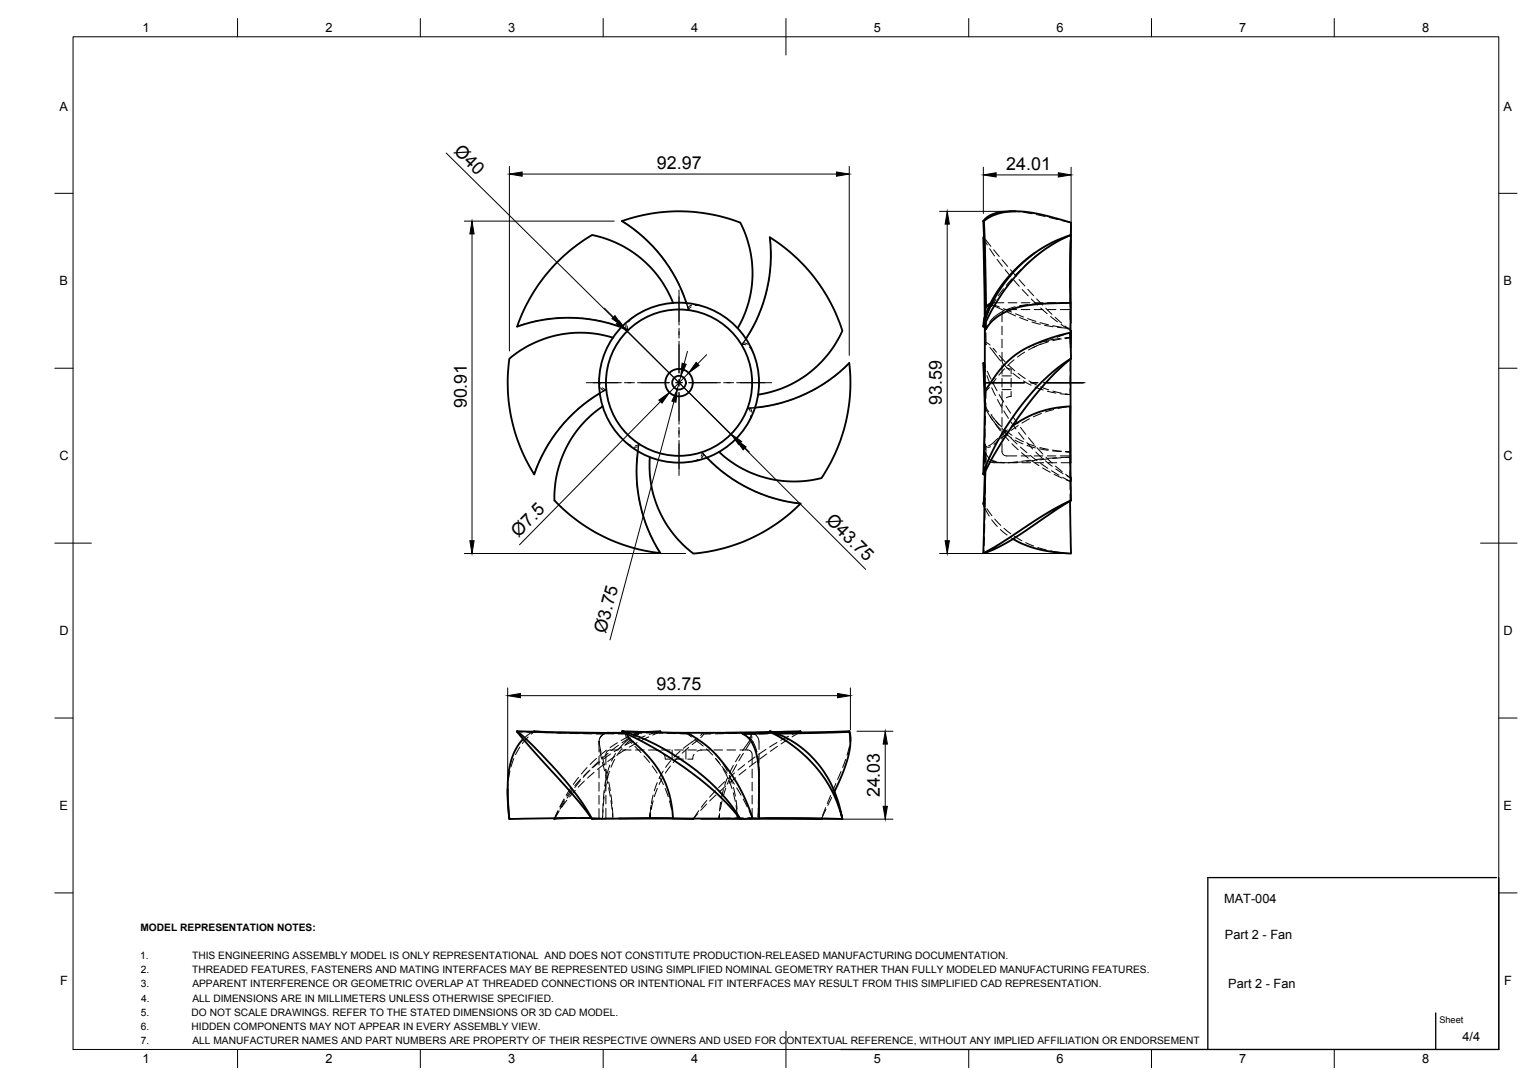
ISO-10303-21;
HEADER;
/* Generated by software containing ST-Developer
 * from STEP Tools, Inc. (www.steptools.com) 
 */

FILE_DESCRIPTION(
/* description */ ('STEP AP214'),
/* implementation_level */ '2;1');

FILE_NAME(
/* name */ 'Part 2 - Fan.step',
/* time_stamp */ '2026-11-14T05:34:33-08:00',
/* author */ (''),
/* organization */ (''),
/* preprocessor_version */ 'ST-DEVELOPER v20.2',
/* originating_system */ 'Autodesk Translation Framework v15.17.0.0',
/* authorisation */ '');

FILE_SCHEMA (('AUTOMOTIVE_DESIGN { 1 0 10303 214 3 1 1 }'));
ENDSEC;

DATA;
#10=MECHANICAL_DESIGN_GEOMETRIC_PRESENTATION_REPRESENTATION('',(#24),#37625);
#20=SHAPE_REPRESENTATION_RELATIONSHIP('SRR','None',#37640,#22);
#22=ADVANCED_BREP_SHAPE_REPRESENTATION('',(#26),#37624);
#24=STYLED_ITEM('',(#37659),#26);
#26=MANIFOLD_SOLID_BREP('Body1',#11498);
#243=B_SPLINE_SURFACE_WITH_KNOTS('',3,3,((#32650,#32651,#32652,#32653,#32654,
#32655,#32656),(#32657,#32658,#32659,#32660,#32661,#32662,#32663),(#32664,
#32665,#32666,#32667,#32668,#32669,#32670),(#32671,#32672,#32673,#32674,
#32675,#32676,#32677),(#32678,#32679,#32680,#32681,#32682,#32683,#32684),
(#32685,#32686,#32687,#32688,#32689,#32690,#32691),(#32692,#32693,#32694,
#32695,#32696,#32697,#32698),(#32699,#32700,#32701,#32702,#32703,#32704,
#32705),(#32706,#32707,#32708,#32709,#32710,#32711,#32712),(#32713,#32714,
#32715,#32716,#32717,#32718,#32719),(#32720,#32721,#32722,#32723,#32724,
#32725,#32726),(#32727,#32728,#32729,#32730,#32731,#32732,#32733),(#32734,
#32735,#32736,#32737,#32738,#32739,#32740)),.UNSPECIFIED.,.F.,.F.,.F.,(4,
3,1,1,1,3,4),(4,3,4),(0.991784279387784,0.992409194183265,0.994306895637448,
0.996204597091632,0.998102298545816,1.,1.0001828629104),(-0.00779503841308724,
0.,0.779503841308724),.UNSPECIFIED.);
#244=B_SPLINE_SURFACE_WITH_KNOTS('',3,3,((#32756,#32757,#32758,#32759,#32760,
#32761,#32762,#32763,#32764,#32765,#32766,#32767,#32768,#32769,#32770,#32771,
#32772),(#32773,#32774,#32775,#32776,#32777,#32778,#32779,#32780,#32781,
#32782,#32783,#32784,#32785,#32786,#32787,#32788,#32789),(#32790,#32791,
#32792,#32793,#32794,#32795,#32796,#32797,#32798,#32799,#32800,#32801,#32802,
#32803,#32804,#32805,#32806),(#32807,#32808,#32809,#32810,#32811,#32812,
#32813,#32814,#32815,#32816,#32817,#32818,#32819,#32820,#32821,#32822,#32823),
(#32824,#32825,#32826,#32827,#32828,#32829,#32830,#32831,#32832,#32833,
#32834,#32835,#32836,#32837,#32838,#32839,#32840),(#32841,#32842,#32843,
#32844,#32845,#32846,#32847,#32848,#32849,#32850,#32851,#32852,#32853,#32854,
#32855,#32856,#32857),(#32858,#32859,#32860,#32861,#32862,#32863,#32864,
#32865,#32866,#32867,#32868,#32869,#32870,#32871,#32872,#32873,#32874),
(#32875,#32876,#32877,#32878,#32879,#32880,#32881,#32882,#32883,#32884,
#32885,#32886,#32887,#32888,#32889,#32890,#32891),(#32892,#32893,#32894,
#32895,#32896,#32897,#32898,#32899,#32900,#32901,#32902,#32903,#32904,#32905,
#32906,#32907,#32908),(#32909,#32910,#32911,#32912,#32913,#32914,#32915,
#32916,#32917,#32918,#32919,#32920,#32921,#32922,#32923,#32924,#32925),
(#32926,#32927,#32928,#32929,#32930,#32931,#32932,#32933,#32934,#32935,
#32936,#32937,#32938,#32939,#32940,#32941,#32942),(#32943,#32944,#32945,
#32946,#32947,#32948,#32949,#32950,#32951,#32952,#32953,#32954,#32955,#32956,
#32957,#32958,#32959),(#32960,#32961,#32962,#32963,#32964,#32965,#32966,
#32967,#32968,#32969,#32970,#32971,#32972,#32973,#32974,#32975,#32976),
(#32977,#32978,#32979,#32980,#32981,#32982,#32983,#32984,#32985,#32986,
#32987,#32988,#32989,#32990,#32991,#32992,#32993),(#32994,#32995,#32996,
#32997,#32998,#32999,#33000,#33001,#33002,#33003,#33004,#33005,#33006,#33007,
#33008,#33009,#33010),(#33011,#33012,#33013,#33014,#33015,#33016,#33017,
#33018,#33019,#33020,#33021,#33022,#33023,#33024,#33025,#33026,#33027)),
 .UNSPECIFIED.,.F.,.F.,.F.,(4,2,1,1,1,1,1,1,1,1,2,4),(4,2,1,1,1,1,1,1,1,
1,1,2,4),(-0.035701835836904,0.,0.090219017653024,0.22554754413256,0.315766561785584,
0.45109508826512,0.541314105918144,0.67664263239768,0.766861650050704,0.90219017653024,
0.992409194183265,1.02810227746674),(-0.0217729438654334,0.,0.0708639855735204,
0.141727971147041,0.212591956720561,0.318887935080842,0.389751920654362,
0.460615906227882,0.566911884588163,0.637775870161683,0.708639855735204,
0.779503841308724,0.801994948010107),.UNSPECIFIED.);
#245=B_SPLINE_SURFACE_WITH_KNOTS('',3,3,((#33062,#33063,#33064,#33065,#33066,
#33067,#33068,#33069,#33070,#33071,#33072,#33073,#33074,#33075,#33076,#33077,
#33078),(#33079,#33080,#33081,#33082,#33083,#33084,#33085,#33086,#33087,
#33088,#33089,#33090,#33091,#33092,#33093,#33094,#33095),(#33096,#33097,
#33098,#33099,#33100,#33101,#33102,#33103,#33104,#33105,#33106,#33107,#33108,
#33109,#33110,#33111,#33112),(#33113,#33114,#33115,#33116,#33117,#33118,
#33119,#33120,#33121,#33122,#33123,#33124,#33125,#33126,#33127,#33128,#33129),
(#33130,#33131,#33132,#33133,#33134,#33135,#33136,#33137,#33138,#33139,
#33140,#33141,#33142,#33143,#33144,#33145,#33146),(#33147,#33148,#33149,
#33150,#33151,#33152,#33153,#33154,#33155,#33156,#33157,#33158,#33159,#33160,
#33161,#33162,#33163),(#33164,#33165,#33166,#33167,#33168,#33169,#33170,
#33171,#33172,#33173,#33174,#33175,#33176,#33177,#33178,#33179,#33180),
(#33181,#33182,#33183,#33184,#33185,#33186,#33187,#33188,#33189,#33190,
#33191,#33192,#33193,#33194,#33195,#33196,#33197),(#33198,#33199,#33200,
#33201,#33202,#33203,#33204,#33205,#33206,#33207,#33208,#33209,#33210,#33211,
#33212,#33213,#33214),(#33215,#33216,#33217,#33218,#33219,#33220,#33221,
#33222,#33223,#33224,#33225,#33226,#33227,#33228,#33229,#33230,#33231),
(#33232,#33233,#33234,#33235,#33236,#33237,#33238,#33239,#33240,#33241,
#33242,#33243,#33244,#33245,#33246,#33247,#33248),(#33249,#33250,#33251,
#33252,#33253,#33254,#33255,#33256,#33257,#33258,#33259,#33260,#33261,#33262,
#33263,#33264,#33265),(#33266,#33267,#33268,#33269,#33270,#33271,#33272,
#33273,#33274,#33275,#33276,#33277,#33278,#33279,#33280,#33281,#33282),
(#33283,#33284,#33285,#33286,#33287,#33288,#33289,#33290,#33291,#33292,
#33293,#33294,#33295,#33296,#33297,#33298,#33299),(#33300,#33301,#33302,
#33303,#33304,#33305,#33306,#33307,#33308,#33309,#33310,#33311,#33312,#33313,
#33314,#33315,#33316),(#33317,#33318,#33319,#33320,#33321,#33322,#33323,
#33324,#33325,#33326,#33327,#33328,#33329,#33330,#33331,#33332,#33333),
(#33334,#33335,#33336,#33337,#33338,#33339,#33340,#33341,#33342,#33343,
#33344,#33345,#33346,#33347,#33348,#33349,#33350)),.UNSPECIFIED.,.F.,.F.,
 .F.,(4,2,1,1,1,1,1,1,1,1,1,2,4),(4,2,1,1,1,1,1,1,1,1,1,2,4),(-0.0353050121574204,
0.,0.0909090909090909,0.181818181818182,0.272727272727273,0.409090909090909,
0.5,0.590909090909091,0.727272727272727,0.818181818181818,0.909090909090909,
1.,1.03479194496591),(-0.021689269548343,0.,0.0708639855735204,0.141727971147041,
0.212591956720561,0.318887935080842,0.389751920654362,0.460615906227882,
0.566911884588163,0.637775870161683,0.708639855735204,0.779503841308724,
0.801875267322681),.UNSPECIFIED.);
#246=B_SPLINE_SURFACE_WITH_KNOTS('',3,3,((#33361,#33362,#33363,#33364,#33365,
#33366,#33367,#33368,#33369,#33370,#33371,#33372,#33373,#33374,#33375,#33376,
#33377),(#33378,#33379,#33380,#33381,#33382,#33383,#33384,#33385,#33386,
#33387,#33388,#33389,#33390,#33391,#33392,#33393,#33394),(#33395,#33396,
#33397,#33398,#33399,#33400,#33401,#33402,#33403,#33404,#33405,#33406,#33407,
#33408,#33409,#33410,#33411),(#33412,#33413,#33414,#33415,#33416,#33417,
#33418,#33419,#33420,#33421,#33422,#33423,#33424,#33425,#33426,#33427,#33428),
(#33429,#33430,#33431,#33432,#33433,#33434,#33435,#33436,#33437,#33438,
#33439,#33440,#33441,#33442,#33443,#33444,#33445),(#33446,#33447,#33448,
#33449,#33450,#33451,#33452,#33453,#33454,#33455,#33456,#33457,#33458,#33459,
#33460,#33461,#33462),(#33463,#33464,#33465,#33466,#33467,#33468,#33469,
#33470,#33471,#33472,#33473,#33474,#33475,#33476,#33477,#33478,#33479),
(#33480,#33481,#33482,#33483,#33484,#33485,#33486,#33487,#33488,#33489,
#33490,#33491,#33492,#33493,#33494,#33495,#33496),(#33497,#33498,#33499,
#33500,#33501,#33502,#33503,#33504,#33505,#33506,#33507,#33508,#33509,#33510,
#33511,#33512,#33513),(#33514,#33515,#33516,#33517,#33518,#33519,#33520,
#33521,#33522,#33523,#33524,#33525,#33526,#33527,#33528,#33529,#33530),
(#33531,#33532,#33533,#33534,#33535,#33536,#33537,#33538,#33539,#33540,
#33541,#33542,#33543,#33544,#33545,#33546,#33547),(#33548,#33549,#33550,
#33551,#33552,#33553,#33554,#33555,#33556,#33557,#33558,#33559,#33560,#33561,
#33562,#33563,#33564),(#33565,#33566,#33567,#33568,#33569,#33570,#33571,
#33572,#33573,#33574,#33575,#33576,#33577,#33578,#33579,#33580,#33581),
(#33582,#33583,#33584,#33585,#33586,#33587,#33588,#33589,#33590,#33591,
#33592,#33593,#33594,#33595,#33596,#33597,#33598),(#33599,#33600,#33601,
#33602,#33603,#33604,#33605,#33606,#33607,#33608,#33609,#33610,#33611,#33612,
#33613,#33614,#33615),(#33616,#33617,#33618,#33619,#33620,#33621,#33622,
#33623,#33624,#33625,#33626,#33627,#33628,#33629,#33630,#33631,#33632),
(#33633,#33634,#33635,#33636,#33637,#33638,#33639,#33640,#33641,#33642,
#33643,#33644,#33645,#33646,#33647,#33648,#33649)),.UNSPECIFIED.,.F.,.F.,
 .F.,(4,2,1,1,1,1,1,1,1,1,1,2,4),(4,2,1,1,1,1,1,1,1,1,1,2,4),(-0.0353050121574204,
0.,0.0909090909090909,0.181818181818182,0.272727272727273,0.409090909090909,
0.5,0.590909090909091,0.727272727272727,0.818181818181818,0.909090909090909,
1.,1.03479194496591),(-0.021689269548343,0.,0.0708639855735204,0.141727971147041,
0.212591956720561,0.318887935080842,0.389751920654362,0.460615906227882,
0.566911884588163,0.637775870161683,0.708639855735204,0.779503841308724,
0.801875267322681),.UNSPECIFIED.);
#247=B_SPLINE_SURFACE_WITH_KNOTS('',3,3,((#33693,#33694,#33695,#33696,#33697,
#33698,#33699,#33700,#33701,#33702,#33703,#33704,#33705,#33706,#33707,#33708,
#33709),(#33710,#33711,#33712,#33713,#33714,#33715,#33716,#33717,#33718,
#33719,#33720,#33721,#33722,#33723,#33724,#33725,#33726),(#33727,#33728,
#33729,#33730,#33731,#33732,#33733,#33734,#33735,#33736,#33737,#33738,#33739,
#33740,#33741,#33742,#33743),(#33744,#33745,#33746,#33747,#33748,#33749,
#33750,#33751,#33752,#33753,#33754,#33755,#33756,#33757,#33758,#33759,#33760),
(#33761,#33762,#33763,#33764,#33765,#33766,#33767,#33768,#33769,#33770,
#33771,#33772,#33773,#33774,#33775,#33776,#33777),(#33778,#33779,#33780,
#33781,#33782,#33783,#33784,#33785,#33786,#33787,#33788,#33789,#33790,#33791,
#33792,#33793,#33794),(#33795,#33796,#33797,#33798,#33799,#33800,#33801,
#33802,#33803,#33804,#33805,#33806,#33807,#33808,#33809,#33810,#33811),
(#33812,#33813,#33814,#33815,#33816,#33817,#33818,#33819,#33820,#33821,
#33822,#33823,#33824,#33825,#33826,#33827,#33828),(#33829,#33830,#33831,
#33832,#33833,#33834,#33835,#33836,#33837,#33838,#33839,#33840,#33841,#33842,
#33843,#33844,#33845),(#33846,#33847,#33848,#33849,#33850,#33851,#33852,
#33853,#33854,#33855,#33856,#33857,#33858,#33859,#33860,#33861,#33862),
(#33863,#33864,#33865,#33866,#33867,#33868,#33869,#33870,#33871,#33872,
#33873,#33874,#33875,#33876,#33877,#33878,#33879),(#33880,#33881,#33882,
#33883,#33884,#33885,#33886,#33887,#33888,#33889,#33890,#33891,#33892,#33893,
#33894,#33895,#33896),(#33897,#33898,#33899,#33900,#33901,#33902,#33903,
#33904,#33905,#33906,#33907,#33908,#33909,#33910,#33911,#33912,#33913),
(#33914,#33915,#33916,#33917,#33918,#33919,#33920,#33921,#33922,#33923,
#33924,#33925,#33926,#33927,#33928,#33929,#33930),(#33931,#33932,#33933,
#33934,#33935,#33936,#33937,#33938,#33939,#33940,#33941,#33942,#33943,#33944,
#33945,#33946,#33947),(#33948,#33949,#33950,#33951,#33952,#33953,#33954,
#33955,#33956,#33957,#33958,#33959,#33960,#33961,#33962,#33963,#33964)),
 .UNSPECIFIED.,.F.,.F.,.F.,(4,2,1,1,1,1,1,1,1,1,2,4),(4,2,1,1,1,1,1,1,1,
1,1,2,4),(-0.035701835836904,0.,0.090219017653024,0.22554754413256,0.315766561785584,
0.45109508826512,0.541314105918144,0.67664263239768,0.766861650050704,0.90219017653024,
0.992409194183265,1.02810227746674),(-0.0217729438654334,0.,0.0708639855735204,
0.141727971147041,0.212591956720561,0.318887935080842,0.389751920654362,
0.460615906227882,0.566911884588163,0.637775870161683,0.708639855735204,
0.779503841308724,0.801994948010107),.UNSPECIFIED.);
#248=B_SPLINE_SURFACE_WITH_KNOTS('',3,3,((#33980,#33981,#33982,#33983,#33984,
#33985,#33986),(#33987,#33988,#33989,#33990,#33991,#33992,#33993),(#33994,
#33995,#33996,#33997,#33998,#33999,#34000),(#34001,#34002,#34003,#34004,
#34005,#34006,#34007),(#34008,#34009,#34010,#34011,#34012,#34013,#34014),
(#34015,#34016,#34017,#34018,#34019,#34020,#34021),(#34022,#34023,#34024,
#34025,#34026,#34027,#34028),(#34029,#34030,#34031,#34032,#34033,#34034,
#34035),(#34036,#34037,#34038,#34039,#34040,#34041,#34042),(#34043,#34044,
#34045,#34046,#34047,#34048,#34049),(#34050,#34051,#34052,#34053,#34054,
#34055,#34056),(#34057,#34058,#34059,#34060,#34061,#34062,#34063),(#34064,
#34065,#34066,#34067,#34068,#34069,#34070)),.UNSPECIFIED.,.F.,.F.,.F.,(4,
3,1,1,1,3,4),(4,3,4),(0.991784279387784,0.992409194183265,0.994306895637448,
0.996204597091632,0.998102298545816,1.,1.0001828629104),(-0.00779503841308724,
0.,0.779503841308724),.UNSPECIFIED.);
#249=B_SPLINE_SURFACE_WITH_KNOTS('',3,3,((#34072,#34073,#34074,#34075,#34076,
#34077,#34078,#34079,#34080,#34081,#34082,#34083,#34084,#34085,#34086,#34087,
#34088),(#34089,#34090,#34091,#34092,#34093,#34094,#34095,#34096,#34097,
#34098,#34099,#34100,#34101,#34102,#34103,#34104,#34105),(#34106,#34107,
#34108,#34109,#34110,#34111,#34112,#34113,#34114,#34115,#34116,#34117,#34118,
#34119,#34120,#34121,#34122),(#34123,#34124,#34125,#34126,#34127,#34128,
#34129,#34130,#34131,#34132,#34133,#34134,#34135,#34136,#34137,#34138,#34139),
(#34140,#34141,#34142,#34143,#34144,#34145,#34146,#34147,#34148,#34149,
#34150,#34151,#34152,#34153,#34154,#34155,#34156),(#34157,#34158,#34159,
#34160,#34161,#34162,#34163,#34164,#34165,#34166,#34167,#34168,#34169,#34170,
#34171,#34172,#34173),(#34174,#34175,#34176,#34177,#34178,#34179,#34180,
#34181,#34182,#34183,#34184,#34185,#34186,#34187,#34188,#34189,#34190),
(#34191,#34192,#34193,#34194,#34195,#34196,#34197,#34198,#34199,#34200,
#34201,#34202,#34203,#34204,#34205,#34206,#34207),(#34208,#34209,#34210,
#34211,#34212,#34213,#34214,#34215,#34216,#34217,#34218,#34219,#34220,#34221,
#34222,#34223,#34224),(#34225,#34226,#34227,#34228,#34229,#34230,#34231,
#34232,#34233,#34234,#34235,#34236,#34237,#34238,#34239,#34240,#34241),
(#34242,#34243,#34244,#34245,#34246,#34247,#34248,#34249,#34250,#34251,
#34252,#34253,#34254,#34255,#34256,#34257,#34258),(#34259,#34260,#34261,
#34262,#34263,#34264,#34265,#34266,#34267,#34268,#34269,#34270,#34271,#34272,
#34273,#34274,#34275),(#34276,#34277,#34278,#34279,#34280,#34281,#34282,
#34283,#34284,#34285,#34286,#34287,#34288,#34289,#34290,#34291,#34292),
(#34293,#34294,#34295,#34296,#34297,#34298,#34299,#34300,#34301,#34302,
#34303,#34304,#34305,#34306,#34307,#34308,#34309),(#34310,#34311,#34312,
#34313,#34314,#34315,#34316,#34317,#34318,#34319,#34320,#34321,#34322,#34323,
#34324,#34325,#34326),(#34327,#34328,#34329,#34330,#34331,#34332,#34333,
#34334,#34335,#34336,#34337,#34338,#34339,#34340,#34341,#34342,#34343),
(#34344,#34345,#34346,#34347,#34348,#34349,#34350,#34351,#34352,#34353,
#34354,#34355,#34356,#34357,#34358,#34359,#34360)),.UNSPECIFIED.,.F.,.F.,
 .F.,(4,2,1,1,1,1,1,1,1,1,1,2,4),(4,2,1,1,1,1,1,1,1,1,1,2,4),(-0.0353050121574204,
0.,0.0909090909090909,0.181818181818182,0.272727272727273,0.409090909090909,
0.5,0.590909090909091,0.727272727272727,0.818181818181818,0.909090909090909,
1.,1.03479194496591),(-0.021689269548343,0.,0.0708639855735204,0.141727971147041,
0.212591956720561,0.318887935080842,0.389751920654362,0.460615906227882,
0.566911884588163,0.637775870161683,0.708639855735204,0.779503841308724,
0.801875267322681),.UNSPECIFIED.);
#250=B_SPLINE_SURFACE_WITH_KNOTS('',3,3,((#34404,#34405,#34406,#34407,#34408,
#34409,#34410,#34411,#34412,#34413,#34414,#34415,#34416,#34417,#34418,#34419,
#34420),(#34421,#34422,#34423,#34424,#34425,#34426,#34427,#34428,#34429,
#34430,#34431,#34432,#34433,#34434,#34435,#34436,#34437),(#34438,#34439,
#34440,#34441,#34442,#34443,#34444,#34445,#34446,#34447,#34448,#34449,#34450,
#34451,#34452,#34453,#34454),(#34455,#34456,#34457,#34458,#34459,#34460,
#34461,#34462,#34463,#34464,#34465,#34466,#34467,#34468,#34469,#34470,#34471),
(#34472,#34473,#34474,#34475,#34476,#34477,#34478,#34479,#34480,#34481,
#34482,#34483,#34484,#34485,#34486,#34487,#34488),(#34489,#34490,#34491,
#34492,#34493,#34494,#34495,#34496,#34497,#34498,#34499,#34500,#34501,#34502,
#34503,#34504,#34505),(#34506,#34507,#34508,#34509,#34510,#34511,#34512,
#34513,#34514,#34515,#34516,#34517,#34518,#34519,#34520,#34521,#34522),
(#34523,#34524,#34525,#34526,#34527,#34528,#34529,#34530,#34531,#34532,
#34533,#34534,#34535,#34536,#34537,#34538,#34539),(#34540,#34541,#34542,
#34543,#34544,#34545,#34546,#34547,#34548,#34549,#34550,#34551,#34552,#34553,
#34554,#34555,#34556),(#34557,#34558,#34559,#34560,#34561,#34562,#34563,
#34564,#34565,#34566,#34567,#34568,#34569,#34570,#34571,#34572,#34573),
(#34574,#34575,#34576,#34577,#34578,#34579,#34580,#34581,#34582,#34583,
#34584,#34585,#34586,#34587,#34588,#34589,#34590),(#34591,#34592,#34593,
#34594,#34595,#34596,#34597,#34598,#34599,#34600,#34601,#34602,#34603,#34604,
#34605,#34606,#34607),(#34608,#34609,#34610,#34611,#34612,#34613,#34614,
#34615,#34616,#34617,#34618,#34619,#34620,#34621,#34622,#34623,#34624),
(#34625,#34626,#34627,#34628,#34629,#34630,#34631,#34632,#34633,#34634,
#34635,#34636,#34637,#34638,#34639,#34640,#34641),(#34642,#34643,#34644,
#34645,#34646,#34647,#34648,#34649,#34650,#34651,#34652,#34653,#34654,#34655,
#34656,#34657,#34658),(#34659,#34660,#34661,#34662,#34663,#34664,#34665,
#34666,#34667,#34668,#34669,#34670,#34671,#34672,#34673,#34674,#34675)),
 .UNSPECIFIED.,.F.,.F.,.F.,(4,2,1,1,1,1,1,1,1,1,2,4),(4,2,1,1,1,1,1,1,1,
1,1,2,4),(-0.035701835836904,0.,0.090219017653024,0.22554754413256,0.315766561785584,
0.45109508826512,0.541314105918144,0.67664263239768,0.766861650050704,0.90219017653024,
0.992409194183265,1.02810227746674),(-0.0217729438654334,0.,0.0708639855735204,
0.141727971147041,0.212591956720561,0.318887935080842,0.389751920654362,
0.460615906227882,0.566911884588163,0.637775870161683,0.708639855735204,
0.779503841308724,0.801994948010107),.UNSPECIFIED.);
#251=B_SPLINE_SURFACE_WITH_KNOTS('',3,3,((#34691,#34692,#34693,#34694,#34695,
#34696,#34697),(#34698,#34699,#34700,#34701,#34702,#34703,#34704),(#34705,
#34706,#34707,#34708,#34709,#34710,#34711),(#34712,#34713,#34714,#34715,
#34716,#34717,#34718),(#34719,#34720,#34721,#34722,#34723,#34724,#34725),
(#34726,#34727,#34728,#34729,#34730,#34731,#34732),(#34733,#34734,#34735,
#34736,#34737,#34738,#34739),(#34740,#34741,#34742,#34743,#34744,#34745,
#34746),(#34747,#34748,#34749,#34750,#34751,#34752,#34753),(#34754,#34755,
#34756,#34757,#34758,#34759,#34760),(#34761,#34762,#34763,#34764,#34765,
#34766,#34767),(#34768,#34769,#34770,#34771,#34772,#34773,#34774),(#34775,
#34776,#34777,#34778,#34779,#34780,#34781)),.UNSPECIFIED.,.F.,.F.,.F.,(4,
3,1,1,1,3,4),(4,3,4),(0.991784279387784,0.992409194183265,0.994306895637448,
0.996204597091632,0.998102298545816,1.,1.0001828629104),(-0.00779503841308724,
0.,0.779503841308724),.UNSPECIFIED.);
#252=B_SPLINE_SURFACE_WITH_KNOTS('',3,3,((#34783,#34784,#34785,#34786,#34787,
#34788,#34789,#34790,#34791,#34792,#34793,#34794,#34795,#34796,#34797,#34798,
#34799),(#34800,#34801,#34802,#34803,#34804,#34805,#34806,#34807,#34808,
#34809,#34810,#34811,#34812,#34813,#34814,#34815,#34816),(#34817,#34818,
#34819,#34820,#34821,#34822,#34823,#34824,#34825,#34826,#34827,#34828,#34829,
#34830,#34831,#34832,#34833),(#34834,#34835,#34836,#34837,#34838,#34839,
#34840,#34841,#34842,#34843,#34844,#34845,#34846,#34847,#34848,#34849,#34850),
(#34851,#34852,#34853,#34854,#34855,#34856,#34857,#34858,#34859,#34860,
#34861,#34862,#34863,#34864,#34865,#34866,#34867),(#34868,#34869,#34870,
#34871,#34872,#34873,#34874,#34875,#34876,#34877,#34878,#34879,#34880,#34881,
#34882,#34883,#34884),(#34885,#34886,#34887,#34888,#34889,#34890,#34891,
#34892,#34893,#34894,#34895,#34896,#34897,#34898,#34899,#34900,#34901),
(#34902,#34903,#34904,#34905,#34906,#34907,#34908,#34909,#34910,#34911,
#34912,#34913,#34914,#34915,#34916,#34917,#34918),(#34919,#34920,#34921,
#34922,#34923,#34924,#34925,#34926,#34927,#34928,#34929,#34930,#34931,#34932,
#34933,#34934,#34935),(#34936,#34937,#34938,#34939,#34940,#34941,#34942,
#34943,#34944,#34945,#34946,#34947,#34948,#34949,#34950,#34951,#34952),
(#34953,#34954,#34955,#34956,#34957,#34958,#34959,#34960,#34961,#34962,
#34963,#34964,#34965,#34966,#34967,#34968,#34969),(#34970,#34971,#34972,
#34973,#34974,#34975,#34976,#34977,#34978,#34979,#34980,#34981,#34982,#34983,
#34984,#34985,#34986),(#34987,#34988,#34989,#34990,#34991,#34992,#34993,
#34994,#34995,#34996,#34997,#34998,#34999,#35000,#35001,#35002,#35003),
(#35004,#35005,#35006,#35007,#35008,#35009,#35010,#35011,#35012,#35013,
#35014,#35015,#35016,#35017,#35018,#35019,#35020),(#35021,#35022,#35023,
#35024,#35025,#35026,#35027,#35028,#35029,#35030,#35031,#35032,#35033,#35034,
#35035,#35036,#35037),(#35038,#35039,#35040,#35041,#35042,#35043,#35044,
#35045,#35046,#35047,#35048,#35049,#35050,#35051,#35052,#35053,#35054),
(#35055,#35056,#35057,#35058,#35059,#35060,#35061,#35062,#35063,#35064,
#35065,#35066,#35067,#35068,#35069,#35070,#35071)),.UNSPECIFIED.,.F.,.F.,
 .F.,(4,2,1,1,1,1,1,1,1,1,1,2,4),(4,2,1,1,1,1,1,1,1,1,1,2,4),(-0.0353050121574204,
0.,0.0909090909090909,0.181818181818182,0.272727272727273,0.409090909090909,
0.5,0.590909090909091,0.727272727272727,0.818181818181818,0.909090909090909,
1.,1.03479194496591),(-0.021689269548343,0.,0.0708639855735204,0.141727971147041,
0.212591956720561,0.318887935080842,0.389751920654362,0.460615906227882,
0.566911884588163,0.637775870161683,0.708639855735204,0.779503841308724,
0.801875267322681),.UNSPECIFIED.);
#253=B_SPLINE_SURFACE_WITH_KNOTS('',3,3,((#35115,#35116,#35117,#35118,#35119,
#35120,#35121,#35122,#35123,#35124,#35125,#35126,#35127,#35128,#35129,#35130,
#35131),(#35132,#35133,#35134,#35135,#35136,#35137,#35138,#35139,#35140,
#35141,#35142,#35143,#35144,#35145,#35146,#35147,#35148),(#35149,#35150,
#35151,#35152,#35153,#35154,#35155,#35156,#35157,#35158,#35159,#35160,#35161,
#35162,#35163,#35164,#35165),(#35166,#35167,#35168,#35169,#35170,#35171,
#35172,#35173,#35174,#35175,#35176,#35177,#35178,#35179,#35180,#35181,#35182),
(#35183,#35184,#35185,#35186,#35187,#35188,#35189,#35190,#35191,#35192,
#35193,#35194,#35195,#35196,#35197,#35198,#35199),(#35200,#35201,#35202,
#35203,#35204,#35205,#35206,#35207,#35208,#35209,#35210,#35211,#35212,#35213,
#35214,#35215,#35216),(#35217,#35218,#35219,#35220,#35221,#35222,#35223,
#35224,#35225,#35226,#35227,#35228,#35229,#35230,#35231,#35232,#35233),
(#35234,#35235,#35236,#35237,#35238,#35239,#35240,#35241,#35242,#35243,
#35244,#35245,#35246,#35247,#35248,#35249,#35250),(#35251,#35252,#35253,
#35254,#35255,#35256,#35257,#35258,#35259,#35260,#35261,#35262,#35263,#35264,
#35265,#35266,#35267),(#35268,#35269,#35270,#35271,#35272,#35273,#35274,
#35275,#35276,#35277,#35278,#35279,#35280,#35281,#35282,#35283,#35284),
(#35285,#35286,#35287,#35288,#35289,#35290,#35291,#35292,#35293,#35294,
#35295,#35296,#35297,#35298,#35299,#35300,#35301),(#35302,#35303,#35304,
#35305,#35306,#35307,#35308,#35309,#35310,#35311,#35312,#35313,#35314,#35315,
#35316,#35317,#35318),(#35319,#35320,#35321,#35322,#35323,#35324,#35325,
#35326,#35327,#35328,#35329,#35330,#35331,#35332,#35333,#35334,#35335),
(#35336,#35337,#35338,#35339,#35340,#35341,#35342,#35343,#35344,#35345,
#35346,#35347,#35348,#35349,#35350,#35351,#35352),(#35353,#35354,#35355,
#35356,#35357,#35358,#35359,#35360,#35361,#35362,#35363,#35364,#35365,#35366,
#35367,#35368,#35369),(#35370,#35371,#35372,#35373,#35374,#35375,#35376,
#35377,#35378,#35379,#35380,#35381,#35382,#35383,#35384,#35385,#35386)),
 .UNSPECIFIED.,.F.,.F.,.F.,(4,2,1,1,1,1,1,1,1,1,2,4),(4,2,1,1,1,1,1,1,1,
1,1,2,4),(-0.035701835836904,0.,0.090219017653024,0.22554754413256,0.315766561785584,
0.45109508826512,0.541314105918144,0.67664263239768,0.766861650050704,0.90219017653024,
0.992409194183265,1.02810227746674),(-0.0217729438654334,0.,0.0708639855735204,
0.141727971147041,0.212591956720561,0.318887935080842,0.389751920654362,
0.460615906227882,0.566911884588163,0.637775870161683,0.708639855735204,
0.779503841308724,0.801994948010107),.UNSPECIFIED.);
#254=B_SPLINE_SURFACE_WITH_KNOTS('',3,3,((#35402,#35403,#35404,#35405,#35406,
#35407,#35408),(#35409,#35410,#35411,#35412,#35413,#35414,#35415),(#35416,
#35417,#35418,#35419,#35420,#35421,#35422),(#35423,#35424,#35425,#35426,
#35427,#35428,#35429),(#35430,#35431,#35432,#35433,#35434,#35435,#35436),
(#35437,#35438,#35439,#35440,#35441,#35442,#35443),(#35444,#35445,#35446,
#35447,#35448,#35449,#35450),(#35451,#35452,#35453,#35454,#35455,#35456,
#35457),(#35458,#35459,#35460,#35461,#35462,#35463,#35464),(#35465,#35466,
#35467,#35468,#35469,#35470,#35471),(#35472,#35473,#35474,#35475,#35476,
#35477,#35478),(#35479,#35480,#35481,#35482,#35483,#35484,#35485),(#35486,
#35487,#35488,#35489,#35490,#35491,#35492)),.UNSPECIFIED.,.F.,.F.,.F.,(4,
3,1,1,1,3,4),(4,3,4),(0.991784279387784,0.992409194183265,0.994306895637448,
0.996204597091632,0.998102298545816,1.,1.0001828629104),(-0.00779503841308724,
0.,0.779503841308724),.UNSPECIFIED.);
#255=B_SPLINE_SURFACE_WITH_KNOTS('',3,3,((#35494,#35495,#35496,#35497,#35498,
#35499,#35500,#35501,#35502,#35503,#35504,#35505,#35506,#35507,#35508,#35509,
#35510),(#35511,#35512,#35513,#35514,#35515,#35516,#35517,#35518,#35519,
#35520,#35521,#35522,#35523,#35524,#35525,#35526,#35527),(#35528,#35529,
#35530,#35531,#35532,#35533,#35534,#35535,#35536,#35537,#35538,#35539,#35540,
#35541,#35542,#35543,#35544),(#35545,#35546,#35547,#35548,#35549,#35550,
#35551,#35552,#35553,#35554,#35555,#35556,#35557,#35558,#35559,#35560,#35561),
(#35562,#35563,#35564,#35565,#35566,#35567,#35568,#35569,#35570,#35571,
#35572,#35573,#35574,#35575,#35576,#35577,#35578),(#35579,#35580,#35581,
#35582,#35583,#35584,#35585,#35586,#35587,#35588,#35589,#35590,#35591,#35592,
#35593,#35594,#35595),(#35596,#35597,#35598,#35599,#35600,#35601,#35602,
#35603,#35604,#35605,#35606,#35607,#35608,#35609,#35610,#35611,#35612),
(#35613,#35614,#35615,#35616,#35617,#35618,#35619,#35620,#35621,#35622,
#35623,#35624,#35625,#35626,#35627,#35628,#35629),(#35630,#35631,#35632,
#35633,#35634,#35635,#35636,#35637,#35638,#35639,#35640,#35641,#35642,#35643,
#35644,#35645,#35646),(#35647,#35648,#35649,#35650,#35651,#35652,#35653,
#35654,#35655,#35656,#35657,#35658,#35659,#35660,#35661,#35662,#35663),
(#35664,#35665,#35666,#35667,#35668,#35669,#35670,#35671,#35672,#35673,
#35674,#35675,#35676,#35677,#35678,#35679,#35680),(#35681,#35682,#35683,
#35684,#35685,#35686,#35687,#35688,#35689,#35690,#35691,#35692,#35693,#35694,
#35695,#35696,#35697),(#35698,#35699,#35700,#35701,#35702,#35703,#35704,
#35705,#35706,#35707,#35708,#35709,#35710,#35711,#35712,#35713,#35714),
(#35715,#35716,#35717,#35718,#35719,#35720,#35721,#35722,#35723,#35724,
#35725,#35726,#35727,#35728,#35729,#35730,#35731),(#35732,#35733,#35734,
#35735,#35736,#35737,#35738,#35739,#35740,#35741,#35742,#35743,#35744,#35745,
#35746,#35747,#35748),(#35749,#35750,#35751,#35752,#35753,#35754,#35755,
#35756,#35757,#35758,#35759,#35760,#35761,#35762,#35763,#35764,#35765),
(#35766,#35767,#35768,#35769,#35770,#35771,#35772,#35773,#35774,#35775,
#35776,#35777,#35778,#35779,#35780,#35781,#35782)),.UNSPECIFIED.,.F.,.F.,
 .F.,(4,2,1,1,1,1,1,1,1,1,1,2,4),(4,2,1,1,1,1,1,1,1,1,1,2,4),(-0.0353050121574204,
0.,0.0909090909090909,0.181818181818182,0.272727272727273,0.409090909090909,
0.5,0.590909090909091,0.727272727272727,0.818181818181818,0.909090909090909,
1.,1.03479194496591),(-0.021689269548343,0.,0.0708639855735204,0.141727971147041,
0.212591956720561,0.318887935080842,0.389751920654362,0.460615906227882,
0.566911884588163,0.637775870161683,0.708639855735204,0.779503841308724,
0.801875267322681),.UNSPECIFIED.);
#256=B_SPLINE_SURFACE_WITH_KNOTS('',3,3,((#35814,#35815,#35816,#35817,#35818,
#35819,#35820,#35821,#35822,#35823,#35824,#35825,#35826,#35827,#35828,#35829,
#35830),(#35831,#35832,#35833,#35834,#35835,#35836,#35837,#35838,#35839,
#35840,#35841,#35842,#35843,#35844,#35845,#35846,#35847),(#35848,#35849,
#35850,#35851,#35852,#35853,#35854,#35855,#35856,#35857,#35858,#35859,#35860,
#35861,#35862,#35863,#35864),(#35865,#35866,#35867,#35868,#35869,#35870,
#35871,#35872,#35873,#35874,#35875,#35876,#35877,#35878,#35879,#35880,#35881),
(#35882,#35883,#35884,#35885,#35886,#35887,#35888,#35889,#35890,#35891,
#35892,#35893,#35894,#35895,#35896,#35897,#35898),(#35899,#35900,#35901,
#35902,#35903,#35904,#35905,#35906,#35907,#35908,#35909,#35910,#35911,#35912,
#35913,#35914,#35915),(#35916,#35917,#35918,#35919,#35920,#35921,#35922,
#35923,#35924,#35925,#35926,#35927,#35928,#35929,#35930,#35931,#35932),
(#35933,#35934,#35935,#35936,#35937,#35938,#35939,#35940,#35941,#35942,
#35943,#35944,#35945,#35946,#35947,#35948,#35949),(#35950,#35951,#35952,
#35953,#35954,#35955,#35956,#35957,#35958,#35959,#35960,#35961,#35962,#35963,
#35964,#35965,#35966),(#35967,#35968,#35969,#35970,#35971,#35972,#35973,
#35974,#35975,#35976,#35977,#35978,#35979,#35980,#35981,#35982,#35983),
(#35984,#35985,#35986,#35987,#35988,#35989,#35990,#35991,#35992,#35993,
#35994,#35995,#35996,#35997,#35998,#35999,#36000),(#36001,#36002,#36003,
#36004,#36005,#36006,#36007,#36008,#36009,#36010,#36011,#36012,#36013,#36014,
#36015,#36016,#36017),(#36018,#36019,#36020,#36021,#36022,#36023,#36024,
#36025,#36026,#36027,#36028,#36029,#36030,#36031,#36032,#36033,#36034),
(#36035,#36036,#36037,#36038,#36039,#36040,#36041,#36042,#36043,#36044,
#36045,#36046,#36047,#36048,#36049,#36050,#36051),(#36052,#36053,#36054,
#36055,#36056,#36057,#36058,#36059,#36060,#36061,#36062,#36063,#36064,#36065,
#36066,#36067,#36068),(#36069,#36070,#36071,#36072,#36073,#36074,#36075,
#36076,#36077,#36078,#36079,#36080,#36081,#36082,#36083,#36084,#36085)),
 .UNSPECIFIED.,.F.,.F.,.F.,(4,2,1,1,1,1,1,1,1,1,2,4),(4,2,1,1,1,1,1,1,1,
1,1,2,4),(-0.035701835836904,0.,0.090219017653024,0.22554754413256,0.315766561785584,
0.45109508826512,0.541314105918144,0.67664263239768,0.766861650050704,0.90219017653024,
0.992409194183265,1.02810227746674),(-0.0217729438654334,0.,0.0708639855735204,
0.141727971147041,0.212591956720561,0.318887935080842,0.389751920654362,
0.460615906227882,0.566911884588163,0.637775870161683,0.708639855735204,
0.779503841308724,0.801994948010107),.UNSPECIFIED.);
#257=B_SPLINE_SURFACE_WITH_KNOTS('',3,3,((#36092,#36093,#36094,#36095,#36096,
#36097,#36098),(#36099,#36100,#36101,#36102,#36103,#36104,#36105),(#36106,
#36107,#36108,#36109,#36110,#36111,#36112),(#36113,#36114,#36115,#36116,
#36117,#36118,#36119),(#36120,#36121,#36122,#36123,#36124,#36125,#36126),
(#36127,#36128,#36129,#36130,#36131,#36132,#36133),(#36134,#36135,#36136,
#36137,#36138,#36139,#36140),(#36141,#36142,#36143,#36144,#36145,#36146,
#36147),(#36148,#36149,#36150,#36151,#36152,#36153,#36154),(#36155,#36156,
#36157,#36158,#36159,#36160,#36161),(#36162,#36163,#36164,#36165,#36166,
#36167,#36168),(#36169,#36170,#36171,#36172,#36173,#36174,#36175),(#36176,
#36177,#36178,#36179,#36180,#36181,#36182)),.UNSPECIFIED.,.F.,.F.,.F.,(4,
3,1,1,1,3,4),(4,3,4),(0.991784279387784,0.992409194183265,0.994306895637448,
0.996204597091632,0.998102298545816,1.,1.0001828629104),(-0.00779503841308724,
0.,0.779503841308724),.UNSPECIFIED.);
#258=B_SPLINE_SURFACE_WITH_KNOTS('',3,3,((#36183,#36184,#36185,#36186,#36187,
#36188,#36189,#36190,#36191,#36192,#36193,#36194,#36195,#36196,#36197,#36198,
#36199),(#36200,#36201,#36202,#36203,#36204,#36205,#36206,#36207,#36208,
#36209,#36210,#36211,#36212,#36213,#36214,#36215,#36216),(#36217,#36218,
#36219,#36220,#36221,#36222,#36223,#36224,#36225,#36226,#36227,#36228,#36229,
#36230,#36231,#36232,#36233),(#36234,#36235,#36236,#36237,#36238,#36239,
#36240,#36241,#36242,#36243,#36244,#36245,#36246,#36247,#36248,#36249,#36250),
(#36251,#36252,#36253,#36254,#36255,#36256,#36257,#36258,#36259,#36260,
#36261,#36262,#36263,#36264,#36265,#36266,#36267),(#36268,#36269,#36270,
#36271,#36272,#36273,#36274,#36275,#36276,#36277,#36278,#36279,#36280,#36281,
#36282,#36283,#36284),(#36285,#36286,#36287,#36288,#36289,#36290,#36291,
#36292,#36293,#36294,#36295,#36296,#36297,#36298,#36299,#36300,#36301),
(#36302,#36303,#36304,#36305,#36306,#36307,#36308,#36309,#36310,#36311,
#36312,#36313,#36314,#36315,#36316,#36317,#36318),(#36319,#36320,#36321,
#36322,#36323,#36324,#36325,#36326,#36327,#36328,#36329,#36330,#36331,#36332,
#36333,#36334,#36335),(#36336,#36337,#36338,#36339,#36340,#36341,#36342,
#36343,#36344,#36345,#36346,#36347,#36348,#36349,#36350,#36351,#36352),
(#36353,#36354,#36355,#36356,#36357,#36358,#36359,#36360,#36361,#36362,
#36363,#36364,#36365,#36366,#36367,#36368,#36369),(#36370,#36371,#36372,
#36373,#36374,#36375,#36376,#36377,#36378,#36379,#36380,#36381,#36382,#36383,
#36384,#36385,#36386),(#36387,#36388,#36389,#36390,#36391,#36392,#36393,
#36394,#36395,#36396,#36397,#36398,#36399,#36400,#36401,#36402,#36403),
(#36404,#36405,#36406,#36407,#36408,#36409,#36410,#36411,#36412,#36413,
#36414,#36415,#36416,#36417,#36418,#36419,#36420),(#36421,#36422,#36423,
#36424,#36425,#36426,#36427,#36428,#36429,#36430,#36431,#36432,#36433,#36434,
#36435,#36436,#36437),(#36438,#36439,#36440,#36441,#36442,#36443,#36444,
#36445,#36446,#36447,#36448,#36449,#36450,#36451,#36452,#36453,#36454),
(#36455,#36456,#36457,#36458,#36459,#36460,#36461,#36462,#36463,#36464,
#36465,#36466,#36467,#36468,#36469,#36470,#36471)),.UNSPECIFIED.,.F.,.F.,
 .F.,(4,2,1,1,1,1,1,1,1,1,1,2,4),(4,2,1,1,1,1,1,1,1,1,1,2,4),(-0.0353050121574204,
0.,0.0909090909090909,0.181818181818182,0.272727272727273,0.409090909090909,
0.5,0.590909090909091,0.727272727272727,0.818181818181818,0.909090909090909,
1.,1.03479194496591),(-0.021689269548343,0.,0.0708639855735204,0.141727971147041,
0.212591956720561,0.318887935080842,0.389751920654362,0.460615906227882,
0.566911884588163,0.637775870161683,0.708639855735204,0.779503841308724,
0.801875267322681),.UNSPECIFIED.);
#259=B_SPLINE_SURFACE_WITH_KNOTS('',3,3,((#36515,#36516,#36517,#36518,#36519,
#36520,#36521,#36522,#36523,#36524,#36525,#36526,#36527,#36528,#36529,#36530,
#36531),(#36532,#36533,#36534,#36535,#36536,#36537,#36538,#36539,#36540,
#36541,#36542,#36543,#36544,#36545,#36546,#36547,#36548),(#36549,#36550,
#36551,#36552,#36553,#36554,#36555,#36556,#36557,#36558,#36559,#36560,#36561,
#36562,#36563,#36564,#36565),(#36566,#36567,#36568,#36569,#36570,#36571,
#36572,#36573,#36574,#36575,#36576,#36577,#36578,#36579,#36580,#36581,#36582),
(#36583,#36584,#36585,#36586,#36587,#36588,#36589,#36590,#36591,#36592,
#36593,#36594,#36595,#36596,#36597,#36598,#36599),(#36600,#36601,#36602,
#36603,#36604,#36605,#36606,#36607,#36608,#36609,#36610,#36611,#36612,#36613,
#36614,#36615,#36616),(#36617,#36618,#36619,#36620,#36621,#36622,#36623,
#36624,#36625,#36626,#36627,#36628,#36629,#36630,#36631,#36632,#36633),
(#36634,#36635,#36636,#36637,#36638,#36639,#36640,#36641,#36642,#36643,
#36644,#36645,#36646,#36647,#36648,#36649,#36650),(#36651,#36652,#36653,
#36654,#36655,#36656,#36657,#36658,#36659,#36660,#36661,#36662,#36663,#36664,
#36665,#36666,#36667),(#36668,#36669,#36670,#36671,#36672,#36673,#36674,
#36675,#36676,#36677,#36678,#36679,#36680,#36681,#36682,#36683,#36684),
(#36685,#36686,#36687,#36688,#36689,#36690,#36691,#36692,#36693,#36694,
#36695,#36696,#36697,#36698,#36699,#36700,#36701),(#36702,#36703,#36704,
#36705,#36706,#36707,#36708,#36709,#36710,#36711,#36712,#36713,#36714,#36715,
#36716,#36717,#36718),(#36719,#36720,#36721,#36722,#36723,#36724,#36725,
#36726,#36727,#36728,#36729,#36730,#36731,#36732,#36733,#36734,#36735),
(#36736,#36737,#36738,#36739,#36740,#36741,#36742,#36743,#36744,#36745,
#36746,#36747,#36748,#36749,#36750,#36751,#36752),(#36753,#36754,#36755,
#36756,#36757,#36758,#36759,#36760,#36761,#36762,#36763,#36764,#36765,#36766,
#36767,#36768,#36769),(#36770,#36771,#36772,#36773,#36774,#36775,#36776,
#36777,#36778,#36779,#36780,#36781,#36782,#36783,#36784,#36785,#36786)),
 .UNSPECIFIED.,.F.,.F.,.F.,(4,2,1,1,1,1,1,1,1,1,2,4),(4,2,1,1,1,1,1,1,1,
1,1,2,4),(-0.035701835836904,0.,0.090219017653024,0.22554754413256,0.315766561785584,
0.45109508826512,0.541314105918144,0.67664263239768,0.766861650050704,0.90219017653024,
0.992409194183265,1.02810227746674),(-0.0217729438654334,0.,0.0708639855735204,
0.141727971147041,0.212591956720561,0.318887935080842,0.389751920654362,
0.460615906227882,0.566911884588163,0.637775870161683,0.708639855735204,
0.779503841308724,0.801994948010107),.UNSPECIFIED.);
#260=B_SPLINE_SURFACE_WITH_KNOTS('',3,3,((#36802,#36803,#36804,#36805,#36806,
#36807,#36808),(#36809,#36810,#36811,#36812,#36813,#36814,#36815),(#36816,
#36817,#36818,#36819,#36820,#36821,#36822),(#36823,#36824,#36825,#36826,
#36827,#36828,#36829),(#36830,#36831,#36832,#36833,#36834,#36835,#36836),
(#36837,#36838,#36839,#36840,#36841,#36842,#36843),(#36844,#36845,#36846,
#36847,#36848,#36849,#36850),(#36851,#36852,#36853,#36854,#36855,#36856,
#36857),(#36858,#36859,#36860,#36861,#36862,#36863,#36864),(#36865,#36866,
#36867,#36868,#36869,#36870,#36871),(#36872,#36873,#36874,#36875,#36876,
#36877,#36878),(#36879,#36880,#36881,#36882,#36883,#36884,#36885),(#36886,
#36887,#36888,#36889,#36890,#36891,#36892)),.UNSPECIFIED.,.F.,.F.,.F.,(4,
3,1,1,1,3,4),(4,3,4),(0.991784279387784,0.992409194183265,0.994306895637448,
0.996204597091632,0.998102298545816,1.,1.0001828629104),(-0.00779503841308724,
0.,0.779503841308724),.UNSPECIFIED.);
#261=B_SPLINE_SURFACE_WITH_KNOTS('',3,3,((#36894,#36895,#36896,#36897,#36898,
#36899,#36900,#36901,#36902,#36903,#36904,#36905,#36906,#36907,#36908,#36909,
#36910),(#36911,#36912,#36913,#36914,#36915,#36916,#36917,#36918,#36919,
#36920,#36921,#36922,#36923,#36924,#36925,#36926,#36927),(#36928,#36929,
#36930,#36931,#36932,#36933,#36934,#36935,#36936,#36937,#36938,#36939,#36940,
#36941,#36942,#36943,#36944),(#36945,#36946,#36947,#36948,#36949,#36950,
#36951,#36952,#36953,#36954,#36955,#36956,#36957,#36958,#36959,#36960,#36961),
(#36962,#36963,#36964,#36965,#36966,#36967,#36968,#36969,#36970,#36971,
#36972,#36973,#36974,#36975,#36976,#36977,#36978),(#36979,#36980,#36981,
#36982,#36983,#36984,#36985,#36986,#36987,#36988,#36989,#36990,#36991,#36992,
#36993,#36994,#36995),(#36996,#36997,#36998,#36999,#37000,#37001,#37002,
#37003,#37004,#37005,#37006,#37007,#37008,#37009,#37010,#37011,#37012),
(#37013,#37014,#37015,#37016,#37017,#37018,#37019,#37020,#37021,#37022,
#37023,#37024,#37025,#37026,#37027,#37028,#37029),(#37030,#37031,#37032,
#37033,#37034,#37035,#37036,#37037,#37038,#37039,#37040,#37041,#37042,#37043,
#37044,#37045,#37046),(#37047,#37048,#37049,#37050,#37051,#37052,#37053,
#37054,#37055,#37056,#37057,#37058,#37059,#37060,#37061,#37062,#37063),
(#37064,#37065,#37066,#37067,#37068,#37069,#37070,#37071,#37072,#37073,
#37074,#37075,#37076,#37077,#37078,#37079,#37080),(#37081,#37082,#37083,
#37084,#37085,#37086,#37087,#37088,#37089,#37090,#37091,#37092,#37093,#37094,
#37095,#37096,#37097),(#37098,#37099,#37100,#37101,#37102,#37103,#37104,
#37105,#37106,#37107,#37108,#37109,#37110,#37111,#37112,#37113,#37114),
(#37115,#37116,#37117,#37118,#37119,#37120,#37121,#37122,#37123,#37124,
#37125,#37126,#37127,#37128,#37129,#37130,#37131),(#37132,#37133,#37134,
#37135,#37136,#37137,#37138,#37139,#37140,#37141,#37142,#37143,#37144,#37145,
#37146,#37147,#37148),(#37149,#37150,#37151,#37152,#37153,#37154,#37155,
#37156,#37157,#37158,#37159,#37160,#37161,#37162,#37163,#37164,#37165),
(#37166,#37167,#37168,#37169,#37170,#37171,#37172,#37173,#37174,#37175,
#37176,#37177,#37178,#37179,#37180,#37181,#37182)),.UNSPECIFIED.,.F.,.F.,
 .F.,(4,2,1,1,1,1,1,1,1,1,1,2,4),(4,2,1,1,1,1,1,1,1,1,1,2,4),(-0.0353050121574204,
0.,0.0909090909090909,0.181818181818182,0.272727272727273,0.409090909090909,
0.5,0.590909090909091,0.727272727272727,0.818181818181818,0.909090909090909,
1.,1.03479194496591),(-0.021689269548343,0.,0.0708639855735204,0.141727971147041,
0.212591956720561,0.318887935080842,0.389751920654362,0.460615906227882,
0.566911884588163,0.637775870161683,0.708639855735204,0.779503841308724,
0.801875267322681),.UNSPECIFIED.);
#262=B_SPLINE_SURFACE_WITH_KNOTS('',3,3,((#37226,#37227,#37228,#37229,#37230,
#37231,#37232,#37233,#37234,#37235,#37236,#37237,#37238,#37239,#37240,#37241,
#37242),(#37243,#37244,#37245,#37246,#37247,#37248,#37249,#37250,#37251,
#37252,#37253,#37254,#37255,#37256,#37257,#37258,#37259),(#37260,#37261,
#37262,#37263,#37264,#37265,#37266,#37267,#37268,#37269,#37270,#37271,#37272,
#37273,#37274,#37275,#37276),(#37277,#37278,#37279,#37280,#37281,#37282,
#37283,#37284,#37285,#37286,#37287,#37288,#37289,#37290,#37291,#37292,#37293),
(#37294,#37295,#37296,#37297,#37298,#37299,#37300,#37301,#37302,#37303,
#37304,#37305,#37306,#37307,#37308,#37309,#37310),(#37311,#37312,#37313,
#37314,#37315,#37316,#37317,#37318,#37319,#37320,#37321,#37322,#37323,#37324,
#37325,#37326,#37327),(#37328,#37329,#37330,#37331,#37332,#37333,#37334,
#37335,#37336,#37337,#37338,#37339,#37340,#37341,#37342,#37343,#37344),
(#37345,#37346,#37347,#37348,#37349,#37350,#37351,#37352,#37353,#37354,
#37355,#37356,#37357,#37358,#37359,#37360,#37361),(#37362,#37363,#37364,
#37365,#37366,#37367,#37368,#37369,#37370,#37371,#37372,#37373,#37374,#37375,
#37376,#37377,#37378),(#37379,#37380,#37381,#37382,#37383,#37384,#37385,
#37386,#37387,#37388,#37389,#37390,#37391,#37392,#37393,#37394,#37395),
(#37396,#37397,#37398,#37399,#37400,#37401,#37402,#37403,#37404,#37405,
#37406,#37407,#37408,#37409,#37410,#37411,#37412),(#37413,#37414,#37415,
#37416,#37417,#37418,#37419,#37420,#37421,#37422,#37423,#37424,#37425,#37426,
#37427,#37428,#37429),(#37430,#37431,#37432,#37433,#37434,#37435,#37436,
#37437,#37438,#37439,#37440,#37441,#37442,#37443,#37444,#37445,#37446),
(#37447,#37448,#37449,#37450,#37451,#37452,#37453,#37454,#37455,#37456,
#37457,#37458,#37459,#37460,#37461,#37462,#37463),(#37464,#37465,#37466,
#37467,#37468,#37469,#37470,#37471,#37472,#37473,#37474,#37475,#37476,#37477,
#37478,#37479,#37480),(#37481,#37482,#37483,#37484,#37485,#37486,#37487,
#37488,#37489,#37490,#37491,#37492,#37493,#37494,#37495,#37496,#37497)),
 .UNSPECIFIED.,.F.,.F.,.F.,(4,2,1,1,1,1,1,1,1,1,2,4),(4,2,1,1,1,1,1,1,1,
1,1,2,4),(-0.035701835836904,0.,0.090219017653024,0.22554754413256,0.315766561785584,
0.45109508826512,0.541314105918144,0.67664263239768,0.766861650050704,0.90219017653024,
0.992409194183265,1.02810227746674),(-0.0217729438654334,0.,0.0708639855735204,
0.141727971147041,0.212591956720561,0.318887935080842,0.389751920654362,
0.460615906227882,0.566911884588163,0.637775870161683,0.708639855735204,
0.779503841308724,0.801994948010107),.UNSPECIFIED.);
#263=B_SPLINE_SURFACE_WITH_KNOTS('',3,3,((#37513,#37514,#37515,#37516,#37517,
#37518,#37519),(#37520,#37521,#37522,#37523,#37524,#37525,#37526),(#37527,
#37528,#37529,#37530,#37531,#37532,#37533),(#37534,#37535,#37536,#37537,
#37538,#37539,#37540),(#37541,#37542,#37543,#37544,#37545,#37546,#37547),
(#37548,#37549,#37550,#37551,#37552,#37553,#37554),(#37555,#37556,#37557,
#37558,#37559,#37560,#37561),(#37562,#37563,#37564,#37565,#37566,#37567,
#37568),(#37569,#37570,#37571,#37572,#37573,#37574,#37575),(#37576,#37577,
#37578,#37579,#37580,#37581,#37582),(#37583,#37584,#37585,#37586,#37587,
#37588,#37589),(#37590,#37591,#37592,#37593,#37594,#37595,#37596),(#37597,
#37598,#37599,#37600,#37601,#37602,#37603)),.UNSPECIFIED.,.F.,.F.,.F.,(4,
3,1,1,1,3,4),(4,3,4),(0.991784279387784,0.992409194183265,0.994306895637448,
0.996204597091632,0.998102298545816,1.,1.0001828629104),(-0.00779503841308724,
0.,0.779503841308724),.UNSPECIFIED.);
#312=FACE_BOUND('',#2525,.T.);
#313=FACE_BOUND('',#2533,.T.);
#314=FACE_BOUND('',#2535,.T.);
#414=PLANE('',#12980);
#415=PLANE('',#12981);
#416=PLANE('',#12988);
#417=PLANE('',#12989);
#418=PLANE('',#12990);
#745=B_SPLINE_CURVE_WITH_KNOTS('',3,(#32202,#32203,#32204,#32205,#32206,
#32207,#32208,#32209,#32210,#32211),.UNSPECIFIED.,.F.,.F.,(4,2,2,2,4),(0.276263636539841,
0.629117133783239,1.26931031034628,1.89807374671191,2.54124258875015),
 .UNSPECIFIED.);
#746=B_SPLINE_CURVE_WITH_KNOTS('',3,(#32215,#32216,#32217,#32218,#32219,
#32220,#32221,#32222,#32223,#32224),.UNSPECIFIED.,.F.,.F.,(4,2,2,2,4),(1.00000001210554E-6,
0.634808922936136,1.24939733333229,1.87099835051043,2.49652016978958),
 .UNSPECIFIED.);
#747=B_SPLINE_CURVE_WITH_KNOTS('',3,(#32226,#32227,#32228,#32229,#32230,
#32231,#32232,#32233,#32234,#32235),.UNSPECIFIED.,.F.,.F.,(4,2,2,2,4),(9.90463797838316E-7,
0.628842488476587,1.26874459572359,1.89778547935364,2.54125154834499),
 .UNSPECIFIED.);
#748=B_SPLINE_CURVE_WITH_KNOTS('',3,(#32239,#32240,#32241,#32242,#32243,
#32244,#32245,#32246,#32247,#32248),.UNSPECIFIED.,.F.,.F.,(4,2,2,2,4),(1.00000001226936E-6,
0.634808922936138,1.24939733333229,1.87099835051041,2.49652016978955),
 .UNSPECIFIED.);
#749=B_SPLINE_CURVE_WITH_KNOTS('',3,(#32250,#32251,#32252,#32253,#32254,
#32255,#32256,#32257,#32258,#32259),.UNSPECIFIED.,.F.,.F.,(4,2,2,2,4),(9.90463797798848E-7,
0.62884248847666,1.26874459572371,1.8977854793538,2.54125154834516),
 .UNSPECIFIED.);
#750=B_SPLINE_CURVE_WITH_KNOTS('',3,(#32265,#32266,#32267,#32268,#32269,
#32270,#32271,#32272,#32273,#32274),.UNSPECIFIED.,.F.,.F.,(4,2,2,2,4),(1.00000001376695E-6,
0.680457901220549,1.33757522030194,1.9141295972232,2.49600347486028),
 .UNSPECIFIED.);
#751=B_SPLINE_CURVE_WITH_KNOTS('',3,(#32276,#32277,#32278,#32279,#32280,
#32281,#32282,#32283,#32284,#32285),.UNSPECIFIED.,.F.,.F.,(4,2,2,2,4),(-2.54325661086045,
-1.81843643838175,-1.11345157109682,-0.553213495814432,-1.00000000724521E-6),
 .UNSPECIFIED.);
#752=B_SPLINE_CURVE_WITH_KNOTS('',3,(#32289,#32290,#32291,#32292,#32293,
#32294,#32295,#32296,#32297,#32298),.UNSPECIFIED.,.F.,.F.,(4,2,2,2,4),(1.00000001195455E-6,
0.634808922936142,1.24939733333231,1.87099835051046,2.49652016978959),
 .UNSPECIFIED.);
#753=B_SPLINE_CURVE_WITH_KNOTS('',3,(#32300,#32301,#32302,#32303,#32304,
#32305,#32306,#32307,#32308,#32309),.UNSPECIFIED.,.F.,.F.,(4,2,2,2,4),(9.90463797727588E-7,
0.628842488476649,1.26874459572375,1.89778547935391,2.54125154834539),
 .UNSPECIFIED.);
#754=B_SPLINE_CURVE_WITH_KNOTS('',3,(#32313,#32314,#32315,#32316,#32317,
#32318,#32319,#32320,#32321,#32322),.UNSPECIFIED.,.F.,.F.,(4,2,2,2,4),(1.00000001181796E-6,
0.634808922936134,1.24939733333227,1.87099835051039,2.4965201697895),
 .UNSPECIFIED.);
#755=B_SPLINE_CURVE_WITH_KNOTS('',3,(#32324,#32325,#32326,#32327,#32328,
#32329,#32330,#32331,#32332,#32333),.UNSPECIFIED.,.F.,.F.,(4,2,2,2,4),(9.90463798206886E-7,
0.6288424884766,1.26874459572362,1.89778547935369,2.54125154834506),
 .UNSPECIFIED.);
#756=B_SPLINE_CURVE_WITH_KNOTS('',3,(#32337,#32338,#32339,#32340,#32341,
#32342,#32343,#32344,#32345,#32346),.UNSPECIFIED.,.F.,.F.,(4,2,2,2,4),(1.00000001290734E-6,
0.634808922936141,1.24939733333231,1.87099835051047,2.49652016978959),
 .UNSPECIFIED.);
#757=B_SPLINE_CURVE_WITH_KNOTS('',3,(#32348,#32349,#32350,#32351,#32352,
#32353,#32354,#32355,#32356,#32357),.UNSPECIFIED.,.F.,.F.,(4,2,2,2,4),(9.9046379766505E-7,
0.628842488476696,1.26874459572384,1.89778547935403,2.54125154834553),
 .UNSPECIFIED.);
#758=B_SPLINE_CURVE_WITH_KNOTS('',3,(#32363,#32364,#32365,#32366),
 .UNSPECIFIED.,.F.,.F.,(4,4),(2.08467470935283,2.49651756792621),
 .UNSPECIFIED.);
#759=B_SPLINE_CURVE_WITH_KNOTS('',3,(#32367,#32368,#32369,#32370),
 .UNSPECIFIED.,.F.,.F.,(4,4),(9.99129608606638E-7,0.276263636539841),
 .UNSPECIFIED.);
#760=B_SPLINE_CURVE_WITH_KNOTS('',3,(#32396,#32397,#32398,#32399,#32400,
#32401,#32402,#32403,#32404,#32405),.UNSPECIFIED.,.F.,.F.,(4,2,2,2,4),(-4.16323414483187,
-3.10732772174226,-2.02362880934783,-0.957049330172841,-1.00000000020696E-6),
 .UNSPECIFIED.);
#761=B_SPLINE_CURVE_WITH_KNOTS('',3,(#32408,#32409,#32410,#32411,#32412,
#32413,#32414,#32415),.UNSPECIFIED.,.F.,.F.,(4,2,2,4),(-3.79953187020984,
-2.88369731719006,-1.89738143645868,-9.66593405760108E-7),.UNSPECIFIED.);
#762=B_SPLINE_CURVE_WITH_KNOTS('',3,(#32421,#32422,#32423,#32424,#32425,
#32426,#32427,#32428,#32429,#32430),.UNSPECIFIED.,.F.,.F.,(4,2,2,2,4),(-0.416082413068314,
-0.360585309636598,-0.306832956120282,-0.200050893588257,-1.00000028174785E-6),
 .UNSPECIFIED.);
#763=B_SPLINE_CURVE_WITH_KNOTS('',3,(#32432,#32433,#32434,#32435,#32436,
#32437,#32438),.UNSPECIFIED.,.F.,.F.,(4,3,4),(6.80202241033507E-5,0.000423360973853086,
0.00074564696373395),.UNSPECIFIED.);
#764=B_SPLINE_CURVE_WITH_KNOTS('',3,(#32439,#32440,#32441,#32442,#32443,
#32444,#32445,#32446,#32447,#32448,#32449,#32450),.UNSPECIFIED.,.F.,.F.,
(4,2,2,2,2,4),(-0.410791572873837,-0.314481286284345,-0.223124863886982,
-0.108117426869209,-0.0434561601514269,-1.00000038416592E-6),
 .UNSPECIFIED.);
#765=B_SPLINE_CURVE_WITH_KNOTS('',3,(#32452,#32453,#32454,#32455,#32456,
#32457,#32458,#32459,#32460,#32461),.UNSPECIFIED.,.F.,.F.,(4,2,2,2,4),(-0.416082413067571,
-0.360585309635978,-0.306832956119768,-0.200050893587991,-1.00000028163683E-6),
 .UNSPECIFIED.);
#766=B_SPLINE_CURVE_WITH_KNOTS('',3,(#32463,#32464,#32465,#32466,#32467,
#32468,#32469),.UNSPECIFIED.,.F.,.F.,(4,3,4),(6.80202241033475E-5,0.000423360973855293,
0.000745646963733951),.UNSPECIFIED.);
#767=B_SPLINE_CURVE_WITH_KNOTS('',3,(#32470,#32471,#32472,#32473,#32474,
#32475,#32476,#32477,#32478,#32479,#32480,#32481),.UNSPECIFIED.,.F.,.F.,
(4,2,2,2,2,4),(-0.410791572872332,-0.314481286283402,-0.223124863886612,
-0.108117426869205,-0.0434561601514252,-1.00000038433246E-6),
 .UNSPECIFIED.);
#768=B_SPLINE_CURVE_WITH_KNOTS('',3,(#32483,#32484,#32485,#32486,#32487,
#32488,#32489,#32490,#32491,#32492),.UNSPECIFIED.,.F.,.F.,(4,2,2,2,4),(-0.416082413068048,
-0.360584308223045,-0.30683210398761,-0.2000503380104,-1.00000028219194E-6),
 .UNSPECIFIED.);
#769=B_SPLINE_CURVE_WITH_KNOTS('',3,(#32494,#32495,#32496,#32497,#32498,
#32499,#32500),.UNSPECIFIED.,.F.,.F.,(4,3,4),(6.80202241033436E-5,0.000423360973850319,
0.000745646963733949),.UNSPECIFIED.);
#770=B_SPLINE_CURVE_WITH_KNOTS('',3,(#32502,#32503,#32504,#32505,#32506,
#32507,#32508,#32509,#32510,#32511,#32512,#32513),.UNSPECIFIED.,.F.,.F.,
(4,2,2,2,2,4),(-0.410791572872144,-0.314481286283286,-0.223124863886566,
-0.108117426869204,-0.043456160151425,-1.00000038433246E-6),
 .UNSPECIFIED.);
#771=B_SPLINE_CURVE_WITH_KNOTS('',3,(#32516,#32517,#32518,#32519,#32520,
#32521,#32522,#32523,#32524,#32525),.UNSPECIFIED.,.F.,.F.,(4,2,2,2,4),(-0.416082413068513,
-0.360585309636774,-0.306832956120457,-0.200050893588368,-1.00000028135927E-6),
 .UNSPECIFIED.);
#772=B_SPLINE_CURVE_WITH_KNOTS('',3,(#32527,#32528,#32529,#32530,#32531,
#32532,#32533),.UNSPECIFIED.,.F.,.F.,(4,3,4),(6.80202241033427E-5,0.000423360973852712,
0.00074564696373395),.UNSPECIFIED.);
#773=B_SPLINE_CURVE_WITH_KNOTS('',3,(#32534,#32535,#32536,#32537,#32538,
#32539,#32540,#32541,#32542,#32543,#32544,#32545),.UNSPECIFIED.,.F.,.F.,
(4,2,2,2,2,4),(-0.410791572872511,-0.314481286283472,-0.223124863886587,
-0.108117426869161,-0.0434561601514204,-1.00000038433246E-6),
 .UNSPECIFIED.);
#774=B_SPLINE_CURVE_WITH_KNOTS('',3,(#32547,#32548,#32549,#32550,#32551,
#32552,#32553,#32554,#32555,#32556),.UNSPECIFIED.,.F.,.F.,(4,2,2,2,4),(-0.416082413068343,
-0.360584308223297,-0.306832103987803,-0.200050338010502,-1.00000028147029E-6),
 .UNSPECIFIED.);
#775=B_SPLINE_CURVE_WITH_KNOTS('',3,(#32558,#32559,#32560,#32561,#32562,
#32563,#32564),.UNSPECIFIED.,.F.,.F.,(4,3,4),(6.80202241033462E-5,0.000423360973856063,
0.000745646963733952),.UNSPECIFIED.);
#776=B_SPLINE_CURVE_WITH_KNOTS('',3,(#32565,#32566,#32567,#32568,#32569,
#32570,#32571,#32572,#32573,#32574,#32575,#32576),.UNSPECIFIED.,.F.,.F.,
(4,2,2,2,2,4),(-0.410791572872343,-0.314480677796283,-0.223124432164779,
-0.108117217674975,-0.0434560760701422,-1.00000038427694E-6),
 .UNSPECIFIED.);
#777=B_SPLINE_CURVE_WITH_KNOTS('',3,(#32578,#32579,#32580,#32581,#32582,
#32583,#32584,#32585,#32586,#32587),.UNSPECIFIED.,.F.,.F.,(4,2,2,2,4),(-0.41608241306817,
-0.360584308223134,-0.306832103987679,-0.200050338010442,-1.00000028141478E-6),
 .UNSPECIFIED.);
#778=B_SPLINE_CURVE_WITH_KNOTS('',3,(#32589,#32590,#32591,#32592,#32593,
#32594,#32595),.UNSPECIFIED.,.F.,.F.,(4,3,4),(6.80202241033419E-5,0.000423360973850686,
0.000745646963733949),.UNSPECIFIED.);
#779=B_SPLINE_CURVE_WITH_KNOTS('',3,(#32596,#32597,#32598,#32599,#32600,
#32601,#32602,#32603,#32604,#32605,#32606,#32607),.UNSPECIFIED.,.F.,.F.,
(4,2,2,2,2,4),(-0.410791572871703,-0.314481286282978,-0.223124863886396,
-0.108117426869157,-0.0434561601514192,-1.00000038499859E-6),
 .UNSPECIFIED.);
#780=B_SPLINE_CURVE_WITH_KNOTS('',3,(#32609,#32610,#32611,#32612,#32613,
#32614,#32615,#32616,#32617,#32618),.UNSPECIFIED.,.F.,.F.,(4,2,2,2,4),(-0.416082413069045,
-0.360585309637195,-0.306832956120764,-0.200050893588512,-1.00000028130376E-6),
 .UNSPECIFIED.);
#781=B_SPLINE_CURVE_WITH_KNOTS('',3,(#32620,#32621,#32622,#32623,#32624,
#32625,#32626),.UNSPECIFIED.,.F.,.F.,(4,3,4),(6.80202241033508E-5,0.000423360973851168,
0.000745646963733949),.UNSPECIFIED.);
#782=B_SPLINE_CURVE_WITH_KNOTS('',3,(#32627,#32628,#32629,#32630,#32631,
#32632,#32633,#32634,#32635,#32636,#32637,#32638),.UNSPECIFIED.,.F.,.F.,
(4,2,2,2,2,4),(-0.410791572871773,-0.314480677795932,-0.223124432164652,
-0.108117217674975,-0.0434560760701403,-1.0000003840549E-6),
 .UNSPECIFIED.);
#783=B_SPLINE_CURVE_WITH_KNOTS('',3,(#32640,#32641,#32642,#32643,#32644,
#32645,#32646,#32647,#32648,#32649),.UNSPECIFIED.,.F.,.F.,(4,2,2,2,4),(1.00000001324041E-6,
0.635035409735681,1.24983493879194,1.87121208677302,2.08467470935283),
 .UNSPECIFIED.);
#784=B_SPLINE_CURVE_WITH_KNOTS('',3,(#32742,#32743,#32744,#32745,#32746,
#32747),.UNSPECIFIED.,.F.,.F.,(4,2,4),(-3.04622791888176,-1.52235182247481,
-1.00000000191613E-6),.UNSPECIFIED.);
#785=B_SPLINE_CURVE_WITH_KNOTS('',3,(#32750,#32751,#32752,#32753,#32754,
#32755),.UNSPECIFIED.,.F.,.F.,(4,2,4),(-3.11031182561968,-1.55397466140411,
-1.00000000147205E-6),.UNSPECIFIED.);
#786=B_SPLINE_CURVE_WITH_KNOTS('',3,(#33029,#33030,#33031,#33032,#33033,
#33034,#33035,#33036,#33037,#33038,#33039,#33040,#33041,#33042,#33043,#33044,
#33045,#33046,#33047,#33048,#33049,#33050,#33051,#33052,#33053),
 .UNSPECIFIED.,.F.,.F.,(4,3,3,3,3,3,3,3,4),(0.169188754138552,0.21259195128669,
0.318887932838093,0.389751920511185,0.460615908147183,0.566911889469088,
0.637775876850632,0.708639855735204,0.737840512980669),.UNSPECIFIED.);
#787=B_SPLINE_CURVE_WITH_KNOTS('',3,(#33054,#33055,#33056,#33057,#33058,
#33059,#33060,#33061),.UNSPECIFIED.,.F.,.F.,(4,2,2,4),(9.75623641873708E-7,
1.95229904030299,2.9045389655587,3.79841482214538),.UNSPECIFIED.);
#788=B_SPLINE_CURVE_WITH_KNOTS('',3,(#33351,#33352,#33353,#33354,#33355,
#33356,#33357,#33358,#33359,#33360),.UNSPECIFIED.,.F.,.F.,(4,2,2,2,4),(9.99999995110559E-7,
0.975019787491179,2.07352620290794,3.13207699922824,4.16223065422311),
 .UNSPECIFIED.);
#789=B_SPLINE_CURVE_WITH_KNOTS('',3,(#33651,#33652,#33653,#33654,#33655,
#33656),.UNSPECIFIED.,.F.,.F.,(4,2,4),(-3.11031182562015,-1.55397466140411,
-1.00000000147205E-6),.UNSPECIFIED.);
#790=B_SPLINE_CURVE_WITH_KNOTS('',3,(#33658,#33659,#33660,#33661,#33662,
#33663,#33664,#33665,#33666,#33667),.UNSPECIFIED.,.F.,.F.,(4,2,2,2,4),(9.99999994354565E-7,
0.975020551048607,2.07352669960846,3.13207725037619,4.16223066592058),
 .UNSPECIFIED.);
#791=B_SPLINE_CURVE_WITH_KNOTS('',3,(#33668,#33669,#33670,#33671,#33672,
#33673,#33674,#33675,#33676,#33677,#33678,#33679,#33680,#33681,#33682,#33683,
#33684,#33685,#33686,#33687,#33688,#33689,#33690,#33691,#33692),
 .UNSPECIFIED.,.F.,.F.,(4,3,3,3,3,3,3,3,4),(0.169188762886294,0.212591956720561,
0.318887932838093,0.389751920511184,0.460615908147183,0.566911889469088,
0.637775876850632,0.708639855735204,0.737840512980669),.UNSPECIFIED.);
#792=B_SPLINE_CURVE_WITH_KNOTS('',3,(#33966,#33967,#33968,#33969,#33970,
#33971,#33972,#33973),.UNSPECIFIED.,.F.,.F.,(4,2,2,4),(9.64894431166974E-7,
1.95229904275442,2.90453896597694,3.79841482198892),.UNSPECIFIED.);
#793=B_SPLINE_CURVE_WITH_KNOTS('',3,(#33974,#33975,#33976,#33977,#33978,
#33979),.UNSPECIFIED.,.F.,.F.,(4,2,4),(-3.04622791888257,-1.52235182247559,
-1.00000000236022E-6),.UNSPECIFIED.);
#794=B_SPLINE_CURVE_WITH_KNOTS('',3,(#34362,#34363,#34364,#34365,#34366,
#34367),.UNSPECIFIED.,.F.,.F.,(4,2,4),(-3.11031182562014,-1.5539746614041,
-1.00000000236022E-6),.UNSPECIFIED.);
#795=B_SPLINE_CURVE_WITH_KNOTS('',3,(#34369,#34370,#34371,#34372,#34373,
#34374,#34375,#34376,#34377,#34378),.UNSPECIFIED.,.F.,.F.,(4,2,2,2,4),(9.99999995275062E-7,
0.975019785302907,2.07352619778517,3.13207700287578,4.16223066592084),
 .UNSPECIFIED.);
#796=B_SPLINE_CURVE_WITH_KNOTS('',3,(#34379,#34380,#34381,#34382,#34383,
#34384,#34385,#34386,#34387,#34388,#34389,#34390,#34391,#34392,#34393,#34394,
#34395,#34396,#34397,#34398,#34399,#34400,#34401,#34402,#34403),
 .UNSPECIFIED.,.F.,.F.,(4,3,3,3,3,3,3,3,4),(0.169188762886294,0.212591956720561,
0.318887932838093,0.389751920511184,0.460615908147183,0.566911889469088,
0.637775876850632,0.708639855735204,0.737840512980669),.UNSPECIFIED.);
#797=B_SPLINE_CURVE_WITH_KNOTS('',3,(#34677,#34678,#34679,#34680,#34681,
#34682,#34683,#34684),.UNSPECIFIED.,.F.,.F.,(4,2,2,4),(9.64894429904643E-7,
1.95229950803617,2.90453965820161,3.7984148219903),.UNSPECIFIED.);
#798=B_SPLINE_CURVE_WITH_KNOTS('',3,(#34685,#34686,#34687,#34688,#34689,
#34690),.UNSPECIFIED.,.F.,.F.,(4,2,4),(-3.0462279188826,-1.52235182247563,
-1.00000000236022E-6),.UNSPECIFIED.);
#799=B_SPLINE_CURVE_WITH_KNOTS('',3,(#35073,#35074,#35075,#35076,#35077,
#35078),.UNSPECIFIED.,.F.,.F.,(4,2,4),(-3.11031182562016,-1.55397466140411,
-1.00000000147205E-6),.UNSPECIFIED.);
#800=B_SPLINE_CURVE_WITH_KNOTS('',3,(#35080,#35081,#35082,#35083,#35084,
#35085,#35086,#35087,#35088,#35089),.UNSPECIFIED.,.F.,.F.,(4,2,2,2,4),(9.99999995037368E-7,
0.975020551048589,2.07352669960851,3.13207725037625,4.16223066592104),
 .UNSPECIFIED.);
#801=B_SPLINE_CURVE_WITH_KNOTS('',3,(#35090,#35091,#35092,#35093,#35094,
#35095,#35096,#35097,#35098,#35099,#35100,#35101,#35102,#35103,#35104,#35105,
#35106,#35107,#35108,#35109,#35110,#35111,#35112,#35113,#35114),
 .UNSPECIFIED.,.F.,.F.,(4,3,3,3,3,3,3,3,4),(0.169188762886294,0.212591956720561,
0.318887932838093,0.389751920511184,0.460615908147183,0.566911889469088,
0.637775876850632,0.708639855735204,0.737840512980669),.UNSPECIFIED.);
#802=B_SPLINE_CURVE_WITH_KNOTS('',3,(#35388,#35389,#35390,#35391,#35392,
#35393,#35394,#35395),.UNSPECIFIED.,.F.,.F.,(4,2,2,4),(9.64894429706047E-7,
1.95229950803846,2.90453965820592,3.7984148219965),.UNSPECIFIED.);
#803=B_SPLINE_CURVE_WITH_KNOTS('',3,(#35396,#35397,#35398,#35399,#35400,
#35401),.UNSPECIFIED.,.F.,.F.,(4,2,4),(-3.04622791888258,-1.52235182247565,
-1.00000000147205E-6),.UNSPECIFIED.);
#804=B_SPLINE_CURVE_WITH_KNOTS('',3,(#35783,#35784,#35785,#35786,#35787,
#35788),.UNSPECIFIED.,.F.,.F.,(4,2,4),(-3.11031182562014,-1.5539746614041,
-1.00000000191613E-6),.UNSPECIFIED.);
#805=B_SPLINE_CURVE_WITH_KNOTS('',3,(#35789,#35790,#35791,#35792,#35793,
#35794,#35795,#35796,#35797,#35798,#35799,#35800,#35801,#35802,#35803,#35804,
#35805,#35806,#35807,#35808,#35809,#35810,#35811,#35812,#35813),
 .UNSPECIFIED.,.F.,.F.,(4,3,3,3,3,3,3,3,4),(0.169188754745471,0.212591956720561,
0.318887932838093,0.389751920511185,0.460615908147183,0.566911889469088,
0.637775876850632,0.708639855735204,0.737840512980669),.UNSPECIFIED.);
#806=B_SPLINE_CURVE_WITH_KNOTS('',3,(#36086,#36087,#36088,#36089,#36090,
#36091),.UNSPECIFIED.,.F.,.F.,(4,2,4),(-3.04622791888258,-1.5223518224756,
-1.00000000191613E-6),.UNSPECIFIED.);
#807=B_SPLINE_CURVE_WITH_KNOTS('',3,(#36473,#36474,#36475,#36476,#36477,
#36478),.UNSPECIFIED.,.F.,.F.,(4,2,4),(-3.11031182562015,-1.55397466140411,
-1.00000000147205E-6),.UNSPECIFIED.);
#808=B_SPLINE_CURVE_WITH_KNOTS('',3,(#36480,#36481,#36482,#36483,#36484,
#36485,#36486,#36487,#36488,#36489),.UNSPECIFIED.,.F.,.F.,(4,2,2,2,4),(9.99999995076136E-7,
0.975019785302952,2.07352619778527,3.13207700287592,4.16223066592085),
 .UNSPECIFIED.);
#809=B_SPLINE_CURVE_WITH_KNOTS('',3,(#36490,#36491,#36492,#36493,#36494,
#36495,#36496,#36497,#36498,#36499,#36500,#36501,#36502,#36503,#36504,#36505,
#36506,#36507,#36508,#36509,#36510,#36511,#36512,#36513,#36514),
 .UNSPECIFIED.,.F.,.F.,(4,3,3,3,3,3,3,3,4),(0.169188762886294,0.212591956720561,
0.318887932838093,0.389751920511184,0.460615908147183,0.566911889469088,
0.637775876850632,0.708639855735204,0.737840512980669),.UNSPECIFIED.);
#810=B_SPLINE_CURVE_WITH_KNOTS('',3,(#36788,#36789,#36790,#36791,#36792,
#36793,#36794,#36795),.UNSPECIFIED.,.F.,.F.,(4,2,2,4),(9.64894430459731E-7,
1.95229950803543,2.90453965820021,3.79841482198824),.UNSPECIFIED.);
#811=B_SPLINE_CURVE_WITH_KNOTS('',3,(#36796,#36797,#36798,#36799,#36800,
#36801),.UNSPECIFIED.,.F.,.F.,(4,2,4),(-3.04622791888258,-1.52235182247563,
-1.00000000102796E-6),.UNSPECIFIED.);
#812=B_SPLINE_CURVE_WITH_KNOTS('',3,(#37184,#37185,#37186,#37187,#37188,
#37189),.UNSPECIFIED.,.F.,.F.,(4,2,4),(-3.11031182562016,-1.55397466140411,
-1.00000000102796E-6),.UNSPECIFIED.);
#813=B_SPLINE_CURVE_WITH_KNOTS('',3,(#37191,#37192,#37193,#37194,#37195,
#37196,#37197,#37198,#37199,#37200),.UNSPECIFIED.,.F.,.F.,(4,2,2,2,4),(9.99999995482632E-7,
0.975020551048628,2.07352669960854,3.13207725037628,4.16223066592066),
 .UNSPECIFIED.);
#814=B_SPLINE_CURVE_WITH_KNOTS('',3,(#37201,#37202,#37203,#37204,#37205,
#37206,#37207,#37208,#37209,#37210,#37211,#37212,#37213,#37214,#37215,#37216,
#37217,#37218,#37219,#37220,#37221,#37222,#37223,#37224,#37225),
 .UNSPECIFIED.,.F.,.F.,(4,3,3,3,3,3,3,3,4),(0.169188762886294,0.212591956720561,
0.318887932838093,0.389751920511185,0.460615908147183,0.566911889469088,
0.637775876850632,0.708639855735204,0.737840512980669),.UNSPECIFIED.);
#815=B_SPLINE_CURVE_WITH_KNOTS('',3,(#37499,#37500,#37501,#37502,#37503,
#37504,#37505,#37506),.UNSPECIFIED.,.F.,.F.,(4,2,2,4),(9.64894430661712E-7,
1.95229950804045,2.90453965820967,3.7984148220019),.UNSPECIFIED.);
#816=B_SPLINE_CURVE_WITH_KNOTS('',3,(#37507,#37508,#37509,#37510,#37511,
#37512),.UNSPECIFIED.,.F.,.F.,(4,2,4),(-3.04622791888259,-1.52235182247564,
-1.00000000147205E-6),.UNSPECIFIED.);
#1009=TOROIDAL_SURFACE('',#12961,6.25,2.5);
#1010=TOROIDAL_SURFACE('',#12968,18.75,1.25);
#1011=TOROIDAL_SURFACE('',#12975,19.375,2.5);
#1719=FACE_OUTER_BOUND('',#2494,.T.);
#1720=FACE_OUTER_BOUND('',#2495,.T.);
#1721=FACE_OUTER_BOUND('',#2496,.T.);
#1722=FACE_OUTER_BOUND('',#2497,.T.);
#1723=FACE_OUTER_BOUND('',#2498,.T.);
#1724=FACE_OUTER_BOUND('',#2499,.T.);
#1725=FACE_OUTER_BOUND('',#2500,.T.);
#1726=FACE_OUTER_BOUND('',#2501,.T.);
#1727=FACE_OUTER_BOUND('',#2502,.T.);
#1728=FACE_OUTER_BOUND('',#2503,.T.);
#1729=FACE_OUTER_BOUND('',#2504,.T.);
#1730=FACE_OUTER_BOUND('',#2505,.T.);
#1731=FACE_OUTER_BOUND('',#2506,.T.);
#1732=FACE_OUTER_BOUND('',#2507,.T.);
#1733=FACE_OUTER_BOUND('',#2508,.T.);
#1734=FACE_OUTER_BOUND('',#2509,.T.);
#1735=FACE_OUTER_BOUND('',#2510,.T.);
#1736=FACE_OUTER_BOUND('',#2511,.T.);
#1737=FACE_OUTER_BOUND('',#2512,.T.);
#1738=FACE_OUTER_BOUND('',#2513,.T.);
#1739=FACE_OUTER_BOUND('',#2514,.T.);
#1740=FACE_OUTER_BOUND('',#2515,.T.);
#1741=FACE_OUTER_BOUND('',#2516,.T.);
#1742=FACE_OUTER_BOUND('',#2517,.T.);
#1743=FACE_OUTER_BOUND('',#2518,.T.);
#1744=FACE_OUTER_BOUND('',#2519,.T.);
#1745=FACE_OUTER_BOUND('',#2520,.T.);
#1746=FACE_OUTER_BOUND('',#2521,.T.);
#1747=FACE_OUTER_BOUND('',#2522,.T.);
#1748=FACE_OUTER_BOUND('',#2523,.T.);
#1749=FACE_OUTER_BOUND('',#2524,.T.);
#1750=FACE_OUTER_BOUND('',#2526,.T.);
#1751=FACE_OUTER_BOUND('',#2527,.T.);
#1752=FACE_OUTER_BOUND('',#2528,.T.);
#1753=FACE_OUTER_BOUND('',#2529,.T.);
#1754=FACE_OUTER_BOUND('',#2530,.T.);
#1755=FACE_OUTER_BOUND('',#2531,.T.);
#1756=FACE_OUTER_BOUND('',#2532,.T.);
#1757=FACE_OUTER_BOUND('',#2534,.T.);
#1758=FACE_OUTER_BOUND('',#2536,.T.);
#2494=EDGE_LOOP('',(#10331,#10332,#10333,#10334,#10335,#10336,#10337,#10338,
#10339,#10340,#10341,#10342,#10343,#10344,#10345,#10346,#10347,#10348,#10349,
#10350,#10351,#10352,#10353,#10354,#10355,#10356,#10357));
#2495=EDGE_LOOP('',(#10358,#10359,#10360,#10361));
#2496=EDGE_LOOP('',(#10362,#10363,#10364,#10365));
#2497=EDGE_LOOP('',(#10366,#10367,#10368,#10369));
#2498=EDGE_LOOP('',(#10370,#10371,#10372,#10373));
#2499=EDGE_LOOP('',(#10374,#10375,#10376));
#2500=EDGE_LOOP('',(#10377,#10378,#10379,#10380,#10381,#10382,#10383,#10384,
#10385,#10386,#10387,#10388,#10389,#10390,#10391,#10392,#10393,#10394,#10395,
#10396,#10397,#10398,#10399,#10400,#10401,#10402,#10403,#10404,#10405,#10406,
#10407,#10408,#10409));
#2501=EDGE_LOOP('',(#10410,#10411,#10412));
#2502=EDGE_LOOP('',(#10413,#10414,#10415,#10416));
#2503=EDGE_LOOP('',(#10417,#10418,#10419,#10420,#10421));
#2504=EDGE_LOOP('',(#10422,#10423,#10424,#10425,#10426));
#2505=EDGE_LOOP('',(#10427,#10428,#10429,#10430,#10431,#10432));
#2506=EDGE_LOOP('',(#10433,#10434,#10435,#10436,#10437,#10438));
#2507=EDGE_LOOP('',(#10439,#10440,#10441,#10442));
#2508=EDGE_LOOP('',(#10443,#10444,#10445,#10446,#10447));
#2509=EDGE_LOOP('',(#10448,#10449,#10450,#10451,#10452));
#2510=EDGE_LOOP('',(#10453,#10454,#10455,#10456));
#2511=EDGE_LOOP('',(#10457,#10458,#10459,#10460,#10461));
#2512=EDGE_LOOP('',(#10462,#10463,#10464,#10465,#10466));
#2513=EDGE_LOOP('',(#10467,#10468,#10469,#10470));
#2514=EDGE_LOOP('',(#10471,#10472,#10473,#10474,#10475));
#2515=EDGE_LOOP('',(#10476,#10477,#10478,#10479,#10480));
#2516=EDGE_LOOP('',(#10481,#10482,#10483,#10484));
#2517=EDGE_LOOP('',(#10485,#10486,#10487,#10488,#10489));
#2518=EDGE_LOOP('',(#10490,#10491,#10492,#10493,#10494));
#2519=EDGE_LOOP('',(#10495,#10496,#10497,#10498));
#2520=EDGE_LOOP('',(#10499,#10500,#10501,#10502,#10503));
#2521=EDGE_LOOP('',(#10504,#10505,#10506,#10507,#10508));
#2522=EDGE_LOOP('',(#10509,#10510,#10511,#10512));
#2523=EDGE_LOOP('',(#10513));
#2524=EDGE_LOOP('',(#10514));
#2525=EDGE_LOOP('',(#10515));
#2526=EDGE_LOOP('',(#10516,#10517,#10518));
#2527=EDGE_LOOP('',(#10519,#10520,#10521));
#2528=EDGE_LOOP('',(#10522,#10523,#10524));
#2529=EDGE_LOOP('',(#10525,#10526,#10527));
#2530=EDGE_LOOP('',(#10528,#10529,#10530));
#2531=EDGE_LOOP('',(#10531,#10532,#10533));
#2532=EDGE_LOOP('',(#10534));
#2533=EDGE_LOOP('',(#10535));
#2534=EDGE_LOOP('',(#10536));
#2535=EDGE_LOOP('',(#10537));
#2536=EDGE_LOOP('',(#10538));
#2964=LINE('',#32200,#3402);
#2965=LINE('',#32361,#3403);
#2966=LINE('',#32381,#3404);
#2967=LINE('',#32391,#3405);
#2968=LINE('',#32407,#3406);
#2969=LINE('',#32749,#3407);
#2970=LINE('',#34071,#3408);
#2971=LINE('',#34782,#3409);
#2972=LINE('',#35493,#3410);
#2973=LINE('',#36893,#3411);
#2974=LINE('',#37604,#3412);
#3402=VECTOR('',#16282,21.875);
#3403=VECTOR('',#16299,21.875);
#3404=VECTOR('',#16312,1.875);
#3405=VECTOR('',#16325,20.);
#3406=VECTOR('',#16330,10.);
#3407=VECTOR('',#16341,10.);
#3408=VECTOR('',#16342,10.);
#3409=VECTOR('',#16343,10.);
#3410=VECTOR('',#16344,10.);
#3411=VECTOR('',#16345,10.);
#3412=VECTOR('',#16346,10.);
#4280=CIRCLE('',#12952,21.875);
#4281=CIRCLE('',#12953,21.875);
#4282=CIRCLE('',#12954,21.875);
#4283=CIRCLE('',#12955,21.875);
#4284=CIRCLE('',#12956,21.875);
#4285=CIRCLE('',#12957,21.875);
#4286=CIRCLE('',#12958,21.875);
#4287=CIRCLE('',#12959,21.875);
#4288=CIRCLE('',#12960,21.875);
#4289=CIRCLE('',#12962,3.75);
#4290=CIRCLE('',#12963,2.5);
#4291=CIRCLE('',#12964,6.25);
#4292=CIRCLE('',#12966,1.875);
#4293=CIRCLE('',#12967,1.875);
#4294=CIRCLE('',#12969,18.75);
#4295=CIRCLE('',#12970,1.25);
#4296=CIRCLE('',#12971,20.);
#4297=CIRCLE('',#12973,20.);
#4298=CIRCLE('',#12976,19.375);
#4299=CIRCLE('',#12977,2.5);
#4300=CIRCLE('',#12978,21.875);
#5238=VERTEX_POINT('',#32197);
#5239=VERTEX_POINT('',#32199);
#5240=VERTEX_POINT('',#32201);
#5241=VERTEX_POINT('',#32212);
#5242=VERTEX_POINT('',#32214);
#5243=VERTEX_POINT('',#32225);
#5244=VERTEX_POINT('',#32236);
#5245=VERTEX_POINT('',#32238);
#5246=VERTEX_POINT('',#32249);
#5247=VERTEX_POINT('',#32260);
#5248=VERTEX_POINT('',#32262);
#5249=VERTEX_POINT('',#32264);
#5250=VERTEX_POINT('',#32275);
#5251=VERTEX_POINT('',#32286);
#5252=VERTEX_POINT('',#32288);
#5253=VERTEX_POINT('',#32299);
#5254=VERTEX_POINT('',#32310);
#5255=VERTEX_POINT('',#32312);
#5256=VERTEX_POINT('',#32323);
#5257=VERTEX_POINT('',#32334);
#5258=VERTEX_POINT('',#32336);
#5259=VERTEX_POINT('',#32347);
#5260=VERTEX_POINT('',#32358);
#5261=VERTEX_POINT('',#32360);
#5262=VERTEX_POINT('',#32362);
#5263=VERTEX_POINT('',#32372);
#5264=VERTEX_POINT('',#32374);
#5265=VERTEX_POINT('',#32378);
#5266=VERTEX_POINT('',#32380);
#5267=VERTEX_POINT('',#32384);
#5268=VERTEX_POINT('',#32386);
#5269=VERTEX_POINT('',#32390);
#5270=VERTEX_POINT('',#32394);
#5271=VERTEX_POINT('',#32395);
#5272=VERTEX_POINT('',#32406);
#5273=VERTEX_POINT('',#32417);
#5274=VERTEX_POINT('',#32420);
#5275=VERTEX_POINT('',#32431);
#5276=VERTEX_POINT('',#32451);
#5277=VERTEX_POINT('',#32462);
#5278=VERTEX_POINT('',#32482);
#5279=VERTEX_POINT('',#32493);
#5280=VERTEX_POINT('',#32501);
#5281=VERTEX_POINT('',#32515);
#5282=VERTEX_POINT('',#32526);
#5283=VERTEX_POINT('',#32546);
#5284=VERTEX_POINT('',#32557);
#5285=VERTEX_POINT('',#32577);
#5286=VERTEX_POINT('',#32588);
#5287=VERTEX_POINT('',#32608);
#5288=VERTEX_POINT('',#32619);
#5289=VERTEX_POINT('',#32741);
#5290=VERTEX_POINT('',#32748);
#5291=VERTEX_POINT('',#33028);
#5292=VERTEX_POINT('',#33650);
#5293=VERTEX_POINT('',#33657);
#5294=VERTEX_POINT('',#33965);
#5295=VERTEX_POINT('',#34361);
#5296=VERTEX_POINT('',#34368);
#5297=VERTEX_POINT('',#34676);
#5298=VERTEX_POINT('',#35072);
#5299=VERTEX_POINT('',#35079);
#5300=VERTEX_POINT('',#35387);
#5301=VERTEX_POINT('',#36472);
#5302=VERTEX_POINT('',#36479);
#5303=VERTEX_POINT('',#36787);
#5304=VERTEX_POINT('',#37183);
#5305=VERTEX_POINT('',#37190);
#5306=VERTEX_POINT('',#37498);
#6947=EDGE_CURVE('',#5238,#5238,#4280,.T.);
#6948=EDGE_CURVE('',#5238,#5239,#2964,.T.);
#6949=EDGE_CURVE('',#5239,#5240,#745,.T.);
#6950=EDGE_CURVE('',#5240,#5241,#4281,.T.);
#6951=EDGE_CURVE('',#5241,#5242,#746,.T.);
#6952=EDGE_CURVE('',#5242,#5243,#747,.T.);
#6953=EDGE_CURVE('',#5243,#5244,#4282,.T.);
#6954=EDGE_CURVE('',#5244,#5245,#748,.T.);
#6955=EDGE_CURVE('',#5245,#5246,#749,.T.);
#6956=EDGE_CURVE('',#5246,#5247,#4283,.T.);
#6957=EDGE_CURVE('',#5247,#5248,#4284,.T.);
#6958=EDGE_CURVE('',#5248,#5249,#750,.T.);
#6959=EDGE_CURVE('',#5249,#5250,#751,.F.);
#6960=EDGE_CURVE('',#5250,#5251,#4285,.T.);
#6961=EDGE_CURVE('',#5251,#5252,#752,.T.);
#6962=EDGE_CURVE('',#5252,#5253,#753,.T.);
#6963=EDGE_CURVE('',#5253,#5254,#4286,.T.);
#6964=EDGE_CURVE('',#5254,#5255,#754,.T.);
#6965=EDGE_CURVE('',#5255,#5256,#755,.T.);
#6966=EDGE_CURVE('',#5256,#5257,#4287,.T.);
#6967=EDGE_CURVE('',#5257,#5258,#756,.T.);
#6968=EDGE_CURVE('',#5258,#5259,#757,.T.);
#6969=EDGE_CURVE('',#5259,#5260,#4288,.T.);
#6970=EDGE_CURVE('',#5261,#5260,#2965,.T.);
#6971=EDGE_CURVE('',#5261,#5262,#758,.T.);
#6972=EDGE_CURVE('',#5262,#5239,#759,.T.);
#6973=EDGE_CURVE('',#5263,#5263,#4289,.T.);
#6974=EDGE_CURVE('',#5263,#5264,#4290,.T.);
#6975=EDGE_CURVE('',#5264,#5264,#4291,.T.);
#6976=EDGE_CURVE('',#5265,#5265,#4292,.T.);
#6977=EDGE_CURVE('',#5265,#5266,#2966,.T.);
#6978=EDGE_CURVE('',#5266,#5266,#4293,.T.);
#6979=EDGE_CURVE('',#5267,#5267,#4294,.T.);
#6980=EDGE_CURVE('',#5267,#5268,#4295,.T.);
#6981=EDGE_CURVE('',#5268,#5268,#4296,.T.);
#6982=EDGE_CURVE('',#5268,#5269,#2967,.T.);
#6983=EDGE_CURVE('',#5269,#5269,#4297,.T.);
#6984=EDGE_CURVE('',#5270,#5271,#760,.F.);
#6985=EDGE_CURVE('',#5272,#5270,#2968,.T.);
#6986=EDGE_CURVE('',#5271,#5272,#761,.F.);
#6987=EDGE_CURVE('',#5273,#5273,#4298,.T.);
#6988=EDGE_CURVE('',#5273,#5247,#4299,.T.);
#6989=EDGE_CURVE('',#5274,#5246,#762,.T.);
#6990=EDGE_CURVE('',#5275,#5274,#763,.T.);
#6991=EDGE_CURVE('',#5244,#5275,#764,.T.);
#6992=EDGE_CURVE('',#5276,#5243,#765,.T.);
#6993=EDGE_CURVE('',#5277,#5276,#766,.T.);
#6994=EDGE_CURVE('',#5241,#5277,#767,.T.);
#6995=EDGE_CURVE('',#5278,#5240,#768,.T.);
#6996=EDGE_CURVE('',#5279,#5278,#769,.T.);
#6997=EDGE_CURVE('',#5280,#5279,#770,.T.);
#6998=EDGE_CURVE('',#5260,#5280,#4300,.T.);
#6999=EDGE_CURVE('',#5281,#5259,#771,.T.);
#7000=EDGE_CURVE('',#5282,#5281,#772,.T.);
#7001=EDGE_CURVE('',#5257,#5282,#773,.T.);
#7002=EDGE_CURVE('',#5283,#5256,#774,.T.);
#7003=EDGE_CURVE('',#5284,#5283,#775,.T.);
#7004=EDGE_CURVE('',#5254,#5284,#776,.T.);
#7005=EDGE_CURVE('',#5285,#5253,#777,.T.);
#7006=EDGE_CURVE('',#5286,#5285,#778,.T.);
#7007=EDGE_CURVE('',#5251,#5286,#779,.T.);
#7008=EDGE_CURVE('',#5287,#5250,#780,.T.);
#7009=EDGE_CURVE('',#5288,#5287,#781,.T.);
#7010=EDGE_CURVE('',#5248,#5288,#782,.T.);
#7011=EDGE_CURVE('',#5280,#5261,#783,.T.);
#7012=EDGE_CURVE('',#5281,#5289,#784,.T.);
#7013=EDGE_CURVE('',#5289,#5290,#2969,.T.);
#7014=EDGE_CURVE('',#5290,#5282,#785,.T.);
#7015=EDGE_CURVE('',#5291,#5258,#786,.T.);
#7016=EDGE_CURVE('',#5291,#5289,#787,.T.);
#7017=EDGE_CURVE('',#5290,#5291,#788,.T.);
#7018=EDGE_CURVE('',#5292,#5279,#789,.T.);
#7019=EDGE_CURVE('',#5292,#5293,#790,.T.);
#7020=EDGE_CURVE('',#5293,#5262,#791,.T.);
#7021=EDGE_CURVE('',#5293,#5294,#792,.T.);
#7022=EDGE_CURVE('',#5278,#5294,#793,.T.);
#7023=EDGE_CURVE('',#5294,#5292,#2970,.T.);
#7024=EDGE_CURVE('',#5295,#5277,#794,.T.);
#7025=EDGE_CURVE('',#5295,#5296,#795,.T.);
#7026=EDGE_CURVE('',#5296,#5242,#796,.T.);
#7027=EDGE_CURVE('',#5296,#5297,#797,.T.);
#7028=EDGE_CURVE('',#5276,#5297,#798,.T.);
#7029=EDGE_CURVE('',#5297,#5295,#2971,.T.);
#7030=EDGE_CURVE('',#5298,#5275,#799,.T.);
#7031=EDGE_CURVE('',#5298,#5299,#800,.T.);
#7032=EDGE_CURVE('',#5299,#5245,#801,.T.);
#7033=EDGE_CURVE('',#5299,#5300,#802,.T.);
#7034=EDGE_CURVE('',#5274,#5300,#803,.T.);
#7035=EDGE_CURVE('',#5300,#5298,#2972,.T.);
#7036=EDGE_CURVE('',#5270,#5288,#804,.T.);
#7037=EDGE_CURVE('',#5271,#5249,#805,.T.);
#7038=EDGE_CURVE('',#5287,#5272,#806,.T.);
#7039=EDGE_CURVE('',#5301,#5286,#807,.T.);
#7040=EDGE_CURVE('',#5301,#5302,#808,.T.);
#7041=EDGE_CURVE('',#5302,#5252,#809,.T.);
#7042=EDGE_CURVE('',#5302,#5303,#810,.T.);
#7043=EDGE_CURVE('',#5285,#5303,#811,.T.);
#7044=EDGE_CURVE('',#5303,#5301,#2973,.T.);
#7045=EDGE_CURVE('',#5304,#5284,#812,.T.);
#7046=EDGE_CURVE('',#5304,#5305,#813,.T.);
#7047=EDGE_CURVE('',#5305,#5255,#814,.T.);
#7048=EDGE_CURVE('',#5305,#5306,#815,.T.);
#7049=EDGE_CURVE('',#5283,#5306,#816,.T.);
#7050=EDGE_CURVE('',#5306,#5304,#2974,.T.);
#10331=ORIENTED_EDGE('',*,*,#6947,.T.);
#10332=ORIENTED_EDGE('',*,*,#6948,.T.);
#10333=ORIENTED_EDGE('',*,*,#6949,.T.);
#10334=ORIENTED_EDGE('',*,*,#6950,.T.);
#10335=ORIENTED_EDGE('',*,*,#6951,.T.);
#10336=ORIENTED_EDGE('',*,*,#6952,.T.);
#10337=ORIENTED_EDGE('',*,*,#6953,.T.);
#10338=ORIENTED_EDGE('',*,*,#6954,.T.);
#10339=ORIENTED_EDGE('',*,*,#6955,.T.);
#10340=ORIENTED_EDGE('',*,*,#6956,.T.);
#10341=ORIENTED_EDGE('',*,*,#6957,.T.);
#10342=ORIENTED_EDGE('',*,*,#6958,.T.);
#10343=ORIENTED_EDGE('',*,*,#6959,.T.);
#10344=ORIENTED_EDGE('',*,*,#6960,.T.);
#10345=ORIENTED_EDGE('',*,*,#6961,.T.);
#10346=ORIENTED_EDGE('',*,*,#6962,.T.);
#10347=ORIENTED_EDGE('',*,*,#6963,.T.);
#10348=ORIENTED_EDGE('',*,*,#6964,.T.);
#10349=ORIENTED_EDGE('',*,*,#6965,.T.);
#10350=ORIENTED_EDGE('',*,*,#6966,.T.);
#10351=ORIENTED_EDGE('',*,*,#6967,.T.);
#10352=ORIENTED_EDGE('',*,*,#6968,.T.);
#10353=ORIENTED_EDGE('',*,*,#6969,.T.);
#10354=ORIENTED_EDGE('',*,*,#6970,.F.);
#10355=ORIENTED_EDGE('',*,*,#6971,.T.);
#10356=ORIENTED_EDGE('',*,*,#6972,.T.);
#10357=ORIENTED_EDGE('',*,*,#6948,.F.);
#10358=ORIENTED_EDGE('',*,*,#6973,.F.);
#10359=ORIENTED_EDGE('',*,*,#6974,.T.);
#10360=ORIENTED_EDGE('',*,*,#6975,.F.);
#10361=ORIENTED_EDGE('',*,*,#6974,.F.);
#10362=ORIENTED_EDGE('',*,*,#6976,.T.);
#10363=ORIENTED_EDGE('',*,*,#6977,.T.);
#10364=ORIENTED_EDGE('',*,*,#6978,.T.);
#10365=ORIENTED_EDGE('',*,*,#6977,.F.);
#10366=ORIENTED_EDGE('',*,*,#6979,.F.);
#10367=ORIENTED_EDGE('',*,*,#6980,.T.);
#10368=ORIENTED_EDGE('',*,*,#6981,.F.);
#10369=ORIENTED_EDGE('',*,*,#6980,.F.);
#10370=ORIENTED_EDGE('',*,*,#6981,.T.);
#10371=ORIENTED_EDGE('',*,*,#6982,.T.);
#10372=ORIENTED_EDGE('',*,*,#6983,.T.);
#10373=ORIENTED_EDGE('',*,*,#6982,.F.);
#10374=ORIENTED_EDGE('',*,*,#6984,.F.);
#10375=ORIENTED_EDGE('',*,*,#6985,.F.);
#10376=ORIENTED_EDGE('',*,*,#6986,.F.);
#10377=ORIENTED_EDGE('',*,*,#6987,.F.);
#10378=ORIENTED_EDGE('',*,*,#6988,.T.);
#10379=ORIENTED_EDGE('',*,*,#6956,.F.);
#10380=ORIENTED_EDGE('',*,*,#6989,.F.);
#10381=ORIENTED_EDGE('',*,*,#6990,.F.);
#10382=ORIENTED_EDGE('',*,*,#6991,.F.);
#10383=ORIENTED_EDGE('',*,*,#6953,.F.);
#10384=ORIENTED_EDGE('',*,*,#6992,.F.);
#10385=ORIENTED_EDGE('',*,*,#6993,.F.);
#10386=ORIENTED_EDGE('',*,*,#6994,.F.);
#10387=ORIENTED_EDGE('',*,*,#6950,.F.);
#10388=ORIENTED_EDGE('',*,*,#6995,.F.);
#10389=ORIENTED_EDGE('',*,*,#6996,.F.);
#10390=ORIENTED_EDGE('',*,*,#6997,.F.);
#10391=ORIENTED_EDGE('',*,*,#6998,.F.);
#10392=ORIENTED_EDGE('',*,*,#6969,.F.);
#10393=ORIENTED_EDGE('',*,*,#6999,.F.);
#10394=ORIENTED_EDGE('',*,*,#7000,.F.);
#10395=ORIENTED_EDGE('',*,*,#7001,.F.);
#10396=ORIENTED_EDGE('',*,*,#6966,.F.);
#10397=ORIENTED_EDGE('',*,*,#7002,.F.);
#10398=ORIENTED_EDGE('',*,*,#7003,.F.);
#10399=ORIENTED_EDGE('',*,*,#7004,.F.);
#10400=ORIENTED_EDGE('',*,*,#6963,.F.);
#10401=ORIENTED_EDGE('',*,*,#7005,.F.);
#10402=ORIENTED_EDGE('',*,*,#7006,.F.);
#10403=ORIENTED_EDGE('',*,*,#7007,.F.);
#10404=ORIENTED_EDGE('',*,*,#6960,.F.);
#10405=ORIENTED_EDGE('',*,*,#7008,.F.);
#10406=ORIENTED_EDGE('',*,*,#7009,.F.);
#10407=ORIENTED_EDGE('',*,*,#7010,.F.);
#10408=ORIENTED_EDGE('',*,*,#6957,.F.);
#10409=ORIENTED_EDGE('',*,*,#6988,.F.);
#10410=ORIENTED_EDGE('',*,*,#6970,.T.);
#10411=ORIENTED_EDGE('',*,*,#6998,.T.);
#10412=ORIENTED_EDGE('',*,*,#7011,.T.);
#10413=ORIENTED_EDGE('',*,*,#7012,.T.);
#10414=ORIENTED_EDGE('',*,*,#7013,.T.);
#10415=ORIENTED_EDGE('',*,*,#7014,.T.);
#10416=ORIENTED_EDGE('',*,*,#7000,.T.);
#10417=ORIENTED_EDGE('',*,*,#7015,.F.);
#10418=ORIENTED_EDGE('',*,*,#7016,.T.);
#10419=ORIENTED_EDGE('',*,*,#7012,.F.);
#10420=ORIENTED_EDGE('',*,*,#6999,.T.);
#10421=ORIENTED_EDGE('',*,*,#6968,.F.);
#10422=ORIENTED_EDGE('',*,*,#7014,.F.);
#10423=ORIENTED_EDGE('',*,*,#7017,.T.);
#10424=ORIENTED_EDGE('',*,*,#7015,.T.);
#10425=ORIENTED_EDGE('',*,*,#6967,.F.);
#10426=ORIENTED_EDGE('',*,*,#7001,.T.);
#10427=ORIENTED_EDGE('',*,*,#7018,.F.);
#10428=ORIENTED_EDGE('',*,*,#7019,.T.);
#10429=ORIENTED_EDGE('',*,*,#7020,.T.);
#10430=ORIENTED_EDGE('',*,*,#6971,.F.);
#10431=ORIENTED_EDGE('',*,*,#7011,.F.);
#10432=ORIENTED_EDGE('',*,*,#6997,.T.);
#10433=ORIENTED_EDGE('',*,*,#7020,.F.);
#10434=ORIENTED_EDGE('',*,*,#7021,.T.);
#10435=ORIENTED_EDGE('',*,*,#7022,.F.);
#10436=ORIENTED_EDGE('',*,*,#6995,.T.);
#10437=ORIENTED_EDGE('',*,*,#6949,.F.);
#10438=ORIENTED_EDGE('',*,*,#6972,.F.);
#10439=ORIENTED_EDGE('',*,*,#7022,.T.);
#10440=ORIENTED_EDGE('',*,*,#7023,.T.);
#10441=ORIENTED_EDGE('',*,*,#7018,.T.);
#10442=ORIENTED_EDGE('',*,*,#6996,.T.);
#10443=ORIENTED_EDGE('',*,*,#7024,.F.);
#10444=ORIENTED_EDGE('',*,*,#7025,.T.);
#10445=ORIENTED_EDGE('',*,*,#7026,.T.);
#10446=ORIENTED_EDGE('',*,*,#6951,.F.);
#10447=ORIENTED_EDGE('',*,*,#6994,.T.);
#10448=ORIENTED_EDGE('',*,*,#7026,.F.);
#10449=ORIENTED_EDGE('',*,*,#7027,.T.);
#10450=ORIENTED_EDGE('',*,*,#7028,.F.);
#10451=ORIENTED_EDGE('',*,*,#6992,.T.);
#10452=ORIENTED_EDGE('',*,*,#6952,.F.);
#10453=ORIENTED_EDGE('',*,*,#7028,.T.);
#10454=ORIENTED_EDGE('',*,*,#7029,.T.);
#10455=ORIENTED_EDGE('',*,*,#7024,.T.);
#10456=ORIENTED_EDGE('',*,*,#6993,.T.);
#10457=ORIENTED_EDGE('',*,*,#7030,.F.);
#10458=ORIENTED_EDGE('',*,*,#7031,.T.);
#10459=ORIENTED_EDGE('',*,*,#7032,.T.);
#10460=ORIENTED_EDGE('',*,*,#6954,.F.);
#10461=ORIENTED_EDGE('',*,*,#6991,.T.);
#10462=ORIENTED_EDGE('',*,*,#7032,.F.);
#10463=ORIENTED_EDGE('',*,*,#7033,.T.);
#10464=ORIENTED_EDGE('',*,*,#7034,.F.);
#10465=ORIENTED_EDGE('',*,*,#6989,.T.);
#10466=ORIENTED_EDGE('',*,*,#6955,.F.);
#10467=ORIENTED_EDGE('',*,*,#7034,.T.);
#10468=ORIENTED_EDGE('',*,*,#7035,.T.);
#10469=ORIENTED_EDGE('',*,*,#7030,.T.);
#10470=ORIENTED_EDGE('',*,*,#6990,.T.);
#10471=ORIENTED_EDGE('',*,*,#7036,.F.);
#10472=ORIENTED_EDGE('',*,*,#6984,.T.);
#10473=ORIENTED_EDGE('',*,*,#7037,.T.);
#10474=ORIENTED_EDGE('',*,*,#6958,.F.);
#10475=ORIENTED_EDGE('',*,*,#7010,.T.);
#10476=ORIENTED_EDGE('',*,*,#7037,.F.);
#10477=ORIENTED_EDGE('',*,*,#6986,.T.);
#10478=ORIENTED_EDGE('',*,*,#7038,.F.);
#10479=ORIENTED_EDGE('',*,*,#7008,.T.);
#10480=ORIENTED_EDGE('',*,*,#6959,.F.);
#10481=ORIENTED_EDGE('',*,*,#7038,.T.);
#10482=ORIENTED_EDGE('',*,*,#6985,.T.);
#10483=ORIENTED_EDGE('',*,*,#7036,.T.);
#10484=ORIENTED_EDGE('',*,*,#7009,.T.);
#10485=ORIENTED_EDGE('',*,*,#7039,.F.);
#10486=ORIENTED_EDGE('',*,*,#7040,.T.);
#10487=ORIENTED_EDGE('',*,*,#7041,.T.);
#10488=ORIENTED_EDGE('',*,*,#6961,.F.);
#10489=ORIENTED_EDGE('',*,*,#7007,.T.);
#10490=ORIENTED_EDGE('',*,*,#7041,.F.);
#10491=ORIENTED_EDGE('',*,*,#7042,.T.);
#10492=ORIENTED_EDGE('',*,*,#7043,.F.);
#10493=ORIENTED_EDGE('',*,*,#7005,.T.);
#10494=ORIENTED_EDGE('',*,*,#6962,.F.);
#10495=ORIENTED_EDGE('',*,*,#7043,.T.);
#10496=ORIENTED_EDGE('',*,*,#7044,.T.);
#10497=ORIENTED_EDGE('',*,*,#7039,.T.);
#10498=ORIENTED_EDGE('',*,*,#7006,.T.);
#10499=ORIENTED_EDGE('',*,*,#7045,.F.);
#10500=ORIENTED_EDGE('',*,*,#7046,.T.);
#10501=ORIENTED_EDGE('',*,*,#7047,.T.);
#10502=ORIENTED_EDGE('',*,*,#6964,.F.);
#10503=ORIENTED_EDGE('',*,*,#7004,.T.);
#10504=ORIENTED_EDGE('',*,*,#7047,.F.);
#10505=ORIENTED_EDGE('',*,*,#7048,.T.);
#10506=ORIENTED_EDGE('',*,*,#7049,.F.);
#10507=ORIENTED_EDGE('',*,*,#7002,.T.);
#10508=ORIENTED_EDGE('',*,*,#6965,.F.);
#10509=ORIENTED_EDGE('',*,*,#7049,.T.);
#10510=ORIENTED_EDGE('',*,*,#7050,.T.);
#10511=ORIENTED_EDGE('',*,*,#7045,.T.);
#10512=ORIENTED_EDGE('',*,*,#7003,.T.);
#10513=ORIENTED_EDGE('',*,*,#6987,.T.);
#10514=ORIENTED_EDGE('',*,*,#6947,.F.);
#10515=ORIENTED_EDGE('',*,*,#6983,.F.);
#10516=ORIENTED_EDGE('',*,*,#7050,.F.);
#10517=ORIENTED_EDGE('',*,*,#7048,.F.);
#10518=ORIENTED_EDGE('',*,*,#7046,.F.);
#10519=ORIENTED_EDGE('',*,*,#7044,.F.);
#10520=ORIENTED_EDGE('',*,*,#7042,.F.);
#10521=ORIENTED_EDGE('',*,*,#7040,.F.);
#10522=ORIENTED_EDGE('',*,*,#7035,.F.);
#10523=ORIENTED_EDGE('',*,*,#7033,.F.);
#10524=ORIENTED_EDGE('',*,*,#7031,.F.);
#10525=ORIENTED_EDGE('',*,*,#7029,.F.);
#10526=ORIENTED_EDGE('',*,*,#7027,.F.);
#10527=ORIENTED_EDGE('',*,*,#7025,.F.);
#10528=ORIENTED_EDGE('',*,*,#7023,.F.);
#10529=ORIENTED_EDGE('',*,*,#7021,.F.);
#10530=ORIENTED_EDGE('',*,*,#7019,.F.);
#10531=ORIENTED_EDGE('',*,*,#7016,.F.);
#10532=ORIENTED_EDGE('',*,*,#7017,.F.);
#10533=ORIENTED_EDGE('',*,*,#7013,.F.);
#10534=ORIENTED_EDGE('',*,*,#6979,.T.);
#10535=ORIENTED_EDGE('',*,*,#6975,.T.);
#10536=ORIENTED_EDGE('',*,*,#6973,.T.);
#10537=ORIENTED_EDGE('',*,*,#6976,.F.);
#10538=ORIENTED_EDGE('',*,*,#6978,.F.);
#10739=CYLINDRICAL_SURFACE('',#12951,21.875);
#10740=CYLINDRICAL_SURFACE('',#12965,1.875);
#10741=CYLINDRICAL_SURFACE('',#12972,20.);
#10742=CYLINDRICAL_SURFACE('',#12974,46.875);
#10743=CYLINDRICAL_SURFACE('',#12979,21.875);
#10744=CYLINDRICAL_SURFACE('',#12982,46.875);
#10745=CYLINDRICAL_SURFACE('',#12983,46.875);
#10746=CYLINDRICAL_SURFACE('',#12984,46.875);
#10747=CYLINDRICAL_SURFACE('',#12985,46.875);
#10748=CYLINDRICAL_SURFACE('',#12986,46.875);
#10749=CYLINDRICAL_SURFACE('',#12987,46.875);
#11457=ADVANCED_FACE('',(#1719),#10739,.T.);
#11458=ADVANCED_FACE('',(#1720),#1009,.F.);
#11459=ADVANCED_FACE('',(#1721),#10740,.F.);
#11460=ADVANCED_FACE('',(#1722),#1010,.F.);
#11461=ADVANCED_FACE('',(#1723),#10741,.F.);
#11462=ADVANCED_FACE('',(#1724),#10742,.T.);
#11463=ADVANCED_FACE('',(#1725),#1011,.T.);
#11464=ADVANCED_FACE('',(#1726),#10743,.T.);
#11465=ADVANCED_FACE('',(#1727),#243,.T.);
#11466=ADVANCED_FACE('',(#1728),#244,.T.);
#11467=ADVANCED_FACE('',(#1729),#245,.T.);
#11468=ADVANCED_FACE('',(#1730),#246,.T.);
#11469=ADVANCED_FACE('',(#1731),#247,.T.);
#11470=ADVANCED_FACE('',(#1732),#248,.T.);
#11471=ADVANCED_FACE('',(#1733),#249,.T.);
#11472=ADVANCED_FACE('',(#1734),#250,.T.);
#11473=ADVANCED_FACE('',(#1735),#251,.T.);
#11474=ADVANCED_FACE('',(#1736),#252,.T.);
#11475=ADVANCED_FACE('',(#1737),#253,.T.);
#11476=ADVANCED_FACE('',(#1738),#254,.T.);
#11477=ADVANCED_FACE('',(#1739),#255,.T.);
#11478=ADVANCED_FACE('',(#1740),#256,.T.);
#11479=ADVANCED_FACE('',(#1741),#257,.T.);
#11480=ADVANCED_FACE('',(#1742),#258,.T.);
#11481=ADVANCED_FACE('',(#1743),#259,.T.);
#11482=ADVANCED_FACE('',(#1744),#260,.T.);
#11483=ADVANCED_FACE('',(#1745),#261,.T.);
#11484=ADVANCED_FACE('',(#1746),#262,.T.);
#11485=ADVANCED_FACE('',(#1747),#263,.T.);
#11486=ADVANCED_FACE('',(#1748),#414,.T.);
#11487=ADVANCED_FACE('',(#1749,#312),#415,.F.);
#11488=ADVANCED_FACE('',(#1750),#10744,.T.);
#11489=ADVANCED_FACE('',(#1751),#10745,.T.);
#11490=ADVANCED_FACE('',(#1752),#10746,.T.);
#11491=ADVANCED_FACE('',(#1753),#10747,.T.);
#11492=ADVANCED_FACE('',(#1754),#10748,.T.);
#11493=ADVANCED_FACE('',(#1755),#10749,.T.);
#11494=ADVANCED_FACE('',(#1756,#313),#416,.T.);
#11495=ADVANCED_FACE('',(#1757,#314),#417,.T.);
#11496=ADVANCED_FACE('',(#1758),#418,.T.);
#11498=CLOSED_SHELL('',(#11457,#11458,#11459,#11460,#11461,#11462,#11463,
#11464,#11465,#11466,#11467,#11468,#11469,#11470,#11471,#11472,#11473,#11474,
#11475,#11476,#11477,#11478,#11479,#11480,#11481,#11482,#11483,#11484,#11485,
#11486,#11487,#11488,#11489,#11490,#11491,#11492,#11493,#11494,#11495,#11496));
#12950=AXIS2_PLACEMENT_3D('',#32195,#16276,#16277);
#12951=AXIS2_PLACEMENT_3D('',#32196,#16278,#16279);
#12952=AXIS2_PLACEMENT_3D('',#32198,#16280,#16281);
#12953=AXIS2_PLACEMENT_3D('',#32213,#16283,#16284);
#12954=AXIS2_PLACEMENT_3D('',#32237,#16285,#16286);
#12955=AXIS2_PLACEMENT_3D('',#32261,#16287,#16288);
#12956=AXIS2_PLACEMENT_3D('',#32263,#16289,#16290);
#12957=AXIS2_PLACEMENT_3D('',#32287,#16291,#16292);
#12958=AXIS2_PLACEMENT_3D('',#32311,#16293,#16294);
#12959=AXIS2_PLACEMENT_3D('',#32335,#16295,#16296);
#12960=AXIS2_PLACEMENT_3D('',#32359,#16297,#16298);
#12961=AXIS2_PLACEMENT_3D('',#32371,#16300,#16301);
#12962=AXIS2_PLACEMENT_3D('',#32373,#16302,#16303);
#12963=AXIS2_PLACEMENT_3D('',#32375,#16304,#16305);
#12964=AXIS2_PLACEMENT_3D('',#32376,#16306,#16307);
#12965=AXIS2_PLACEMENT_3D('',#32377,#16308,#16309);
#12966=AXIS2_PLACEMENT_3D('',#32379,#16310,#16311);
#12967=AXIS2_PLACEMENT_3D('',#32382,#16313,#16314);
#12968=AXIS2_PLACEMENT_3D('',#32383,#16315,#16316);
#12969=AXIS2_PLACEMENT_3D('',#32385,#16317,#16318);
#12970=AXIS2_PLACEMENT_3D('',#32387,#16319,#16320);
#12971=AXIS2_PLACEMENT_3D('',#32388,#16321,#16322);
#12972=AXIS2_PLACEMENT_3D('',#32389,#16323,#16324);
#12973=AXIS2_PLACEMENT_3D('',#32392,#16326,#16327);
#12974=AXIS2_PLACEMENT_3D('',#32393,#16328,#16329);
#12975=AXIS2_PLACEMENT_3D('',#32416,#16331,#16332);
#12976=AXIS2_PLACEMENT_3D('',#32418,#16333,#16334);
#12977=AXIS2_PLACEMENT_3D('',#32419,#16335,#16336);
#12978=AXIS2_PLACEMENT_3D('',#32514,#16337,#16338);
#12979=AXIS2_PLACEMENT_3D('',#32639,#16339,#16340);
#12980=AXIS2_PLACEMENT_3D('',#37605,#16347,#16348);
#12981=AXIS2_PLACEMENT_3D('',#37606,#16349,#16350);
#12982=AXIS2_PLACEMENT_3D('',#37607,#16351,#16352);
#12983=AXIS2_PLACEMENT_3D('',#37608,#16353,#16354);
#12984=AXIS2_PLACEMENT_3D('',#37609,#16355,#16356);
#12985=AXIS2_PLACEMENT_3D('',#37610,#16357,#16358);
#12986=AXIS2_PLACEMENT_3D('',#37611,#16359,#16360);
#12987=AXIS2_PLACEMENT_3D('',#37612,#16361,#16362);
#12988=AXIS2_PLACEMENT_3D('',#37613,#16363,#16364);
#12989=AXIS2_PLACEMENT_3D('',#37614,#16365,#16366);
#12990=AXIS2_PLACEMENT_3D('',#37615,#16367,#16368);
#16276=DIRECTION('axis',(0.,0.,1.));
#16277=DIRECTION('refdir',(1.,0.,0.));
#16278=DIRECTION('center_axis',(0.,-1.,0.));
#16279=DIRECTION('ref_axis',(0.,0.,-1.));
#16280=DIRECTION('center_axis',(0.,1.,0.));
#16281=DIRECTION('ref_axis',(0.,0.,1.));
#16282=DIRECTION('',(0.,1.,0.));
#16283=DIRECTION('center_axis',(0.,-1.,0.));
#16284=DIRECTION('ref_axis',(0.,0.,1.));
#16285=DIRECTION('center_axis',(0.,-1.,0.));
#16286=DIRECTION('ref_axis',(0.,0.,1.));
#16287=DIRECTION('center_axis',(0.,-1.,0.));
#16288=DIRECTION('ref_axis',(0.,0.,1.));
#16289=DIRECTION('center_axis',(0.,-1.,0.));
#16290=DIRECTION('ref_axis',(0.,0.,1.));
#16291=DIRECTION('center_axis',(0.,-1.,0.));
#16292=DIRECTION('ref_axis',(0.,0.,1.));
#16293=DIRECTION('center_axis',(0.,-1.,0.));
#16294=DIRECTION('ref_axis',(0.,0.,1.));
#16295=DIRECTION('center_axis',(0.,-1.,0.));
#16296=DIRECTION('ref_axis',(2.66453528935155E-15,0.,1.));
#16297=DIRECTION('center_axis',(0.,-1.,0.));
#16298=DIRECTION('ref_axis',(-9.76996260157579E-15,0.,1.));
#16299=DIRECTION('',(0.,1.,0.));
#16300=DIRECTION('center_axis',(0.,-1.,0.));
#16301=DIRECTION('ref_axis',(0.,0.,-1.));
#16302=DIRECTION('center_axis',(0.,-1.,0.));
#16303=DIRECTION('ref_axis',(1.,0.,0.));
#16304=DIRECTION('center_axis',(1.,0.,1.2246462853756E-16));
#16305=DIRECTION('ref_axis',(-1.2246462853756E-16,0.,1.));
#16306=DIRECTION('center_axis',(0.,1.,0.));
#16307=DIRECTION('ref_axis',(0.,0.,-1.));
#16308=DIRECTION('center_axis',(0.,1.,0.));
#16309=DIRECTION('ref_axis',(0.,0.,1.));
#16310=DIRECTION('center_axis',(0.,-1.,0.));
#16311=DIRECTION('ref_axis',(0.,0.,-1.));
#16312=DIRECTION('',(0.,1.,0.));
#16313=DIRECTION('center_axis',(0.,1.,0.));
#16314=DIRECTION('ref_axis',(0.,0.,-1.));
#16315=DIRECTION('center_axis',(0.,-1.,0.));
#16316=DIRECTION('ref_axis',(0.,0.,-1.));
#16317=DIRECTION('center_axis',(0.,-1.,0.));
#16318=DIRECTION('ref_axis',(0.,0.,-1.));
#16319=DIRECTION('center_axis',(1.,0.,1.22464658788737E-16));
#16320=DIRECTION('ref_axis',(-1.22464658788737E-16,0.,1.));
#16321=DIRECTION('center_axis',(0.,1.,0.));
#16322=DIRECTION('ref_axis',(0.,0.,-1.));
#16323=DIRECTION('center_axis',(0.,-1.,0.));
#16324=DIRECTION('ref_axis',(0.,0.,-1.));
#16325=DIRECTION('',(0.,-1.,0.));
#16326=DIRECTION('center_axis',(0.,-1.,0.));
#16327=DIRECTION('ref_axis',(0.,0.,-1.));
#16328=DIRECTION('center_axis',(0.,-1.,0.));
#16329=DIRECTION('ref_axis',(0.,0.,-1.));
#16330=DIRECTION('',(-0.100145321866555,0.991509942423395,-0.0829394271972054));
#16331=DIRECTION('center_axis',(0.,1.,0.));
#16332=DIRECTION('ref_axis',(0.,0.,1.));
#16333=DIRECTION('center_axis',(0.,1.,0.));
#16334=DIRECTION('ref_axis',(0.,0.,1.));
#16335=DIRECTION('center_axis',(-1.,0.,1.22464701140385E-16));
#16336=DIRECTION('ref_axis',(-1.22464701140385E-16,0.,-1.));
#16337=DIRECTION('center_axis',(0.,-1.,0.));
#16338=DIRECTION('ref_axis',(-9.76996260157579E-15,0.,1.));
#16339=DIRECTION('center_axis',(0.,-1.,0.));
#16340=DIRECTION('ref_axis',(0.,0.,-1.));
#16341=DIRECTION('',(0.126213886040806,0.99150994242542,0.0312744151347175));
#16342=DIRECTION('',(0.0542417484749782,0.99150994242342,0.118177268532842));
#16343=DIRECTION('',(-0.0585755320417947,0.991509942423397,0.116090228363862));
#16344=DIRECTION('',(-0.127284242208166,0.991509942423416,0.0265848784275387));
#16345=DIRECTION('',(0.00240506843293452,0.9915099424234,-0.130008652486594));
#16346=DIRECTION('',(0.103144393148005,0.991509942423398,-0.0791787107603998));
#16347=DIRECTION('center_axis',(0.,1.,0.));
#16348=DIRECTION('ref_axis',(0.,0.,1.));
#16349=DIRECTION('center_axis',(0.,1.,0.));
#16350=DIRECTION('ref_axis',(0.,0.,1.));
#16351=DIRECTION('center_axis',(0.,-1.,0.));
#16352=DIRECTION('ref_axis',(0.,0.,-1.));
#16353=DIRECTION('center_axis',(0.,-1.,0.));
#16354=DIRECTION('ref_axis',(0.,0.,-1.));
#16355=DIRECTION('center_axis',(0.,-1.,0.));
#16356=DIRECTION('ref_axis',(0.,0.,-1.));
#16357=DIRECTION('center_axis',(0.,-1.,0.));
#16358=DIRECTION('ref_axis',(0.,0.,-1.));
#16359=DIRECTION('center_axis',(0.,-1.,0.));
#16360=DIRECTION('ref_axis',(0.,0.,-1.));
#16361=DIRECTION('center_axis',(0.,-1.,0.));
#16362=DIRECTION('ref_axis',(0.109251264469497,0.,0.994014165498569));
#16363=DIRECTION('center_axis',(0.,-1.,0.));
#16364=DIRECTION('ref_axis',(0.,0.,-1.));
#16365=DIRECTION('center_axis',(0.,-1.,0.));
#16366=DIRECTION('ref_axis',(0.,0.,-1.));
#16367=DIRECTION('center_axis',(0.,-1.,0.));
#16368=DIRECTION('ref_axis',(0.,0.,-1.));
#32195=CARTESIAN_POINT('',(0.,0.,0.));
#32196=CARTESIAN_POINT('Origin',(7.5111559719605E-6,20.2903503023534,4.07573877568452E-6));
#32197=CARTESIAN_POINT('',(7.51115596928158E-6,-3.14714969764662,21.8750040757388));
#32198=CARTESIAN_POINT('Origin',(7.5111559719605E-6,-3.14714969764662,4.07573877568452E-6));
#32199=CARTESIAN_POINT('',(7.51113043071691E-6,-0.359077263140675,21.8750040757388));
#32200=CARTESIAN_POINT('',(7.51115596928158E-6,20.2903503023534,21.8750040757388));
#32201=CARTESIAN_POINT('',(-11.6286532108092,17.7903562366901,18.528087484808));
#32202=CARTESIAN_POINT('Ctrl Pts',(7.51110489222162E-6,-0.359077263140676,
21.8750040757388));
#32203=CARTESIAN_POINT('Ctrl Pts',(-0.242521808837313,0.787240620602144,
21.8750040757382));
#32204=CARTESIAN_POINT('Ctrl Pts',(-0.54540759357386,1.9195211595413,21.8714101784102));
#32205=CARTESIAN_POINT('Ctrl Pts',(-1.59847036445218,5.0559408312384,21.8271017536525));
#32206=CARTESIAN_POINT('Ctrl Pts',(-2.48649791511479,6.94231008337416,21.7624093403727));
#32207=CARTESIAN_POINT('Ctrl Pts',(-4.68929447542434,10.5092773155408,21.3951090797112));
#32208=CARTESIAN_POINT('Ctrl Pts',(-5.95096816574499,12.119347275553,21.0995416323438));
#32209=CARTESIAN_POINT('Ctrl Pts',(-8.70650705890375,15.1447845037697,20.1220819188374));
#32210=CARTESIAN_POINT('Ctrl Pts',(-10.1763293042647,16.5261427053452,19.4396001110593));
#32211=CARTESIAN_POINT('Ctrl Pts',(-11.6286532108092,17.7903562366901,18.528087484808));
#32212=CARTESIAN_POINT('',(-21.6029109448944,17.7903503023534,3.43941378980876));
#32213=CARTESIAN_POINT('Origin',(7.5111559719605E-6,17.7903503023534,4.07573877568452E-6));
#32214=CARTESIAN_POINT('',(-16.8093026954431,-3.07550340054456,13.9986724319706));
#32215=CARTESIAN_POINT('Ctrl Pts',(-21.6029109448944,17.7903503023534,3.43941378980876));
#32216=CARTESIAN_POINT('Ctrl Pts',(-21.3273236992784,16.6048563822885,5.17037616111758));
#32217=CARTESIAN_POINT('Ctrl Pts',(-20.8613902773445,15.2608755267349,6.74246896531775));
#32218=CARTESIAN_POINT('Ctrl Pts',(-19.7942016810054,12.2596276657995,9.41879827256646));
#32219=CARTESIAN_POINT('Ctrl Pts',(-19.2123581961323,10.6436381400427,10.5083820514703));
#32220=CARTESIAN_POINT('Ctrl Pts',(-18.1533883573703,7.04932465914044,12.2482184494194));
#32221=CARTESIAN_POINT('Ctrl Pts',(-17.7057831864294,5.15107554627117,12.856864075177));
#32222=CARTESIAN_POINT('Ctrl Pts',(-17.0634858899474,1.10319626289942,13.6979815703421));
#32223=CARTESIAN_POINT('Ctrl Pts',(-16.8802985444201,-0.980646982039156,
13.9134220807907));
#32224=CARTESIAN_POINT('Ctrl Pts',(-16.8093024574423,-3.07550338138541,
13.9986727045614));
#32225=CARTESIAN_POINT('',(-21.7361818719648,17.7903503023534,2.46043007566383));
#32226=CARTESIAN_POINT('Ctrl Pts',(-16.809302912983,-3.07550344707786,13.9986721575575));
#32227=CARTESIAN_POINT('Ctrl Pts',(-16.9860508960446,-0.997639372661501,
13.7864368436865));
#32228=CARTESIAN_POINT('Ctrl Pts',(-17.2665397063309,1.04520175631502,13.4472040857416));
#32229=CARTESIAN_POINT('Ctrl Pts',(-18.0609524981394,5.05250922301929,12.3603585968672));
#32230=CARTESIAN_POINT('Ctrl Pts',(-18.5636987886872,6.93818763618362,11.6263456265167));
#32231=CARTESIAN_POINT('Ctrl Pts',(-19.6498492391718,10.5055771888037,9.67592682088231));
#32232=CARTESIAN_POINT('Ctrl Pts',(-20.2057076270334,12.116505550095,8.50500890855202));
#32233=CARTESIAN_POINT('Ctrl Pts',(-21.16013987792,15.143532030257,5.74031484751266));
#32234=CARTESIAN_POINT('Ctrl Pts',(-21.5432335765096,16.525560671386,4.16499696419982));
#32235=CARTESIAN_POINT('Ctrl Pts',(-21.7361818719648,17.7903503023534,2.46043007566384));
#32236=CARTESIAN_POINT('',(-16.1582306321435,17.7903503023534,-14.7454008052546));
#32237=CARTESIAN_POINT('Origin',(7.5111559719605E-6,17.7903503023534,4.07573877568452E-6));
#32238=CARTESIAN_POINT('',(-21.4250256124694,-3.07550340054456,-4.41401688263851));
#32239=CARTESIAN_POINT('Ctrl Pts',(-16.1582306321435,17.7903503023534,-14.7454008052546));
#32240=CARTESIAN_POINT('Ctrl Pts',(-17.3397256718364,16.6048563822885,-13.4507006345531));
#32241=CARTESIAN_POINT('Ctrl Pts',(-18.2783325826005,15.2608755267349,-12.1062353855568));
#32242=CARTESIAN_POINT('Ctrl Pts',(-19.7053898859821,12.2596276657995,-9.60320971372281));
#32243=CARTESIAN_POINT('Ctrl Pts',(-20.1944873080192,10.6436381400427,-8.46896178496286));
#32244=CARTESIAN_POINT('Ctrl Pts',(-20.8944892833356,7.04932465914048,-6.55625557501076));
#32245=CARTESIAN_POINT('Ctrl Pts',(-21.0912703358785,5.15107554627125,-5.8268194200479));
#32246=CARTESIAN_POINT('Ctrl Pts',(-21.3484166599352,1.10319626289929,-4.8002229921537));
#32247=CARTESIAN_POINT('Ctrl Pts',(-21.402639391837,-0.980646982039869,
-4.5226763970588));
#32248=CARTESIAN_POINT('Ctrl Pts',(-21.4250256771985,-3.07550338138541,
-4.41401652660439));
#32249=CARTESIAN_POINT('',(-15.4759234075142,17.7903503023534,-15.4599825736911));
#32250=CARTESIAN_POINT('Ctrl Pts',(-21.4250255335586,-3.07550344707786,
-4.41401722381183));
#32251=CARTESIAN_POINT('Ctrl Pts',(-21.3692938484207,-0.997639372661258,
-4.68453091522497));
#32252=CARTESIAN_POINT('Ctrl Pts',(-21.2789529111239,1.04520175631505,-5.11533406262186));
#32253=CARTESIAN_POINT('Ctrl Pts',(-20.9245311655024,5.05250922301919,-6.41406807184237));
#32254=CARTESIAN_POINT('Ctrl Pts',(-20.6641139018212,6.93818763618362,-7.26478055093226));
#32255=CARTESIAN_POINT('Ctrl Pts',(-19.81641880474,10.5055771888037,-9.33003340248447));
#32256=CARTESIAN_POINT('Ctrl Pts',(-19.2475303536038,12.116505550095,-10.4946763670602));
#32257=CARTESIAN_POINT('Ctrl Pts',(-17.6810842722838,15.1435320302569,-12.9646401010037));
#32258=CARTESIAN_POINT('Ctrl Pts',(-16.6883061704418,16.5255606713859,-14.2463494502274));
#32259=CARTESIAN_POINT('Ctrl Pts',(-15.4759234075142,17.7903503023534,-15.4599825736911));
#32260=CARTESIAN_POINT('',(7.51115596928158E-6,17.7903503023534,-21.8749959242612));
#32261=CARTESIAN_POINT('Origin',(7.5111559719605E-6,17.7903503023534,4.07573877568452E-6));
#32262=CARTESIAN_POINT('',(1.45393257050235,17.7903503023534,-21.8266247734858));
#32263=CARTESIAN_POINT('Origin',(7.5111559719605E-6,17.7903503023534,4.07573877568452E-6));
#32264=CARTESIAN_POINT('',(-9.90726159778959,-3.07550341763295,-19.5028583812017));
#32265=CARTESIAN_POINT('Ctrl Pts',(1.45393257050235,17.7903503023534,-21.8266247734858));
#32266=CARTESIAN_POINT('Ctrl Pts',(-0.42071722963709,16.5196076224518,-21.9514997755189));
#32267=CARTESIAN_POINT('Ctrl Pts',(-2.16453839481852,15.0681198554842,-21.822133979092));
#32268=CARTESIAN_POINT('Ctrl Pts',(-5.15083863820302,11.8037205632591,-21.3119549809142));
#32269=CARTESIAN_POINT('Ctrl Pts',(-6.3697426145343,10.0441260470548,-20.9514582684722));
#32270=CARTESIAN_POINT('Ctrl Pts',(-8.15807676202854,6.37804252407538,-20.316195099095));
#32271=CARTESIAN_POINT('Ctrl Pts',(-8.7555204640488,4.59032766603492,-20.0515884547815));
#32272=CARTESIAN_POINT('Ctrl Pts',(-9.59144327553473,0.814270441473194,
-19.6655393452124));
#32273=CARTESIAN_POINT('Ctrl Pts',(-9.8152351985608,-1.12645709600235,-19.5496069154558));
#32274=CARTESIAN_POINT('Ctrl Pts',(-9.90726191550005,-3.07550338999529,
-19.5028582143879));
#32275=CARTESIAN_POINT('',(2.4380266901546,17.7903503023534,-21.7387099497696));
#32276=CARTESIAN_POINT('Ctrl Pts',(2.4380266901546,17.7903503023534,-21.7387099497696));
#32277=CARTESIAN_POINT('Ctrl Pts',(0.519424066437449,16.366911361741,-21.9538832110771));
#32278=CARTESIAN_POINT('Ctrl Pts',(-1.29094448071633,14.7970175900028,-21.8969955147474));
#32279=CARTESIAN_POINT('Ctrl Pts',(-4.46152970952729,11.3236494616448,-21.4731858316244));
#32280=CARTESIAN_POINT('Ctrl Pts',(-5.790993610098,9.47257185931529,-21.12458283065));
#32281=CARTESIAN_POINT('Ctrl Pts',(-7.71013039377804,5.79264830253153,-20.4907332313965));
#32282=CARTESIAN_POINT('Ctrl Pts',(-8.36432873407734,4.10230776867177,-20.2201250966576));
#32283=CARTESIAN_POINT('Ctrl Pts',(-9.35970303244591,0.555960676466445,
-19.7788756473871));
#32284=CARTESIAN_POINT('Ctrl Pts',(-9.69063212779356,-1.24753824725553,
-19.6129040870217));
#32285=CARTESIAN_POINT('Ctrl Pts',(-9.90726128043683,-3.07550344707786,
-19.502858536994));
#32286=CARTESIAN_POINT('',(17.9712605487941,17.7903503023534,-12.4719520361622));
#32287=CARTESIAN_POINT('Origin',(7.5111559719605E-6,17.7903503023534,4.07573877568452E-6));
#32288=CARTESIAN_POINT('',(9.07087812914772,-3.07550340054456,-19.9056466697429));
#32289=CARTESIAN_POINT('Ctrl Pts',(17.9712652714714,17.790355904801,-12.4719452310979));
#32290=CARTESIAN_POINT('Ctrl Pts',(16.9719333168451,16.6048619847361,-13.9119156145767));
#32291=CARTESIAN_POINT('Ctrl Pts',(15.8700315823639,15.2608755267349,-15.1261681583902));
#32292=CARTESIAN_POINT('Ctrl Pts',(13.747312113943,12.2596276657995,-17.074421765953));
#32293=CARTESIAN_POINT('Ctrl Pts',(12.7503365640078,10.6436381400426,-17.8036504029188));
#32294=CARTESIAN_POINT('Ctrl Pts',(11.0413509854407,7.04932465914046,-18.9117190394597));
#32295=CARTESIAN_POINT('Ctrl Pts',(10.3739912214096,5.1510755462712,-19.2658811946362));
#32296=CARTESIAN_POINT('Ctrl Pts',(9.43035414950194,1.10319626289946,-19.7450195194052));
#32297=CARTESIAN_POINT('Ctrl Pts',(9.17183191995736,-0.980646982038627,
-19.859642701768));
#32298=CARTESIAN_POINT('Ctrl Pts',(9.07087779644369,-3.07550338138541,-19.9056468120741));
#32299=CARTESIAN_POINT('',(18.5160986195094,17.7903503023534,-11.6477422756871));
#32300=CARTESIAN_POINT('Ctrl Pts',(9.0708784442078,-3.07550344707787,-19.9056465168923));
#32301=CARTESIAN_POINT('Ctrl Pts',(9.32220832596597,-0.997639372661295,
-19.7911171821972));
#32302=CARTESIAN_POINT('Ctrl Pts',(9.72210758927721,1.04520175631505,-19.6071785621038));
#32303=CARTESIAN_POINT('Ctrl Pts',(10.909413367516,5.05250922301937,-18.9726474049206));
#32304=CARTESIAN_POINT('Ctrl Pts',(11.6808484158895,6.93818763618365,-18.5294580103685));
#32305=CARTESIAN_POINT('Ctrl Pts',(13.5056911618681,10.5055771888038,-17.243454405821));
#32306=CARTESIAN_POINT('Ctrl Pts',(14.5145445062954,12.1165055500951,-16.4296717356873));
#32307=CARTESIAN_POINT('Ctrl Pts',(16.5740140475861,15.143532030257,-14.3528810911652));
#32308=CARTESIAN_POINT('Ctrl Pts',(17.6026743570154,16.5255606713859,-13.0997868476268));
#32309=CARTESIAN_POINT('Ctrl Pts',(18.5160986195094,17.7903503023534,-11.6477422756871));
#32310=CARTESIAN_POINT('',(20.9558684429898,17.7903503023534,6.27435803496356));
#32311=CARTESIAN_POINT('Origin',(7.5111559719605E-6,17.7903503023534,4.07573877568452E-6));
#32312=CARTESIAN_POINT('',(21.2184672672846,-3.07550340054455,-5.31907394089049));
#32313=CARTESIAN_POINT('Ctrl Pts',(20.9558684429898,17.7903503023534,6.27435803496357));
#32314=CARTESIAN_POINT('Ctrl Pts',(21.4586093402341,16.6048563822885,4.59524200232282));
#32315=CARTESIAN_POINT('Ctrl Pts',(21.7209233366826,15.260875526735,2.97667439299652));
#32316=CARTESIAN_POINT('Ctrl Pts',(21.9206354021396,12.2596276657995,0.102349228387359));
#32317=CARTESIAN_POINT('Ctrl Pts',(21.8691652203497,10.6436381400426,-1.13178426217439));
#32318=CARTESIAN_POINT('Ctrl Pts',(21.6699530853725,7.04932465914044,-3.15879248522481));
#32319=CARTESIAN_POINT('Ctrl Pts',(21.530756201144,5.15107554627118,-3.9013718508336));
#32320=CARTESIAN_POINT('Ctrl Pts',(21.3170135369151,1.10319626289944,-4.9378748808481));
#32321=CARTESIAN_POINT('Ctrl Pts',(21.2454435758322,-0.980646982038895,
-5.21146208408366));
#32322=CARTESIAN_POINT('Ctrl Pts',(21.2184671711261,-3.07550338138541,-5.31907428975103));
#32323=CARTESIAN_POINT('',(20.6511762848484,17.7903503023534,7.2142159717446));
#32324=CARTESIAN_POINT('Ctrl Pts',(21.218467344218,-3.07550344707786,-5.31907359926584));
#32325=CARTESIAN_POINT('Ctrl Pts',(21.2856263228658,-0.997639372661455,
-5.0511681130263));
#32326=CARTESIAN_POINT('Ctrl Pts',(21.3911504312805,1.045201756315,-4.62383042535759));
#32327=CARTESIAN_POINT('Ctrl Pts',(21.6353270404075,5.05250922301931,-3.29993368314891));
#32328=CARTESIAN_POINT('Ctrl Pts',(21.769809504508,6.93818763618363,-2.42047740785612));
#32329=CARTESIAN_POINT('Ctrl Pts',(21.902142242019,10.5055771888038,-0.191947765907667));
#32330=CARTESIAN_POINT('Ctrl Pts',(21.8949111024431,12.116505550095,1.10419073571645));
#32331=CARTESIAN_POINT('Ctrl Pts',(21.5552690502941,15.143532030257,4.00920664773668));
#32332=CARTESIAN_POINT('Ctrl Pts',(21.2169197327024,16.5255606713859,5.59473714402792));
#32333=CARTESIAN_POINT('Ctrl Pts',(20.6511762848484,17.7903503023534,7.2142159717446));
#32334=CARTESIAN_POINT('',(8.16028563385461,17.7903503023534,20.2959516012968));
#32335=CARTESIAN_POINT('Origin',(7.5111559719605E-6,17.7903503023534,4.07573877568452E-6));
#32336=CARTESIAN_POINT('',(17.3881234313567,-3.07550340054456,13.2728730239015));
#32337=CARTESIAN_POINT('Ctrl Pts',(8.16028563385462,17.7903503023534,20.2959516012968));
#32338=CARTESIAN_POINT('Ctrl Pts',(9.78652523329912,16.6048563822885,19.6420985397976));
#32339=CARTESIAN_POINT('Ctrl Pts',(11.2155224484438,15.2608755267349,18.8380234824792));
#32340=CARTESIAN_POINT('Ctrl Pts',(13.587278789106,12.2596276657994,17.2020522353224));
#32341=CARTESIAN_POINT('Ctrl Pts',(14.5200720721495,10.6436381400426,16.3923415812932));
#32342=CARTESIAN_POINT('Ctrl Pts',(15.980644181587,7.0493246591405,14.9727723071226));
#32343=CARTESIAN_POINT('Ctrl Pts',(16.4744282700841,5.15107554627125,14.4009531392434));
#32344=CARTESIAN_POINT('Ctrl Pts',(17.1515325992541,1.1031962628995,13.587593326393));
#32345=CARTESIAN_POINT('Ctrl Pts',(17.3208085470894,-0.980646982038474,
13.3610588464829));
#32346=CARTESIAN_POINT('Ctrl Pts',(17.3881236441529,-3.07550338138541,13.2728727312108));
#32347=CARTESIAN_POINT('',(7.23550265652423,17.7903503023534,20.6437255183797));
#32348=CARTESIAN_POINT('Ctrl Pts',(17.3881232122309,-3.07550344707786,13.27287329705));
#32349=CARTESIAN_POINT('Ctrl Pts',(17.2205392070531,-0.99763937266114,13.4924166394196));
#32350=CARTESIAN_POINT('Ctrl Pts',(16.9522263546354,1.04520175631507,13.8413593997489));
#32351=CARTESIAN_POINT('Ctrl Pts',(16.069403827683,5.05250922301932,14.8577004775278));
#32352=CARTESIAN_POINT('Ctrl Pts',(15.4656656691005,6.93818763618363,15.5111751206272));
#32353=CARTESIAN_POINT('Ctrl Pts',(13.8058391477021,10.5055771888038,17.0041025258692));
#32354=CARTESIAN_POINT('Ctrl Pts',(12.7879687197121,12.116505550095,17.8065781308538));
#32355=CARTESIAN_POINT('Ctrl Pts',(10.3049724668269,15.143532030257,19.3522830770956));
#32356=CARTESIAN_POINT('Ctrl Pts',(8.85439745942891,16.5255606713859,20.0763130235044));
#32357=CARTESIAN_POINT('Ctrl Pts',(7.23550265652423,17.7903503023534,20.6437255183797));
#32358=CARTESIAN_POINT('',(7.51115596928158E-6,17.7903503023534,21.8750040757388));
#32359=CARTESIAN_POINT('Origin',(7.5111559719605E-6,17.7903503023534,4.07573877568452E-6));
#32360=CARTESIAN_POINT('',(7.51080208344241E-6,1.03580637516255,21.8750040757388));
#32361=CARTESIAN_POINT('',(7.51115596928158E-6,20.2903503023534,21.8750040757388));
#32362=CARTESIAN_POINT('',(0.464173657934616,-3.07550341763295,21.8700789498582));
#32363=CARTESIAN_POINT('Ctrl Pts',(7.51044819783525E-6,1.03580637516255,
21.8750040757388));
#32364=CARTESIAN_POINT('Ctrl Pts',(0.243703115036094,-0.321768697993278,
21.8750040757467));
#32365=CARTESIAN_POINT('Ctrl Pts',(0.391146320999169,-1.69625048081135,
21.8716288639911));
#32366=CARTESIAN_POINT('Ctrl Pts',(0.464174017015567,-3.0755033986066,21.8700789374039));
#32367=CARTESIAN_POINT('Ctrl Pts',(0.464173305560506,-3.07550345570599,
21.8700789525037));
#32368=CARTESIAN_POINT('Ctrl Pts',(0.342862298231604,-2.16265365777846,
21.8726536313927));
#32369=CARTESIAN_POINT('Ctrl Pts',(0.189893689499557,-1.25657667567048,
21.8750040757392));
#32370=CARTESIAN_POINT('Ctrl Pts',(7.51110489346195E-6,-0.359077263140675,
21.8750040757388));
#32371=CARTESIAN_POINT('Origin',(7.5111559719605E-6,13.1028503023534,4.07573877568452E-6));
#32372=CARTESIAN_POINT('',(7.51115597150125E-6,13.1028503023534,3.75000407573878));
#32373=CARTESIAN_POINT('Origin',(7.5111559719605E-6,13.1028503023534,4.07573877568452E-6));
#32374=CARTESIAN_POINT('',(7.51115597119509E-6,15.6028503023534,6.25000407573878));
#32375=CARTESIAN_POINT('Origin',(7.51115597119509E-6,13.1028503023534,6.25000407573878));
#32376=CARTESIAN_POINT('Origin',(7.5111559719605E-6,15.6028503023534,4.07573877568452E-6));
#32377=CARTESIAN_POINT('Origin',(7.5111559719605E-6,13.1028503023534,4.07573877568452E-6));
#32378=CARTESIAN_POINT('',(7.51115597173087E-6,13.1028503023534,-1.87499592426122));
#32379=CARTESIAN_POINT('Origin',(7.5111559719605E-6,13.1028503023534,4.07573877568452E-6));
#32380=CARTESIAN_POINT('',(7.51115597173087E-6,15.6028503023534,-1.87499592426122));
#32381=CARTESIAN_POINT('',(7.51115597173087E-6,13.1028503023534,-1.87499592426122));
#32382=CARTESIAN_POINT('Origin',(7.5111559719605E-6,15.6028503023534,4.07573877568452E-6));
#32383=CARTESIAN_POINT('Origin',(7.5111559719605E-6,14.3528503023534,4.07573877568452E-6));
#32384=CARTESIAN_POINT('',(7.51115596966429E-6,15.6028503023534,18.7500040757388));
#32385=CARTESIAN_POINT('Origin',(7.5111559719605E-6,15.6028503023534,4.07573877568452E-6));
#32386=CARTESIAN_POINT('',(7.5111559695112E-6,14.3528503023534,20.0000040757388));
#32387=CARTESIAN_POINT('Origin',(7.51115596966428E-6,14.3528503023534,18.7500040757388));
#32388=CARTESIAN_POINT('Origin',(7.5111559719605E-6,14.3528503023534,4.07573877568452E-6));
#32389=CARTESIAN_POINT('Origin',(7.5111559719605E-6,15.6028503023534,4.07573877568452E-6));
#32390=CARTESIAN_POINT('',(7.5111559695112E-6,-3.14714969764662,20.0000040757388));
#32391=CARTESIAN_POINT('',(7.5111559695112E-6,15.6028503023534,20.0000040757388));
#32392=CARTESIAN_POINT('Origin',(7.5111559719605E-6,-3.14714969764662,4.07573877568452E-6));
#32393=CARTESIAN_POINT('Origin',(7.5111559719605E-6,21.2397676607012,4.07573877568452E-6));
#32394=CARTESIAN_POINT('',(29.890987486445,20.7105311502984,-36.1080966928894));
#32395=CARTESIAN_POINT('',(-0.621426586513352,-3.27137103605589,-46.8708765192191));
#32396=CARTESIAN_POINT('Ctrl Pts',(-0.621426973050868,-3.27137033355074,
-46.8708764811895));
#32397=CARTESIAN_POINT('Ctrl Pts',(1.22198947607096,-0.293500394512695,
-46.8953172968223));
#32398=CARTESIAN_POINT('Ctrl Pts',(3.47149086853713,2.39667808539656,-46.812476661266));
#32399=CARTESIAN_POINT('Ctrl Pts',(8.47386002556298,7.40863725852386,-46.1734052030165));
#32400=CARTESIAN_POINT('Ctrl Pts',(11.2378060047234,9.72308571822484,-45.603191808413));
#32401=CARTESIAN_POINT('Ctrl Pts',(16.8130139628313,13.8834472854297,-43.8519117248611));
#32402=CARTESIAN_POINT('Ctrl Pts',(19.6837688691993,15.782750805847,-42.6607369480052));
#32403=CARTESIAN_POINT('Ctrl Pts',(24.9813517355624,18.7788815506097,-39.7661777334129));
#32404=CARTESIAN_POINT('Ctrl Pts',(27.4992571672096,19.9779504583433,-38.0880170308874));
#32405=CARTESIAN_POINT('Ctrl Pts',(29.8909874864411,20.7105311502992,-36.1080966928852));
#32406=CARTESIAN_POINT('',(29.906901044747,20.5529756002067,-36.0949172314265));
#32407=CARTESIAN_POINT('',(29.906901044747,20.5529756002067,-36.0949172314265));
#32408=CARTESIAN_POINT('Ctrl Pts',(29.9069010447472,20.5529756002057,-36.0949172314263));
#32409=CARTESIAN_POINT('Ctrl Pts',(27.4917467114803,19.3280006163688,-38.0960232290689));
#32410=CARTESIAN_POINT('Ctrl Pts',(24.9374114080822,17.7790790293585,-39.7993592079281));
#32411=CARTESIAN_POINT('Ctrl Pts',(19.584902818122,14.2745254800632,-42.7044404021991));
#32412=CARTESIAN_POINT('Ctrl Pts',(16.7183127703354,12.2572382417917,-43.8921366201915));
#32413=CARTESIAN_POINT('Ctrl Pts',(8.45552582412058,6.00731091640547,-46.4561374167343));
#32414=CARTESIAN_POINT('Ctrl Pts',(3.38588451053795,1.62140339199547,-46.9240070793036));
#32415=CARTESIAN_POINT('Ctrl Pts',(-0.621426068179982,-3.27137132078905,
-46.8708764931867));
#32416=CARTESIAN_POINT('Origin',(7.5111559719605E-6,17.7903503023534,4.07573877568452E-6));
#32417=CARTESIAN_POINT('',(7.51115596958774E-6,20.2903503023534,-19.3749959242612));
#32418=CARTESIAN_POINT('Origin',(7.5111559719605E-6,20.2903503023534,4.07573877568452E-6));
#32419=CARTESIAN_POINT('Origin',(7.51115596958774E-6,17.7903503023534,-19.3749959242612));
#32420=CARTESIAN_POINT('',(-12.693647630517,19.9464420456703,-16.2756753502908));
#32421=CARTESIAN_POINT('Ctrl Pts',(-12.6936476305231,19.9464420456617,-16.2756753502661));
#32422=CARTESIAN_POINT('Ctrl Pts',(-12.8235252273233,19.8728182056928,-16.3334681308482));
#32423=CARTESIAN_POINT('Ctrl Pts',(-12.9581519320085,19.7918094976896,-16.371317941139));
#32424=CARTESIAN_POINT('Ctrl Pts',(-13.2224716578103,19.625306229008,-16.4147366199682));
#32425=CARTESIAN_POINT('Ctrl Pts',(-13.3532075689092,19.5393897285476,-16.4214641365178));
#32426=CARTESIAN_POINT('Ctrl Pts',(-13.7362414247294,19.2783123963091,-16.407438160254));
#32427=CARTESIAN_POINT('Ctrl Pts',(-13.987254982389,19.0945659360765,-16.3530231613382));
#32428=CARTESIAN_POINT('Ctrl Pts',(-14.6625794013184,18.5673472018936,-16.1138738953652));
#32429=CARTESIAN_POINT('Ctrl Pts',(-15.0965980929232,18.1860724615002,-15.8396990959256));
#32430=CARTESIAN_POINT('Ctrl Pts',(-15.4759234075142,17.7903503023534,-15.4599825736911));
#32431=CARTESIAN_POINT('',(-12.5441843191278,20.1925493450899,-15.6634703684439));
#32432=CARTESIAN_POINT('Ctrl Pts',(-12.5441843191278,20.1925493450898,-15.6634703684439));
#32433=CARTESIAN_POINT('Ctrl Pts',(-12.5734306475263,20.1623540838438,-15.774258024762));
#32434=CARTESIAN_POINT('Ctrl Pts',(-12.6011389695311,20.1252944701824,-15.8835795820431));
#32435=CARTESIAN_POINT('Ctrl Pts',(-12.6271510859688,20.0815864671199,-15.9906280584417));
#32436=CARTESIAN_POINT('Ctrl Pts',(-12.6507434848167,20.0419443009946,-16.0877185953578));
#32437=CARTESIAN_POINT('Ctrl Pts',(-12.6729413900718,19.9968331833498,-16.1829393382146));
#32438=CARTESIAN_POINT('Ctrl Pts',(-12.6936476305122,19.946442045657,-16.2756753502846));
#32439=CARTESIAN_POINT('Ctrl Pts',(-16.1582306321435,17.7903503023534,-14.7454008052546));
#32440=CARTESIAN_POINT('Ctrl Pts',(-15.9327118880776,18.0166323356832,-14.9925276628623));
#32441=CARTESIAN_POINT('Ctrl Pts',(-15.6779879864518,18.244370505181,-15.2146917900135));
#32442=CARTESIAN_POINT('Ctrl Pts',(-15.1369202951668,18.6805240933459,-15.5819230082715));
#32443=CARTESIAN_POINT('Ctrl Pts',(-14.8487394640944,18.8925325606821,-15.7331109967917));
#32444=CARTESIAN_POINT('Ctrl Pts',(-14.163605905897,19.353358815909,-15.9788255101609));
#32445=CARTESIAN_POINT('Ctrl Pts',(-13.7876875418779,19.5776706634899,-16.0374669418776));
#32446=CARTESIAN_POINT('Ctrl Pts',(-13.260925054244,19.8635098001506,-16.0019414049453));
#32447=CARTESIAN_POINT('Ctrl Pts',(-13.066900930548,19.9622625901948,-15.9623273700109));
#32448=CARTESIAN_POINT('Ctrl Pts',(-12.7633032903853,20.1031710857547,-15.8284713051116));
#32449=CARTESIAN_POINT('Ctrl Pts',(-12.6477215025671,20.1529191619863,-15.7566974006731));
#32450=CARTESIAN_POINT('Ctrl Pts',(-12.5441843191278,20.1925493450899,-15.6634703684439));
#32451=CARTESIAN_POINT('',(-20.6391955918159,19.9464420456703,-0.223416847360512));
#32452=CARTESIAN_POINT('Ctrl Pts',(-20.6391955918004,19.9464420456617,-0.223416847340363));
#32453=CARTESIAN_POINT('Ctrl Pts',(-20.7653571642138,19.8728182056928,-0.157907662608692));
#32454=CARTESIAN_POINT('Ctrl Pts',(-20.8788877149336,19.7918094976896,-0.0762512372233672));
#32455=CARTESIAN_POINT('Ctrl Pts',(-21.0776344584369,19.625306229008,0.103331142385521));
#32456=CARTESIAN_POINT('Ctrl Pts',(-21.1644067499811,19.5393897285476,0.201350055611236));
#32457=CARTESIAN_POINT('Ctrl Pts',(-21.3922585030362,19.2783123963091,0.509563036104214));
#32458=CARTESIAN_POINT('Ctrl Pts',(-21.5062195370944,19.0945659360766,0.739740534900876));
#32459=CARTESIAN_POINT('Ctrl Pts',(-21.7403030000965,18.5673472018931,1.41683755495611));
#32460=CARTESIAN_POINT('Ctrl Pts',(-21.7965507382266,18.1860724614997,1.92711222340975));
#32461=CARTESIAN_POINT('Ctrl Pts',(-21.7361818719648,17.7903503023534,2.46043007566384));
#32462=CARTESIAN_POINT('',(-20.067365612881,20.1925493450899,0.0414315931501207));
#32463=CARTESIAN_POINT('Ctrl Pts',(-20.067365612881,20.1925493450898,0.0414315931501189));
#32464=CARTESIAN_POINT('Ctrl Pts',(-20.1722176779583,20.1623540838436,-0.00477768044781249));
#32465=CARTESIAN_POINT('Ctrl Pts',(-20.2749645693503,20.1252944701819,-0.0512753180664436));
#32466=CARTESIAN_POINT('Ctrl Pts',(-20.3748767276733,20.0815864671191,-0.0976818598491867));
#32467=CARTESIAN_POINT('Ctrl Pts',(-20.4654947861664,20.0419443009939,-0.139771539306826));
#32468=CARTESIAN_POINT('Ctrl Pts',(-20.5537815282644,19.9968331833494,-0.181785680229823));
#32469=CARTESIAN_POINT('Ctrl Pts',(-20.6391955918081,19.946442045657,-0.223416847360427));
#32470=CARTESIAN_POINT('Ctrl Pts',(-21.6029109448944,17.7903503023534,3.43941378980876));
#32471=CARTESIAN_POINT('Ctrl Pts',(-21.6555138652825,18.0166323356831,3.10901506032762));
#32472=CARTESIAN_POINT('Ctrl Pts',(-21.6703910192109,18.244370505181,2.7713468270818));
#32473=CARTESIAN_POINT('Ctrl Pts',(-21.6201537593587,18.6805240933459,2.11935815238101));
#32474=CARTESIAN_POINT('Ctrl Pts',(-21.55867947929,18.8925325606821,1.79978513699883));
#32475=CARTESIAN_POINT('Ctrl Pts',(-21.3236130350936,19.3533588159098,1.11092565824911));
#32476=CARTESIAN_POINT('Ctrl Pts',(-21.1350794862891,19.5776706634905,0.780458511779776));
#32477=CARTESIAN_POINT('Ctrl Pts',(-20.7788734640431,19.8635098001506,0.390768825148143));
#32478=CARTESIAN_POINT('Ctrl Pts',(-20.6269299019448,19.9622625901948,0.263773603676359));
#32479=CARTESIAN_POINT('Ctrl Pts',(-20.3329869837774,20.1031710857547,0.109869301975848));
#32480=CARTESIAN_POINT('Ctrl Pts',(-20.2048078196825,20.1529191619863,0.0642541189165845));
#32481=CARTESIAN_POINT('Ctrl Pts',(-20.067365612881,20.1925493450898,0.0414315931501027));
#32482=CARTESIAN_POINT('',(-13.0430026535592,19.9464420456703,15.9970821676198));
#32483=CARTESIAN_POINT('Ctrl Pts',(-13.0430026535338,19.9464420456617,15.9970821676202));
#32484=CARTESIAN_POINT('Ctrl Pts',(-13.0704465353675,19.872816673671,16.1365664678557));
#32485=CARTESIAN_POINT('Ctrl Pts',(-13.0773897151475,19.7918112588121,16.2762344448439));
#32486=CARTESIAN_POINT('Ctrl Pts',(-13.0609029504193,19.625306229008,16.5435915160662));
#32487=CARTESIAN_POINT('Ctrl Pts',(-13.0383703170438,19.5393897285476,16.6725466181869));
#32488=CARTESIAN_POINT('Ctrl Pts',(-12.9394629499546,19.2783123963091,17.0428559421987));
#32489=CARTESIAN_POINT('Ctrl Pts',(-12.8305564773841,19.0945659360765,17.2754675895172));
#32490=CARTESIAN_POINT('Ctrl Pts',(-12.4471293623855,18.5673472018934,17.8806444972902));
#32491=CARTESIAN_POINT('Ctrl Pts',(-12.0832504529845,18.1860724615001,18.2427718017058));
#32492=CARTESIAN_POINT('Ctrl Pts',(-11.6286463934656,17.7903503023534,18.5280917635313));
#32493=CARTESIAN_POINT('',(-12.4794056444224,20.1925493450899,15.715137789166));
#32494=CARTESIAN_POINT('Ctrl Pts',(-12.4794056444224,20.1925493450898,15.715137789166));
#32495=CARTESIAN_POINT('Ctrl Pts',(-12.5809077025813,20.162354083844,15.7683034238049));
#32496=CARTESIAN_POINT('Ctrl Pts',(-12.6813226584862,20.125294470183,15.8196433753545));
#32497=CARTESIAN_POINT('Ctrl Pts',(-12.7798989656392,20.081586467121,15.868823840671));
#32498=CARTESIAN_POINT('Ctrl Pts',(-12.8693054374623,20.0419443009953,15.9134294057765));
#32499=CARTESIAN_POINT('Ctrl Pts',(-12.9571992988835,19.9968331833502,15.9562593718345));
#32500=CARTESIAN_POINT('Ctrl Pts',(-13.0430026535542,19.946442045657,15.9970821676137));
#32501=CARTESIAN_POINT('',(-10.7801530410109,17.7903503023534,19.0342827190051));
#32502=CARTESIAN_POINT('Ctrl Pts',(-10.7801530410109,17.7903503023534,19.0342827190051));
#32503=CARTESIAN_POINT('Ctrl Pts',(-11.0712665538967,18.0166323356832,18.8694090998557));
#32504=CARTESIAN_POINT('Ctrl Pts',(-11.3445419630327,18.244370505181,18.6705078273261));
#32505=CARTESIAN_POINT('Ctrl Pts',(-11.8229648159352,18.6805240933458,18.2247224663774));
#32506=CARTESIAN_POINT('Ctrl Pts',(-12.0344884736088,18.8925325606821,17.9774094228175));
#32507=CARTESIAN_POINT('Ctrl Pts',(-12.4264989703763,19.3533588159099,17.3641302163587));
#32508=CARTESIAN_POINT('Ctrl Pts',(-12.5673198444194,19.5776706634906,17.0106858567289));
#32509=CARTESIAN_POINT('Ctrl Pts',(-12.6499006875901,19.8635098001506,16.4892252287881));
#32510=CARTESIAN_POINT('Ctrl Pts',(-12.6544542884334,19.9622625901948,16.2912507429088));
#32511=CARTESIAN_POINT('Ctrl Pts',(-12.5915111049841,20.1031710857547,15.9654791528645));
#32512=CARTESIAN_POINT('Ctrl Pts',(-12.5472560895544,20.1529191619863,15.8368240455314));
#32513=CARTESIAN_POINT('Ctrl Pts',(-12.4794056444224,20.1925493450899,15.715137789166));
#32514=CARTESIAN_POINT('Origin',(7.5111559719605E-6,17.7903503023534,4.07573877568452E-6));
#32515=CARTESIAN_POINT('',(4.37484296764849,19.9464420456703,20.1714550984892));
#32516=CARTESIAN_POINT('Ctrl Pts',(4.37484296766468,19.9464420456617,20.1714550984696));
#32517=CARTESIAN_POINT('Ctrl Pts',(4.46678329128665,19.8728182056928,20.2798763718909));
#32518=CARTESIAN_POINT('Ctrl Pts',(4.57165534378247,19.7918094976897,20.3723902106327));
#32519=CARTESIAN_POINT('Ctrl Pts',(4.79096052918446,19.625306229008,20.5261931194967));
#32520=CARTESIAN_POINT('Ctrl Pts',(4.90583055496595,19.5393897285475,20.5889785884108));
#32521=CARTESIAN_POINT('Ctrl Pts',(5.2570177774387,19.2783123963091,20.742533782027));
#32522=CARTESIAN_POINT('Ctrl Pts',(5.50678296150517,19.0945659360764,20.8024182630235));
#32523=CARTESIAN_POINT('Ctrl Pts',(6.21899221642201,18.5673472018938,20.8799645036025));
#32524=CARTESIAN_POINT('Ctrl Pts',(6.72898953279836,18.1860724615004,20.8212551977046));
#32525=CARTESIAN_POINT('Ctrl Pts',(7.23550265652423,17.7903503023534,20.6437255183797));
#32526=CARTESIAN_POINT('',(4.50580696382332,20.1925493450899,19.5550277686639));
#32527=CARTESIAN_POINT('Ctrl Pts',(4.50580696382332,20.1925493450898,19.5550277686639));
#32528=CARTESIAN_POINT('Ctrl Pts',(4.48408803263945,20.1623540838438,19.6675335042753));
#32529=CARTESIAN_POINT('Ctrl Pts',(4.46161952210836,20.1252944701825,19.7780510143322));
#32530=CARTESIAN_POINT('Ctrl Pts',(4.43860903600032,20.0815864671201,19.885784593266));
#32531=CARTESIAN_POINT('Ctrl Pts',(4.41773904769133,20.0419443009947,19.9834965026223));
#32532=CARTESIAN_POINT('Ctrl Pts',(4.3964239373066,19.9968331833498,20.0789187376476));
#32533=CARTESIAN_POINT('Ctrl Pts',(4.37484296764684,19.946442045657,20.1714550984815));
#32534=CARTESIAN_POINT('Ctrl Pts',(8.16028563385462,17.7903503023534,20.2959516012968));
#32535=CARTESIAN_POINT('Ctrl Pts',(7.84987594130768,18.0166323356831,20.4207562905075));
#32536=CARTESIAN_POINT('Ctrl Pts',(7.52398423384595,18.244370505181,20.5103986937555));
#32537=CARTESIAN_POINT('Ctrl Pts',(6.87716343447198,18.6805240933459,20.6065021157174));
#32538=CARTESIAN_POINT('Ctrl Pts',(6.55192346758059,18.8925325606821,20.6176808100472));
#32539=CARTESIAN_POINT('Ctrl Pts',(5.82802792947244,19.3533588159096,20.5417936269589));
#32540=CARTESIAN_POINT('Ctrl Pts',(5.46389362295823,19.5776706634904,20.431522865921));
#32541=CARTESIAN_POINT('Ctrl Pts',(5.00471097362036,19.8635098001506,20.1709617853684));
#32542=CARTESIAN_POINT('Ctrl Pts',(4.84708916414706,19.9622625901948,20.0510868608924));
#32543=CARTESIAN_POINT('Ctrl Pts',(4.63163511193388,20.1031710857547,19.798760634337));
#32544=CARTESIAN_POINT('Ctrl Pts',(4.55864104944201,20.1529191619863,19.6839455226377));
#32545=CARTESIAN_POINT('Ctrl Pts',(4.50580696382331,20.1925493450898,19.5550277686639));
#32546=CARTESIAN_POINT('',(18.4983482597372,19.9464420456703,9.15631398661356));
#32547=CARTESIAN_POINT('Ctrl Pts',(18.4983482597319,19.9464420456617,9.15631398658867));
#32548=CARTESIAN_POINT('Ctrl Pts',(18.6404422355597,19.872816673671,9.15203161624641));
#32549=CARTESIAN_POINT('Ctrl Pts',(18.7781534476127,19.791811258812,9.12772166732995));
#32550=CARTESIAN_POINT('Ctrl Pts',(19.0351386685812,19.625306229008,9.05215571502665));
#32551=CARTESIAN_POINT('Ctrl Pts',(19.1558466144338,19.5393897285476,9.00149281205167));
#32552=CARTESIAN_POINT('Ctrl Pts',(19.4948625508543,19.2783123963091,8.82266368252409));
#32553=CARTESIAN_POINT('Ctrl Pts',(19.6974081685334,19.0945659360765,8.66472676158745));
#32554=CARTESIAN_POINT('Ctrl Pts',(20.2020914679953,18.5673472018936,8.1562484341617));
#32555=CARTESIAN_POINT('Ctrl Pts',(20.4741688100664,18.1860724615003,7.7209118227428));
#32556=CARTESIAN_POINT('Ctrl Pts',(20.6511762848484,17.7903503023534,7.2142159717446));
#32557=CARTESIAN_POINT('',(18.0980606826517,20.1925493450899,8.66958605760119));
#32558=CARTESIAN_POINT('Ctrl Pts',(18.0980606826517,20.1925493450898,8.66958605760119));
#32559=CARTESIAN_POINT('Ctrl Pts',(18.1724796766112,20.1623540838435,8.75671278057142));
#32560=CARTESIAN_POINT('Ctrl Pts',(18.2448768581592,20.1252944701818,8.84318590991689));
#32561=CARTESIAN_POINT('Ctrl Pts',(18.3147595584651,20.0815864671188,8.92834702016679));
#32562=CARTESIAN_POINT('Ctrl Pts',(18.3781415805357,20.0419443009937,9.00558621306851));
#32563=CARTESIAN_POINT('Ctrl Pts',(18.4394559340548,19.9968331833493,9.0817458278276));
#32564=CARTESIAN_POINT('Ctrl Pts',(18.4983482597302,19.946442045657,9.15631398661009));
#32565=CARTESIAN_POINT('Ctrl Pts',(20.9558684429898,17.7903503023534,6.27435803496357));
#32566=CARTESIAN_POINT('Ctrl Pts',(20.8599066157679,18.0166341860667,6.59486317686292));
#32567=CARTESIAN_POINT('Ctrl Pts',(20.7268038872205,18.2443686579063,6.90554168138285));
#32568=CARTESIAN_POINT('Ctrl Pts',(20.3986530062068,18.6805240933459,7.47116844499778));
#32569=CARTESIAN_POINT('Ctrl Pts',(20.2046090588531,18.8925325606821,7.73242109238302));
#32570=CARTESIAN_POINT('Ctrl Pts',(19.6939365843773,19.3533588159097,8.25107052934689));
#32571=CARTESIAN_POINT('Ctrl Pts',(19.3806894051836,19.5776706634905,8.46700949907594));
#32572=CARTESIAN_POINT('Ctrl Pts',(18.8906788502492,19.8635098001506,8.66355577404548));
#32573=CARTESIAN_POINT('Ctrl Pts',(18.6986812695782,19.9622625901948,8.71204867410587));
#32574=CARTESIAN_POINT('Ctrl Pts',(18.3670712774808,20.1031710857547,8.72317460615268));
#32575=CARTESIAN_POINT('Ctrl Pts',(18.2317941549313,20.1529191619863,8.70865761099829));
#32576=CARTESIAN_POINT('Ctrl Pts',(18.0980606826517,20.1925493450899,8.6695860576012));
#32577=CARTESIAN_POINT('',(18.6922256707601,19.9464420456703,-8.75371524283479));
#32578=CARTESIAN_POINT('Ctrl Pts',(18.6922256707374,19.9464420456617,-8.75371524284621));
#32579=CARTESIAN_POINT('Ctrl Pts',(18.7774717236184,19.872816673671,-8.86747880085354));
#32580=CARTESIAN_POINT('Ctrl Pts',(18.844326976535,19.7918112588121,-8.99030276715853));
#32581=CARTESIAN_POINT('Ctrl Pts',(18.9454748005239,19.625306229008,-9.23833650406963));
#32582=CARTESIAN_POINT('Ctrl Pts',(18.9811251212272,19.5393897285476,-9.36429757965868));
#32583=CARTESIAN_POINT('Ctrl Pts',(19.0526838568059,19.2783123963091,-9.74084905034631));
#32584=CARTESIAN_POINT('Ctrl Pts',(19.0554889268077,19.0945659360765,-9.99767765042472));
#32585=CARTESIAN_POINT('Ctrl Pts',(18.9726094526565,18.5673472018935,-10.7092859942362));
#32586=CARTESIAN_POINT('Ctrl Pts',(18.8018870324763,18.1860724615002,-11.193432563529));
#32587=CARTESIAN_POINT('Ctrl Pts',(18.5160986195094,17.7903503023534,-11.6477422756871));
#32588=CARTESIAN_POINT('',(18.0621112303383,20.1925493450899,-8.74422771304759));
#32589=CARTESIAN_POINT('Ctrl Pts',(18.0621112303383,20.1925493450898,-8.74422771304759));
#32590=CARTESIAN_POINT('Ctrl Pts',(18.1766291291173,20.162354083844,-8.74808820217735));
#32591=CARTESIAN_POINT('Ctrl Pts',(18.2893754484039,20.1252944701829,-8.75077548367181));
#32592=CARTESIAN_POINT('Ctrl Pts',(18.3995282364447,20.0815864671208,-8.75231489509503));
#32593=CARTESIAN_POINT('Ctrl Pts',(18.4994343135196,20.0419443009952,-8.75371110629433));
#32594=CARTESIAN_POINT('Ctrl Pts',(18.5972071721593,19.9968331833502,-8.75416385508704));
#32595=CARTESIAN_POINT('Ctrl Pts',(18.692225670753,19.946442045657,-8.75371524283147));
#32596=CARTESIAN_POINT('Ctrl Pts',(17.9712605487941,17.7903503023534,-12.4719520361622));
#32597=CARTESIAN_POINT('Ctrl Pts',(18.1620087785714,18.0166323356831,-12.1970966186916));
#32598=CARTESIAN_POINT('Ctrl Pts',(18.3219213867259,18.244370505181,-11.8993230080315));
#32599=CARTESIAN_POINT('Ctrl Pts',(18.5595464636318,18.6805240933458,-11.2901043797534));
#32600=CARTESIAN_POINT('Ctrl Pts',(18.6428175859483,18.8925325606821,-10.9755063513766));
#32601=CARTESIAN_POINT('Ctrl Pts',(18.7299149642054,19.35335881591,-10.2528738989142));
#32602=CARTESIAN_POINT('Ctrl Pts',(18.7034364273428,19.5776706634907,-9.87333164697644));
#32603=CARTESIAN_POINT('Ctrl Pts',(18.5515859090712,19.8635098001506,-9.36768137035073));
#32604=CARTESIAN_POINT('Ctrl Pts',(18.4697906514847,19.9622625901948,-9.18733678857422));
#32605=CARTESIAN_POINT('Ctrl Pts',(18.2717338071635,20.1031710857547,-8.92113675168414));
#32606=CARTESIAN_POINT('Ctrl Pts',(18.1760400569865,20.1529191619863,-8.82442403684966));
#32607=CARTESIAN_POINT('Ctrl Pts',(18.0621112303383,20.1925493450898,-8.74422771304758));
#32608=CARTESIAN_POINT('',(4.81048155583834,19.9464420456703,-20.0720152820648));
#32609=CARTESIAN_POINT('Ctrl Pts',(4.81048155581525,19.9464420456617,-20.0720152820541));
#32610=CARTESIAN_POINT('Ctrl Pts',(4.77468841403889,19.8728182056928,-20.2095908854138));
#32611=CARTESIAN_POINT('Ctrl Pts',(4.72034220990053,19.7918094976896,-20.3384452522362));
#32612=CARTESIAN_POINT('Ctrl Pts',(4.58948764646888,19.625306229008,-20.5721698387655));
#32613=CARTESIAN_POINT('Ctrl Pts',(4.51323492339935,19.5393897285476,-20.6785778279124));
#32614=CARTESIAN_POINT('Ctrl Pts',(4.26345127071336,19.2783123963091,-20.9693007020821));
#32615=CARTESIAN_POINT('Ctrl Pts',(4.06440351811344,19.0945659360765,-21.1316238070946));
#32616=CARTESIAN_POINT('Ctrl Pts',(3.4563712048186,18.567347201894,-21.5105065702365));
#32617=CARTESIAN_POINT('Ctrl Pts',(2.97140648688581,18.1860724615007,-21.6788908559357));
#32618=CARTESIAN_POINT('Ctrl Pts',(2.4380266901546,17.7903503023534,-21.7387099497696));
#32619=CARTESIAN_POINT('',(4.42502927770989,20.1925493450898,-19.5734565969181));
#32620=CARTESIAN_POINT('Ctrl Pts',(4.42502927770989,20.1925493450898,-19.5734565969181));
#32621=CARTESIAN_POINT('Ctrl Pts',(4.49341176778961,20.162354083844,-19.6653972710923));
#32622=CARTESIAN_POINT('Ctrl Pts',(4.5616069467874,20.1252944701828,-19.7552213856496));
#32623=CARTESIAN_POINT('Ctrl Pts',(4.62908252646208,20.0815864671207,-19.8423021105449));
#32624=CARTESIAN_POINT('Ctrl Pts',(4.69028134479012,20.0419443009951,-19.9212823503358));
#32625=CARTESIAN_POINT('Ctrl Pts',(4.75088775179068,19.9968331833501,-19.9980065336062));
#32626=CARTESIAN_POINT('Ctrl Pts',(4.81048155583652,19.946442045657,-20.0720152820572));
#32627=CARTESIAN_POINT('Ctrl Pts',(1.45393257050235,17.7903503023534,-21.8266247734858));
#32628=CARTESIAN_POINT('Ctrl Pts',(1.78775549475546,18.0166341860667,-21.8043880131364));
#32629=CARTESIAN_POINT('Ctrl Pts',(2.1202627839953,18.2443686579063,-21.743754918874));
#32630=CARTESIAN_POINT('Ctrl Pts',(2.74472854424224,18.6805240933458,-21.549695261277));
#32631=CARTESIAN_POINT('Ctrl Pts',(3.04260988270327,18.8925325606821,-21.4186505839066));
#32632=CARTESIAN_POINT('Ctrl Pts',(3.66189101140341,19.3533588159101,-21.036192091666));
#32633=CARTESIAN_POINT('Ctrl Pts',(3.94211999519319,19.5776706634907,-20.7788496144794));
#32634=CARTESIAN_POINT('Ctrl Pts',(4.24277605102848,19.8635098001506,-20.3448603078825));
#32635=CARTESIAN_POINT('Ctrl Pts',(4.33277661380831,19.9622625901948,-20.1684671928266));
#32636=CARTESIAN_POINT('Ctrl Pts',(4.41741376066054,20.1031710857547,-19.8476471083627));
#32637=CARTESIAN_POINT('Ctrl Pts',(4.43336272853615,20.1529191619863,-19.7125313303895));
#32638=CARTESIAN_POINT('Ctrl Pts',(4.4250292777099,20.1925493450898,-19.5734565969181));
#32639=CARTESIAN_POINT('Origin',(7.5111559719605E-6,20.2903503023534,4.07573877568452E-6));
#32640=CARTESIAN_POINT('Ctrl Pts',(-10.7801530410109,17.7903503023534,19.0342827190051));
#32641=CARTESIAN_POINT('Ctrl Pts',(-9.25446266768857,16.6044337968475,19.8983652243397));
#32642=CARTESIAN_POINT('Ctrl Pts',(-7.73431157051831,15.2599230184859,20.514394463872));
#32643=CARTESIAN_POINT('Ctrl Pts',(-4.97570813316128,12.2573869722707,21.3487202901183));
#32644=CARTESIAN_POINT('Ctrl Pts',(-3.76084392376818,10.6406932625641,21.5730668416575));
#32645=CARTESIAN_POINT('Ctrl Pts',(-1.74098153262667,7.04601500804021,21.8296182862512));
#32646=CARTESIAN_POINT('Ctrl Pts',(-0.986571430673042,5.14830176393068,
21.8591019108078));
#32647=CARTESIAN_POINT('Ctrl Pts',(-0.278505434869228,2.43854448983318,
21.8739805820085));
#32648=CARTESIAN_POINT('Ctrl Pts',(-0.126302322075248,1.73945090916345,
21.8750040757347));
#32649=CARTESIAN_POINT('Ctrl Pts',(7.5104481972281E-6,1.03580637516255,
21.8750040757388));
#32650=CARTESIAN_POINT('Ctrl Pts',(-19.3643013307678,20.9435908393615,50.1865120070872));
#32651=CARTESIAN_POINT('Ctrl Pts',(-19.2220541116569,20.9358615047579,50.1240929228611));
#32652=CARTESIAN_POINT('Ctrl Pts',(-19.079806892546,20.9281321701544,50.061673838635));
#32653=CARTESIAN_POINT('Ctrl Pts',(-18.9375596734351,20.9204028355509,49.9992547544089));
#32654=CARTESIAN_POINT('Ctrl Pts',(-4.71283776234417,20.1474693751975,43.7573463318004));
#32655=CARTESIAN_POINT('Ctrl Pts',(4.99651958832846,20.0812550388979,28.7471447887935));
#32656=CARTESIAN_POINT('Ctrl Pts',(5.0291830418987,19.8399463130827,13.2252152613227));
#32657=CARTESIAN_POINT('Ctrl Pts',(-19.3642064856396,20.9469886892296,50.1865190303546));
#32658=CARTESIAN_POINT('Ctrl Pts',(-19.2219541714401,20.9392720585054,50.1241062032879));
#32659=CARTESIAN_POINT('Ctrl Pts',(-19.0797018572407,20.9315554277811,50.0616933762211));
#32660=CARTESIAN_POINT('Ctrl Pts',(-18.9374495430412,20.9238387970569,49.9992805491544));
#32661=CARTESIAN_POINT('Ctrl Pts',(-4.71221812309168,20.1521757246323,43.7579978424802));
#32662=CARTESIAN_POINT('Ctrl Pts',(4.99686729900256,20.0873688943554,28.7474275948137));
#32663=CARTESIAN_POINT('Ctrl Pts',(5.02977040929867,19.8474084919615,13.2255751562655));
#32664=CARTESIAN_POINT('Ctrl Pts',(-19.3641116405114,20.9503865390978,50.1865260536221));
#32665=CARTESIAN_POINT('Ctrl Pts',(-19.2218542312234,20.9426826122528,50.1241194837147));
#32666=CARTESIAN_POINT('Ctrl Pts',(-19.0795968219353,20.9349786854078,50.0617129138073));
#32667=CARTESIAN_POINT('Ctrl Pts',(-18.9373394126472,20.9272747585629,49.9993063438999));
#32668=CARTESIAN_POINT('Ctrl Pts',(-4.71159848383918,20.1568820740671,43.75864935316));
#32669=CARTESIAN_POINT('Ctrl Pts',(4.99721500967666,20.093482749813,28.747710400834));
#32670=CARTESIAN_POINT('Ctrl Pts',(5.03035777669865,19.8548706708402,13.2259350512082));
#32671=CARTESIAN_POINT('Ctrl Pts',(-19.3640167953833,20.9537843889659,50.1865330768895));
#32672=CARTESIAN_POINT('Ctrl Pts',(-19.2217542910066,20.9460931660003,50.1241327641415));
#32673=CARTESIAN_POINT('Ctrl Pts',(-19.0794917866299,20.9384019430346,50.0617324513934));
#32674=CARTESIAN_POINT('Ctrl Pts',(-18.9372292822533,20.9307107200689,49.9993321386454));
#32675=CARTESIAN_POINT('Ctrl Pts',(-4.71097884458669,20.1615884235019,43.7593008638397));
#32676=CARTESIAN_POINT('Ctrl Pts',(4.99756272035076,20.0995966052706,28.7479932068543));
#32677=CARTESIAN_POINT('Ctrl Pts',(5.03094514409862,19.862332849719,13.226294946151));
#32678=CARTESIAN_POINT('Ctrl Pts',(-19.363728775738,20.9641027630587,50.1865544047009));
#32679=CARTESIAN_POINT('Ctrl Pts',(-19.2214507989208,20.9564501184246,50.1241730932958));
#32680=CARTESIAN_POINT('Ctrl Pts',(-19.0791728221036,20.9487974737906,50.0617917818908));
#32681=CARTESIAN_POINT('Ctrl Pts',(-18.9368948452864,20.9411448291565,49.9994104704857));
#32682=CARTESIAN_POINT('Ctrl Pts',(-4.70909716356548,20.1758803657488,43.7612793299817));
#32683=CARTESIAN_POINT('Ctrl Pts',(4.99861862598245,20.1181627721728,28.7488520141665));
#32684=CARTESIAN_POINT('Ctrl Pts',(5.03272882401328,19.8849935193208,13.2273878521937));
#32685=CARTESIAN_POINT('Ctrl Pts',(-19.3631527362822,20.9847395112521,50.1865970600935));
#32686=CARTESIAN_POINT('Ctrl Pts',(-19.2208438146391,20.9771640232786,50.1242537514512));
#32687=CARTESIAN_POINT('Ctrl Pts',(-19.078534892996,20.9695885353052,50.061910442809));
#32688=CARTESIAN_POINT('Ctrl Pts',(-18.9362259713529,20.9620130473318,49.9995671341667));
#32689=CARTESIAN_POINT('Ctrl Pts',(-4.70533380704113,20.2044642499886,43.7652362699409));
#32690=CARTESIAN_POINT('Ctrl Pts',(5.00073044157035,20.1552951062578,28.7505696258898));
#32691=CARTESIAN_POINT('Ctrl Pts',(5.03629618384262,19.9303148585245,13.2295736642792));
#32692=CARTESIAN_POINT('Ctrl Pts',(-19.362288665564,21.0156946339229,50.1866610281067));
#32693=CARTESIAN_POINT('Ctrl Pts',(-19.2199333305268,21.0082348808134,50.1243747286337));
#32694=CARTESIAN_POINT('Ctrl Pts',(-19.0775779954895,21.000775127704,50.0620884291608));
#32695=CARTESIAN_POINT('Ctrl Pts',(-18.9352226604523,20.9933153745945,49.9998021296879));
#32696=CARTESIAN_POINT('Ctrl Pts',(-4.69968915672916,20.2473400636495,43.7711721823959));
#32697=CARTESIAN_POINT('Ctrl Pts',(5.00389843664987,20.2109936225946,28.7531458689445));
#32698=CARTESIAN_POINT('Ctrl Pts',(5.0416472235866,19.9982968673298,13.2328523824074));
#32699=CARTESIAN_POINT('Ctrl Pts',(-19.3614245796962,21.0466497571015,50.1867249762735));
#32700=CARTESIAN_POINT('Ctrl Pts',(-19.2190228363148,21.0393057386868,50.1244956925854));
#32701=CARTESIAN_POINT('Ctrl Pts',(-19.0766210929333,21.0319617202721,50.0622664088974));
#32702=CARTESIAN_POINT('Ctrl Pts',(-18.9342193495519,21.0246177018574,50.0000371252093));
#32703=CARTESIAN_POINT('Ctrl Pts',(-4.69404501140909,20.2902158603888,43.7771087564017));
#32704=CARTESIAN_POINT('Ctrl Pts',(5.00706678981436,20.2666921589687,28.7557218794068));
#32705=CARTESIAN_POINT('Ctrl Pts',(5.0469982633306,20.0662788761352,13.2361311005356));
#32706=CARTESIAN_POINT('Ctrl Pts',(-19.3608485148276,21.0672865061488,50.1867675983585));
#32707=CARTESIAN_POINT('Ctrl Pts',(-19.2184158350912,21.0600196441101,50.1245763285357));
#32708=CARTESIAN_POINT('Ctrl Pts',(-19.0759831553547,21.0527527820714,50.0623850587129));
#32709=CARTESIAN_POINT('Ctrl Pts',(-18.9335504756182,21.0454859200326,50.0001937888901));
#32710=CARTESIAN_POINT('Ctrl Pts',(-4.69028250197186,20.3187997161584,43.7810668066102));
#32711=CARTESIAN_POINT('Ctrl Pts',(5.00917920656114,20.3038245267329,28.7574391004138));
#32712=CARTESIAN_POINT('Ctrl Pts',(5.05056562315993,20.1116002153389,13.2383169126211));
#32713=CARTESIAN_POINT('Ctrl Pts',(-19.3605604823138,21.0776048806767,50.1867889092869));
#32714=CARTESIAN_POINT('Ctrl Pts',(-19.2181123344263,21.0703765968246,50.1246166464348));
#32715=CARTESIAN_POINT('Ctrl Pts',(-19.0756641865389,21.0631483129724,50.0624443835827));
#32716=CARTESIAN_POINT('Ctrl Pts',(-18.9332160386514,21.0559200291202,50.0002721207305));
#32717=CARTESIAN_POINT('Ctrl Pts',(-4.68840124990593,20.3330916439037,43.7830458355166));
#32718=CARTESIAN_POINT('Ctrl Pts',(5.01023541710294,20.3223907107576,28.7582977093251));
#32719=CARTESIAN_POINT('Ctrl Pts',(5.05234930307459,20.1342608849406,13.2394098186638));
#32720=CARTESIAN_POINT('Ctrl Pts',(-19.3605327274403,21.0785991614118,50.1867909628125));
#32721=CARTESIAN_POINT('Ctrl Pts',(-19.2180830890386,21.0713745949617,50.124620531476));
#32722=CARTESIAN_POINT('Ctrl Pts',(-19.0756334506368,21.0641500285117,50.0624501001396));
#32723=CARTESIAN_POINT('Ctrl Pts',(-18.9331838122351,21.0569254620617,50.0002796688031));
#32724=CARTESIAN_POINT('Ctrl Pts',(-4.68821997206204,20.3344688170607,43.7832365351574));
#32725=CARTESIAN_POINT('Ctrl Pts',(5.01033719377241,20.3241797521467,28.75838044506));
#32726=CARTESIAN_POINT('Ctrl Pts',(5.05252117884551,20.1364444718193,13.2395151313195));
#32727=CARTESIAN_POINT('Ctrl Pts',(-19.3605049725668,21.0795934421468,50.186793016338));
#32728=CARTESIAN_POINT('Ctrl Pts',(-19.2180538436508,21.0723725930989,50.1246244165172));
#32729=CARTESIAN_POINT('Ctrl Pts',(-19.0756027147348,21.0651517440511,50.0624558166965));
#32730=CARTESIAN_POINT('Ctrl Pts',(-18.9331515858188,21.0579308950032,50.0002872168757));
#32731=CARTESIAN_POINT('Ctrl Pts',(-4.68803869421815,20.3358459902176,43.7834272347982));
#32732=CARTESIAN_POINT('Ctrl Pts',(5.01043897044188,20.3259687935359,28.7584631807949));
#32733=CARTESIAN_POINT('Ctrl Pts',(5.05269305461643,20.1386280586979,13.2396204439751));
#32734=CARTESIAN_POINT('Ctrl Pts',(-19.3604772176933,21.0805877228818,50.1867950698636));
#32735=CARTESIAN_POINT('Ctrl Pts',(-19.218024598263,21.0733705912361,50.1246283015585));
#32736=CARTESIAN_POINT('Ctrl Pts',(-19.0755719788328,21.0661534595904,50.0624615332534));
#32737=CARTESIAN_POINT('Ctrl Pts',(-18.9331193594025,21.0589363279447,50.0002947649483));
#32738=CARTESIAN_POINT('Ctrl Pts',(-4.68785741637426,20.3372231633746,43.7836179344389));
#32739=CARTESIAN_POINT('Ctrl Pts',(5.01054074711136,20.327757834925,28.7585459165298));
#32740=CARTESIAN_POINT('Ctrl Pts',(5.05286493038735,20.1408116455766,13.2397257566308));
#32741=CARTESIAN_POINT('',(-11.284173078362,20.5529756002005,45.4965192546307));
#32742=CARTESIAN_POINT('Ctrl Pts',(4.37484296764849,19.9464420456703,20.1714550984892));
#32743=CARTESIAN_POINT('Ctrl Pts',(3.44448305305149,20.0189549105364,25.1661789821446));
#32744=CARTESIAN_POINT('Ctrl Pts',(1.55215272586899,20.0954766247834,29.9700084636964));
#32745=CARTESIAN_POINT('Ctrl Pts',(-3.79011625520565,20.2752040736288,38.6053112430901));
#32746=CARTESIAN_POINT('Ctrl Pts',(-7.23855178728743,20.3824974081048,42.4380069630988));
#32747=CARTESIAN_POINT('Ctrl Pts',(-11.284173078368,20.5529756002053,45.4965192546226));
#32748=CARTESIAN_POINT('',(-11.2641171037461,20.7105311502992,45.5014889049172));
#32749=CARTESIAN_POINT('',(-11.2841730783683,20.5529756002016,45.4965192546224));
#32750=CARTESIAN_POINT('Ctrl Pts',(-11.264117103744,20.7105311502982,45.50148890492));
#32751=CARTESIAN_POINT('Ctrl Pts',(-7.12723823252845,20.5483438544847,42.3780169116778));
#32752=CARTESIAN_POINT('Ctrl Pts',(-3.61607404464229,20.4520245495079,38.4420106405091));
#32753=CARTESIAN_POINT('Ctrl Pts',(1.76528630148522,20.3052748660675,29.5836747606129));
#32754=CARTESIAN_POINT('Ctrl Pts',(3.63859976812651,20.248474007324,24.6615284366429));
#32755=CARTESIAN_POINT('Ctrl Pts',(4.50580696382332,20.1925493450898,19.5550277686639));
#32756=CARTESIAN_POINT('Ctrl Pts',(16.3617859818256,-4.68328060676847,50.8901188958912));
#32757=CARTESIAN_POINT('Ctrl Pts',(16.622166238714,-4.67927906663786,50.5796103403414));
#32758=CARTESIAN_POINT('Ctrl Pts',(16.8774519664815,-4.67486342687383,50.2628798120286));
#32759=CARTESIAN_POINT('Ctrl Pts',(17.9410437802702,-4.65418501649615,48.8890505498656));
#32760=CARTESIAN_POINT('Ctrl Pts',(19.4134795663389,-4.61395560865182,46.711300994988));
#32761=CARTESIAN_POINT('Ctrl Pts',(21.157886103088,-4.53496565777432,43.2616774490902));
#32762=CARTESIAN_POINT('Ctrl Pts',(22.6517756066693,-4.42959393838223,39.075796489912));
#32763=CARTESIAN_POINT('Ctrl Pts',(23.4697878015651,-4.31850354734918,34.7535560407194));
#32764=CARTESIAN_POINT('Ctrl Pts',(23.6135578037238,-4.2170896233612,30.3929554510995));
#32765=CARTESIAN_POINT('Ctrl Pts',(23.2191400843552,-4.13063759391767,26.0539326403806));
#32766=CARTESIAN_POINT('Ctrl Pts',(22.1536599527665,-4.07121155600733,21.8071760633296));
#32767=CARTESIAN_POINT('Ctrl Pts',(20.4200758048662,-4.04803120464602,17.7504657469389));
#32768=CARTESIAN_POINT('Ctrl Pts',(18.4775377675087,-4.055480889925,14.4481772758194));
#32769=CARTESIAN_POINT('Ctrl Pts',(16.8791012600192,-4.07952578289679,12.3929056948357));
#32770=CARTESIAN_POINT('Ctrl Pts',(15.7266400983712,-4.10152925776619,11.0970184802139));
#32771=CARTESIAN_POINT('Ctrl Pts',(15.4437103800753,-4.1072571624472,10.7918674138708));
#32772=CARTESIAN_POINT('Ctrl Pts',(15.155735551125,-4.11341014061892,10.4938062779888));
#32773=CARTESIAN_POINT('Ctrl Pts',(16.0716182464065,-4.24009445412503,50.8866381127899));
#32774=CARTESIAN_POINT('Ctrl Pts',(16.3335846412505,-4.23725223817857,50.5777035993082));
#32775=CARTESIAN_POINT('Ctrl Pts',(16.5905075369587,-4.23400446880359,50.2625298947483));
#32776=CARTESIAN_POINT('Ctrl Pts',(17.6612842305945,-4.21832863439708,48.8952428878293));
#32777=CARTESIAN_POINT('Ctrl Pts',(19.1454696712926,-4.18572164472913,46.7268968947991));
#32778=CARTESIAN_POINT('Ctrl Pts',(20.9096158518361,-4.11799618192084,43.2893924007819));
#32779=CARTESIAN_POINT('Ctrl Pts',(22.4288153906464,-4.02550335874969,39.115138864075));
#32780=CARTESIAN_POINT('Ctrl Pts',(23.2747425690519,-3.92690475481451,34.801140787119));
#32781=CARTESIAN_POINT('Ctrl Pts',(23.448651990639,-3.83755718932749,30.4450413824504));
#32782=CARTESIAN_POINT('Ctrl Pts',(23.0859365661942,-3.76285616468038,26.1073385430749));
#32783=CARTESIAN_POINT('Ctrl Pts',(22.0538376043168,-3.71481495977278,21.8577037769588));
#32784=CARTESIAN_POINT('Ctrl Pts',(20.3548967622918,-3.70275434803773,17.7935954675031));
#32785=CARTESIAN_POINT('Ctrl Pts',(18.4427064539546,-3.71962751323487,14.4817346886381));
#32786=CARTESIAN_POINT('Ctrl Pts',(16.8648199692177,-3.74992063397164,12.4178382951194));
#32787=CARTESIAN_POINT('Ctrl Pts',(15.7259553229615,-3.77604797989279,11.1155040507245));
#32788=CARTESIAN_POINT('Ctrl Pts',(15.4462443232874,-3.78276245762616,10.8087153709496));
#32789=CARTESIAN_POINT('Ctrl Pts',(15.1614301028927,-3.78989370687861,10.5089349485779));
#32790=CARTESIAN_POINT('Ctrl Pts',(15.775594122299,-3.80075287541765,50.8831473876396));
#32791=CARTESIAN_POINT('Ctrl Pts',(16.0391680422694,-3.79905339336963,50.5757898857823));
#32792=CARTESIAN_POINT('Ctrl Pts',(16.2977495463562,-3.79695621683146,50.262175383072));
#32793=CARTESIAN_POINT('Ctrl Pts',(17.3758025240791,-3.78620663871065,48.9014382062803));
#32794=CARTESIAN_POINT('Ctrl Pts',(18.8718656085796,-3.76109400159902,46.7425044935959));
#32795=CARTESIAN_POINT('Ctrl Pts',(20.6559095081701,-3.70440674399875,43.3171275041978));
#32796=CARTESIAN_POINT('Ctrl Pts',(22.2005654978869,-3.62448835210827,39.1545089959556));
#32797=CARTESIAN_POINT('Ctrl Pts',(23.0745120366084,-3.53802316526296,34.8487637167761));
#32798=CARTESIAN_POINT('Ctrl Pts',(23.2786330544031,-3.46032715355504,30.4971820176086));
#32799=CARTESIAN_POINT('Ctrl Pts',(22.9476767342877,-3.39690914788247,26.1608222559414));
#32800=CARTESIAN_POINT('Ctrl Pts',(21.9490106855406,-3.35971861494906,21.9083363993147));
#32801=CARTESIAN_POINT('Ctrl Pts',(20.2847821490872,-3.35817927654809,17.8368515221065));
#32802=CARTESIAN_POINT('Ctrl Pts',(18.4030315624581,-3.38391914529348,14.515421853483));
#32803=CARTESIAN_POINT('Ctrl Pts',(16.8457803567792,-3.42007079724739,12.4428866920255));
#32804=CARTESIAN_POINT('Ctrl Pts',(15.7205799195479,-3.45006162272336,11.1340878840826));
#32805=CARTESIAN_POINT('Ctrl Pts',(15.4441049216842,-3.45770043113048,10.8256556958562));
#32806=CARTESIAN_POINT('Ctrl Pts',(15.1624694438579,-3.46574819271174,10.5241484978699));
#32807=CARTESIAN_POINT('Ctrl Pts',(14.711130350501,-2.2653457359543,50.8708167537008));
#32808=CARTESIAN_POINT('Ctrl Pts',(14.9804500746946,-2.26761569662348,50.5690252215433));
#32809=CARTESIAN_POINT('Ctrl Pts',(15.2449567812268,-2.26951335386862,50.2609131963582));
#32810=CARTESIAN_POINT('Ctrl Pts',(16.3489904126773,-2.27586002752392,48.9232880647604));
#32811=CARTESIAN_POINT('Ctrl Pts',(17.8873879492628,-2.27671432942662,46.7975592517765));
#32812=CARTESIAN_POINT('Ctrl Pts',(19.7421505042058,-2.25814179129592,43.4149557959663));
#32813=CARTESIAN_POINT('Ctrl Pts',(21.3770820388576,-2.2214798205824,39.2933713189624));
#32814=CARTESIAN_POINT('Ctrl Pts',(22.3501898623555,-2.17652897108851,35.016748143073));
#32815=CARTESIAN_POINT('Ctrl Pts',(22.6610854561747,-2.13845241575724,30.6811445102227));
#32816=CARTESIAN_POINT('Ctrl Pts',(22.442302689862,-2.11316923258448,26.3495962450917));
#32817=CARTESIAN_POINT('Ctrl Pts',(21.5616897778755,-2.11235831802136,22.0871532550128));
#32818=CARTESIAN_POINT('Ctrl Pts',(20.0200811689669,-2.14581153060268,17.9897419444869));
#32819=CARTESIAN_POINT('Ctrl Pts',(18.2459645155416,-2.20085463389179,14.6345975930576));
#32820=CARTESIAN_POINT('Ctrl Pts',(16.7617576425575,-2.25628908058851,12.5315664711582));
#32821=CARTESIAN_POINT('Ctrl Pts',(15.684964406382,-2.29898278275007,11.1999224907658));
#32822=CARTESIAN_POINT('Ctrl Pts',(15.4199619835964,-2.30966173471912,10.8856758941311));
#32823=CARTESIAN_POINT('Ctrl Pts',(15.1496042586498,-2.32072459453129,10.5780537474731));
#32824=CARTESIAN_POINT('Ctrl Pts',(12.7120990401115,0.42091842584111,50.8486555071386));
#32825=CARTESIAN_POINT('Ctrl Pts',(12.9919285081875,0.412015546281074,50.5568402051828));
#32826=CARTESIAN_POINT('Ctrl Pts',(13.2672633776138,0.403442573942463,50.2585955704578));
#32827=CARTESIAN_POINT('Ctrl Pts',(14.4187373325809,0.368526239150617,48.962439393581));
#32828=CARTESIAN_POINT('Ctrl Pts',(16.0343139487426,0.324281374370589,46.8962890085149));
#32829=CARTESIAN_POINT('Ctrl Pts',(18.0176707105305,0.279215865745994,43.5904340408452));
#32830=CARTESIAN_POINT('Ctrl Pts',(19.8164276316666,0.243759038204317,39.5424793938405));
#32831=CARTESIAN_POINT('Ctrl Pts',(20.9691269648152,0.21967725703067,35.3181165575201));
#32832=CARTESIAN_POINT('Ctrl Pts',(21.4731024416312,0.192114722189047,31.0111945273764));
#32833=CARTESIAN_POINT('Ctrl Pts',(21.4569532754525,0.154437491851918,26.6882970928525));
#32834=CARTESIAN_POINT('Ctrl Pts',(20.7893622142715,0.0954817696064694,
22.4080135319735));
#32835=CARTESIAN_POINT('Ctrl Pts',(19.4688186408849,0.0048363712043943,
18.2641179914593));
#32836=CARTESIAN_POINT('Ctrl Pts',(17.8886301147695,-0.0979118428630517,
14.8485179207147));
#32837=CARTESIAN_POINT('Ctrl Pts',(16.5359594711211,-0.184631554593919,
12.6907998414015));
#32838=CARTESIAN_POINT('Ctrl Pts',(15.546316269121,-0.247909792323189,11.3181882229936));
#32839=CARTESIAN_POINT('Ctrl Pts',(15.3019963909978,-0.263520166061751,
10.9935053189798));
#32840=CARTESIAN_POINT('Ctrl Pts',(15.0519971607038,-0.279478515480188,
10.6748977105072));
#32841=CARTESIAN_POINT('Ctrl Pts',(9.60863066089747,3.93922736422659,50.8171955610112));
#32842=CARTESIAN_POINT('Ctrl Pts',(9.90380565178832,3.92273017306588,50.5393909649465));
#32843=CARTESIAN_POINT('Ctrl Pts',(10.1949269853701,3.90651491483579,50.2550114362429));
#32844=CARTESIAN_POINT('Ctrl Pts',(11.415467332142,3.83888692720806,49.0171607997061));
#32845=CARTESIAN_POINT('Ctrl Pts',(13.1430409691099,3.74496038387833,47.0347818971594));
#32846=CARTESIAN_POINT('Ctrl Pts',(15.312014670943,3.6271896762232,43.8368541553498));
#32847=CARTESIAN_POINT('Ctrl Pts',(17.3462446376419,3.50969140214063,39.8924608868101));
#32848=CARTESIAN_POINT('Ctrl Pts',(18.7559848214645,3.40771510315772,35.7416355306005));
#32849=CARTESIAN_POINT('Ctrl Pts',(19.5353770821765,3.30695483103527,31.4751239969068));
#32850=CARTESIAN_POINT('Ctrl Pts',(19.8076156218556,3.1998573133211,27.1644954735594));
#32851=CARTESIAN_POINT('Ctrl Pts',(19.4424544689053,3.07607789704229,22.8592635001078));
#32852=CARTESIAN_POINT('Ctrl Pts',(18.4351120717144,2.92448144596071,18.6501806821044));
#32853=CARTESIAN_POINT('Ctrl Pts',(17.1292759578971,2.77158317941627,15.1497511982359));
#32854=CARTESIAN_POINT('Ctrl Pts',(15.9624469754747,2.65236568914073,12.9152769022098));
#32855=CARTESIAN_POINT('Ctrl Pts',(15.0958611037723,2.56779645721963,11.4851600873672));
#32856=CARTESIAN_POINT('Ctrl Pts',(14.8808083544882,2.54707902977605,11.1458176192315));
#32857=CARTESIAN_POINT('Ctrl Pts',(14.6596795118079,2.52604544176493,10.81176741508));
#32858=CARTESIAN_POINT('Ctrl Pts',(5.74244455804017,7.64857049485316,50.7803662328039));
#32859=CARTESIAN_POINT('Ctrl Pts',(6.05569741160819,7.62538079009264,50.5186066375066));
#32860=CARTESIAN_POINT('Ctrl Pts',(6.36538250903781,7.6024320797305,50.2501220962308));
#32861=CARTESIAN_POINT('Ctrl Pts',(7.66700342527438,7.50598047950645,49.0791935344687));
#32862=CARTESIAN_POINT('Ctrl Pts',(9.52575081707664,7.36825978906471,47.1929758832822));
#32863=CARTESIAN_POINT('Ctrl Pts',(11.9112808060609,7.18657585481396,44.1189689523312));
#32864=CARTESIAN_POINT('Ctrl Pts',(14.2193661405577,6.99739878870591,40.2935266180449));
#32865=CARTESIAN_POINT('Ctrl Pts',(15.9270736912541,6.82819742189185,36.2272337144719));
#32866=CARTESIAN_POINT('Ctrl Pts',(17.024880309348,6.66543158101024,32.0072748538597));
#32867=CARTESIAN_POINT('Ctrl Pts',(17.6299082160355,6.50060855796851,27.7109331227746));
#32868=CARTESIAN_POINT('Ctrl Pts',(17.6130179265134,6.32441606849526,23.3773141230994));
#32869=CARTESIAN_POINT('Ctrl Pts',(16.9656867939234,6.12505774886043,19.093703489216));
#32870=CARTESIAN_POINT('Ctrl Pts',(15.9747785941321,5.93384517916791,15.496190967554));
#32871=CARTESIAN_POINT('Ctrl Pts',(15.0210039512143,5.79035915091665,13.1738276179752));
#32872=CARTESIAN_POINT('Ctrl Pts',(14.295408729852,5.69001969995687,11.6778536150283));
#32873=CARTESIAN_POINT('Ctrl Pts',(14.1139837591531,5.66551509710643,11.3217339373774));
#32874=CARTESIAN_POINT('Ctrl Pts',(13.9261211880402,5.64071489355821,10.9700178599298));
#32875=CARTESIAN_POINT('Ctrl Pts',(2.10026812882245,10.6050661536892,50.7471135490468));
#32876=CARTESIAN_POINT('Ctrl Pts',(2.42970188215053,10.5777689837161,50.4994231232871));
#32877=CARTESIAN_POINT('Ctrl Pts',(2.75597229567527,10.5506896266998,50.2448900518966));
#32878=CARTESIAN_POINT('Ctrl Pts',(4.12990684291117,10.4365567481294,49.1327687224161));
#32879=CARTESIAN_POINT('Ctrl Pts',(6.10543909625537,10.2719415070743,47.3310635731816));
#32880=CARTESIAN_POINT('Ctrl Pts',(8.68319308440481,10.0511774947007,44.3660022123056));
#32881=CARTESIAN_POINT('Ctrl Pts',(11.2337573042792,9.81863871620139,40.6451852338454));
#32882=CARTESIAN_POINT('Ctrl Pts',(13.2046001804074,9.60967367489776,36.6533198393472));
#32883=CARTESIAN_POINT('Ctrl Pts',(14.5829691071597,9.41153176383594,32.4744597064717));
#32884=CARTESIAN_POINT('Ctrl Pts',(15.4807568161021,9.21500541081661,28.1908990385021));
#32885=CARTESIAN_POINT('Ctrl Pts',(15.769686211672,9.01175979868378,23.8326054364364));
#32886=CARTESIAN_POINT('Ctrl Pts',(15.4379491375815,8.78956564702969,19.4838165836314));
#32887=CARTESIAN_POINT('Ctrl Pts',(14.722757944353,8.58124477590158,15.8012895296554));
#32888=CARTESIAN_POINT('Ctrl Pts',(13.9552770836213,8.42762540105217,13.4019109616667));
#32889=CARTESIAN_POINT('Ctrl Pts',(13.3528872797445,8.32086564673385,11.8482144895222));
#32890=CARTESIAN_POINT('Ctrl Pts',(13.2009274270766,8.29482075310626,11.4774240473852));
#32891=CARTESIAN_POINT('Ctrl Pts',(13.0422921111672,8.26849188852043,11.1102890366025));
#32892=CARTESIAN_POINT('Ctrl Pts',(-2.32344597549834,13.6252616883324,50.7074105587169));
#32893=CARTESIAN_POINT('Ctrl Pts',(-1.9752998919414,13.5952855444977,50.4758359591679));
#32894=CARTESIAN_POINT('Ctrl Pts',(-1.62988469132187,13.5655149131873,50.2372979642494));
#32895=CARTESIAN_POINT('Ctrl Pts',(-0.172623734997204,13.4398628522405,
49.1926684568959));
#32896=CARTESIAN_POINT('Ctrl Pts',(1.93734073331834,13.2576618204372,47.4879749039095));
#32897=CARTESIAN_POINT('Ctrl Pts',(4.73595880494755,13.0115743729063,44.6480286235722));
#32898=CARTESIAN_POINT('Ctrl Pts',(7.56468089622281,12.751644575675,41.0474413376908));
#32899=CARTESIAN_POINT('Ctrl Pts',(9.83683823314094,12.5189796899122,37.1412195468378));
#32900=CARTESIAN_POINT('Ctrl Pts',(11.535949107776,12.301865256328,33.0098190474629));
#32901=CARTESIAN_POINT('Ctrl Pts',(12.7680096168006,12.0904144587841,28.7412692264177));
#32902=CARTESIAN_POINT('Ctrl Pts',(13.4056044510136,11.8774764455751,24.3550594803262));
#32903=CARTESIAN_POINT('Ctrl Pts',(13.4331412637371,11.6504923923572,19.9319241108741));
#32904=CARTESIAN_POINT('Ctrl Pts',(13.0314530758916,11.4410171343385,16.1522546984861));
#32905=CARTESIAN_POINT('Ctrl Pts',(12.4755385167765,11.2882220371981,13.6647941021625));
#32906=CARTESIAN_POINT('Ctrl Pts',(12.0129796713749,11.1823584691134,12.0450596698024));
#32907=CARTESIAN_POINT('Ctrl Pts',(11.8945374044748,11.1565388193505,11.657551735864));
#32908=CARTESIAN_POINT('Ctrl Pts',(11.7692258288562,11.1304479812224,11.2729059637599));
#32909=CARTESIAN_POINT('Ctrl Pts',(-6.40110428036058,15.9398275064074,50.6708432675152));
#32910=CARTESIAN_POINT('Ctrl Pts',(-6.03650538939953,15.9092719019138,50.4534079698693));
#32911=CARTESIAN_POINT('Ctrl Pts',(-5.67428759415347,15.8789225535602,50.2289124185247));
#32912=CARTESIAN_POINT('Ctrl Pts',(-4.14402253391207,15.7507918597713,49.2435830363373));
#32913=CARTESIAN_POINT('Ctrl Pts',(-1.91634595810908,15.5646999212503,47.6241454237767));
#32914=CARTESIAN_POINT('Ctrl Pts',(1.07545108130911,15.3133344724918,44.8942114163047));
#32915=CARTESIAN_POINT('Ctrl Pts',(4.14720811862536,15.0487502016962,41.3994183816965));
#32916=CARTESIAN_POINT('Ctrl Pts',(6.68230321143587,14.8142492774957,37.5686748221223));
#32917=CARTESIAN_POINT('Ctrl Pts',(8.66095132605825,14.5991383033468,33.4792697502678));
#32918=CARTESIAN_POINT('Ctrl Pts',(10.1840492935139,14.3930646018661,29.2242550823646));
#32919=CARTESIAN_POINT('Ctrl Pts',(11.1248270635106,14.1899609567462,24.8139220984123));
#32920=CARTESIAN_POINT('Ctrl Pts',(11.46434688115,13.977122935371,20.3259202309031));
#32921=CARTESIAN_POINT('Ctrl Pts',(11.3345865749015,13.7824369346935,16.4613224208427));
#32922=CARTESIAN_POINT('Ctrl Pts',(10.9619607427361,13.6409944051188,13.8967724687642));
#32923=CARTESIAN_POINT('Ctrl Pts',(10.6204652415869,13.5429643472183,12.2192199886043));
#32924=CARTESIAN_POINT('Ctrl Pts',(10.5310903287026,13.5190447294408,11.8171499065311));
#32925=CARTESIAN_POINT('Ctrl Pts',(10.4347273407624,13.4948677704672,11.4173185836932));
#32926=CARTESIAN_POINT('Ctrl Pts',(-11.2581355126793,18.188947172369,50.6263769819591));
#32927=CARTESIAN_POINT('Ctrl Pts',(-10.874837896557,18.1597316481657,50.4251496671371));
#32928=CARTESIAN_POINT('Ctrl Pts',(-10.4935569470502,18.1307342364494,50.2167577112658));
#32929=CARTESIAN_POINT('Ctrl Pts',(-8.88060641151116,18.0083786966032,49.2994700730556));
#32930=CARTESIAN_POINT('Ctrl Pts',(-6.51959375012864,17.830846834045,47.7778825471059));
#32931=CARTESIAN_POINT('Ctrl Pts',(-3.30898627378599,17.5925027676131,45.1742926484351));
#32932=CARTESIAN_POINT('Ctrl Pts',(0.0379893981926304,17.3443426911773,
41.801106220426));
#32933=CARTESIAN_POINT('Ctrl Pts',(2.87070487089537,17.1289494695207,38.0572826893845));
#32934=CARTESIAN_POINT('Ctrl Pts',(5.16554290078262,16.9369213116231,34.0164684807631));
#32935=CARTESIAN_POINT('Ctrl Pts',(7.01762411454711,16.7575317657622,29.7774553228848));
#32936=CARTESIAN_POINT('Ctrl Pts',(8.30079284685546,16.5859876106103,25.3399902329922));
#32937=CARTESIAN_POINT('Ctrl Pts',(8.99223520193867,16.4095763329362,20.7781720131405));
#32938=CARTESIAN_POINT('Ctrl Pts',(9.16889682817149,16.2491906636996,16.8166904505901));
#32939=CARTESIAN_POINT('Ctrl Pts',(9.00256941244382,16.1323920433636,14.1640860328959));
#32940=CARTESIAN_POINT('Ctrl Pts',(8.7972460292566,16.0510402241362,12.4204614509089));
#32941=CARTESIAN_POINT('Ctrl Pts',(8.74059622159544,16.0311583490605,12.0018473869615));
#32942=CARTESIAN_POINT('Ctrl Pts',(8.67685658165753,16.01103806515,11.5848534084937));
#32943=CARTESIAN_POINT('Ctrl Pts',(-15.657276494051,19.7983627848149,50.5847597853741));
#32944=CARTESIAN_POINT('Ctrl Pts',(-15.2578253879166,19.7720645135703,50.3977633519486));
#32945=CARTESIAN_POINT('Ctrl Pts',(-14.860102865805,19.7460021313493,50.2035126492778));
#32946=CARTESIAN_POINT('Ctrl Pts',(-13.175951969311,19.6361820466171,49.3459910091793));
#32947=CARTESIAN_POINT('Ctrl Pts',(-10.7000587998586,19.4774394485581,47.9103778968689));
#32948=CARTESIAN_POINT('Ctrl Pts',(-7.30079683975733,19.2670183310104,45.4178765118453));
#32949=CARTESIAN_POINT('Ctrl Pts',(-3.71645296456281,19.0520629838802,42.1517164114004));
#32950=CARTESIAN_POINT('Ctrl Pts',(-0.627027603513927,18.8717166252608,
38.4845463961827));
#32951=CARTESIAN_POINT('Ctrl Pts',(1.94045298184077,18.7178122962125,34.4868040712865));
#32952=CARTESIAN_POINT('Ctrl Pts',(4.07608978829918,18.5794411422907,30.2623003349598));
#32953=CARTESIAN_POINT('Ctrl Pts',(5.65415883179733,18.4529446490623,25.8015291609108));
#32954=CARTESIAN_POINT('Ctrl Pts',(6.64840096894227,18.3257380682571,21.1754591429953));
#32955=CARTESIAN_POINT('Ctrl Pts',(7.08845542629894,18.2102139945187,17.1294161466707));
#32956=CARTESIAN_POINT('Ctrl Pts',(7.09925335497196,18.1249152482566,14.3998463939675));
#32957=CARTESIAN_POINT('Ctrl Pts',(7.0107674651366,18.064727637235,12.5984411589748));
#32958=CARTESIAN_POINT('Ctrl Pts',(6.982201638659,18.0499634327475,12.1654452776201));
#32959=CARTESIAN_POINT('Ctrl Pts',(6.94646609919288,18.0349776243875,11.7336121997143));
#32960=CARTESIAN_POINT('Ctrl Pts',(-18.8793254736515,20.6836496418694,50.5527496580464));
#32961=CARTESIAN_POINT('Ctrl Pts',(-18.468609657083,20.6606519170286,50.3759538221809));
#32962=CARTESIAN_POINT('Ctrl Pts',(-18.0594351009059,20.6379063239872,50.1918393727547));
#32963=CARTESIAN_POINT('Ctrl Pts',(-16.3257493528884,20.5422448076096,49.3771603969211));
#32964=CARTESIAN_POINT('Ctrl Pts',(-13.7698304039347,20.4047755971079,48.0031978573159));
#32965=CARTESIAN_POINT('Ctrl Pts',(-10.2389125796356,20.225761668211,45.5904189129039));
#32966=CARTESIAN_POINT('Ctrl Pts',(-6.4887184482965,20.0475517349526,42.4011488849344));
#32967=CARTESIAN_POINT('Ctrl Pts',(-3.21976533941777,19.9048724048602,38.7891722537331));
#32968=CARTESIAN_POINT('Ctrl Pts',(-0.461559957111977,19.790507905872,34.8226183318397));
#32969=CARTESIAN_POINT('Ctrl Pts',(1.87242626469179,19.6935273080542,30.6088777136648));
#32970=CARTESIAN_POINT('Ctrl Pts',(3.65670540538569,19.6110850660289,26.1318176353169));
#32971=CARTESIAN_POINT('Ctrl Pts',(4.86251201139915,19.530779076001,21.4601528010746));
#32972=CARTESIAN_POINT('Ctrl Pts',(5.48643851700597,19.4573327991495,17.3539164024331));
#32973=CARTESIAN_POINT('Ctrl Pts',(5.6207501220497,19.4012238336331,14.5694714880378));
#32974=CARTESIAN_POINT('Ctrl Pts',(5.61368274593469,19.3605693891818,12.7268457580551));
#32975=CARTESIAN_POINT('Ctrl Pts',(5.60468015267822,19.3505226070412,12.2836407679017));
#32976=CARTESIAN_POINT('Ctrl Pts',(5.58844640000097,19.3402634731691,11.8413221987243));
#32977=CARTESIAN_POINT('Ctrl Pts',(-20.6920217811532,21.117312799858,50.5343146756899));
#32978=CARTESIAN_POINT('Ctrl Pts',(-20.2750932994788,21.0964267127388,50.3632222074524));
#32979=CARTESIAN_POINT('Ctrl Pts',(-19.8596072866037,21.0758020890032,50.1847744350595));
#32980=CARTESIAN_POINT('Ctrl Pts',(-18.098641284761,20.9891913310095,49.3940446371234));
#32981=CARTESIAN_POINT('Ctrl Pts',(-15.4986177759893,20.8653273744228,48.0545498997513));
#32982=CARTESIAN_POINT('Ctrl Pts',(-11.8950631088073,20.7063681300896,45.6863574981545));
#32983=CARTESIAN_POINT('Ctrl Pts',(-8.05329901501471,20.5515335415639,42.540109695465));
#32984=CARTESIAN_POINT('Ctrl Pts',(-4.68516379227482,20.4326519806542,38.9590447934805));
#32985=CARTESIAN_POINT('Ctrl Pts',(-1.8215597727922,20.3430531321453,35.0099997569466));
#32986=CARTESIAN_POINT('Ctrl Pts',(0.62204841812851,20.2718184169426,30.8023618711775));
#32987=CARTESIAN_POINT('Ctrl Pts',(2.52028916562565,20.2165549432469,26.3162953955452));
#32988=CARTESIAN_POINT('Ctrl Pts',(3.84298678509366,20.164982094833,21.6192526187751));
#32989=CARTESIAN_POINT('Ctrl Pts',(4.56847237094525,20.117197691553,17.4794679698934));
#32990=CARTESIAN_POINT('Ctrl Pts',(4.77097609751765,20.0788282397779,14.6644175519522));
#32991=CARTESIAN_POINT('Ctrl Pts',(4.8088478494176,20.0500302875854,12.7987962353339));
#32992=CARTESIAN_POINT('Ctrl Pts',(4.81063894211702,20.0428451797642,12.3499110360814));
#32993=CARTESIAN_POINT('Ctrl Pts',(4.80516116754767,20.0354515632684,11.9017729301386));
#32994=CARTESIAN_POINT('Ctrl Pts',(-21.2075547412075,21.2334813897109,50.5290240335005));
#32995=CARTESIAN_POINT('Ctrl Pts',(-20.7888675617946,21.2132228077857,50.3595499677703));
#32996=CARTESIAN_POINT('Ctrl Pts',(-20.371595394195,21.1932283095702,50.1827099013443));
#32997=CARTESIAN_POINT('Ctrl Pts',(-18.6029112980843,21.1093059289188,49.3987736984652));
#32998=CARTESIAN_POINT('Ctrl Pts',(-15.9904109360945,20.9894835119608,48.0690557864224));
#32999=CARTESIAN_POINT('Ctrl Pts',(-12.3663152507135,20.8364792943525,45.7135099205708));
#33000=CARTESIAN_POINT('Ctrl Pts',(-8.49866891037799,20.6885792302246,42.5794650410989));
#33001=CARTESIAN_POINT('Ctrl Pts',(-5.10252178725963,20.5767478260626,39.0071711643947));
#33002=CARTESIAN_POINT('Ctrl Pts',(-2.20917801324067,20.4944756050622,35.0631014711985));
#33003=CARTESIAN_POINT('Ctrl Pts',(0.265331834530177,20.4308554028779,30.8572109582053));
#33004=CARTESIAN_POINT('Ctrl Pts',(2.19565922030913,20.3836340081555,26.3686156145749));
#33005=CARTESIAN_POINT('Ctrl Pts',(3.55122733547804,20.340580727313,21.6644068254319));
#33006=CARTESIAN_POINT('Ctrl Pts',(4.30524135296048,20.3004356869138,17.5151329967541));
#33007=CARTESIAN_POINT('Ctrl Pts',(4.52688653784348,20.2673681898868,14.6914125247235));
#33008=CARTESIAN_POINT('Ctrl Pts',(4.57736918620936,20.2421246596599,12.8192708069574));
#33009=CARTESIAN_POINT('Ctrl Pts',(4.58218835934103,20.2357981340653,12.3687776821398));
#33010=CARTESIAN_POINT('Ctrl Pts',(4.57972725339752,20.2292648564311,11.9189947438633));
#33011=CARTESIAN_POINT('Ctrl Pts',(-21.7245808409968,21.3428689572265,50.5236748853477));
#33012=CARTESIAN_POINT('Ctrl Pts',(-21.3041387087102,21.323266505305,50.3558195556542));
#33013=CARTESIAN_POINT('Ctrl Pts',(-20.8850843833989,21.303930781031,50.180587353719));
#33014=CARTESIAN_POINT('Ctrl Pts',(-19.1087003760649,21.2228186866547,49.4034447585614));
#33015=CARTESIAN_POINT('Ctrl Pts',(-16.4837535272471,21.1072213437662,48.0835031545822));
#33016=CARTESIAN_POINT('Ctrl Pts',(-12.8391736157711,20.9604400919523,45.7406026391106));
#33017=CARTESIAN_POINT('Ctrl Pts',(-8.94572887548127,20.819779963638,42.6187594657614));
#33018=CARTESIAN_POINT('Ctrl Pts',(-5.52168169435916,20.7152993064879,39.055238489401));
#33019=CARTESIAN_POINT('Ctrl Pts',(-2.59874401318366,20.6406553883908,35.1161518300549));
#33020=CARTESIAN_POINT('Ctrl Pts',(-0.0935133882118095,20.5849601975755,
30.912023564341));
#33021=CARTESIAN_POINT('Ctrl Pts',(1.8686749135023,20.5461109852346,26.4209236529955));
#33022=CARTESIAN_POINT('Ctrl Pts',(3.25684131524749,20.5119420676311,21.7095802099905));
#33023=CARTESIAN_POINT('Ctrl Pts',(4.03911612791383,20.4797911688045,17.5508438837181));
#33024=CARTESIAN_POINT('Ctrl Pts',(4.27970845737112,20.4522911786996,14.7184653460843));
#33025=CARTESIAN_POINT('Ctrl Pts',(4.34267005657433,20.4307901345004,12.839806484766));
#33026=CARTESIAN_POINT('Ctrl Pts',(4.35048498829163,20.4253683033402,12.3877080831818));
#33027=CARTESIAN_POINT('Ctrl Pts',(4.3510077184132,20.4197421663948,11.9362847456263));
#33028=CARTESIAN_POINT('',(20.8964130901555,-3.27137079310494,41.9595781864667));
#33029=CARTESIAN_POINT('Ctrl Pts',(20.8964126143753,-3.27137063675447,41.9595776658638));
#33030=CARTESIAN_POINT('Ctrl Pts',(21.1817218893114,-3.25992113527386,41.237174740169));
#33031=CARTESIAN_POINT('Ctrl Pts',(21.4383847013129,-3.24789097083339,40.506795170327));
#33032=CARTESIAN_POINT('Ctrl Pts',(21.666400175533,-3.23555894847836,39.7701345246277));
#33033=CARTESIAN_POINT('Ctrl Pts',(22.2248182238258,-3.20535738484082,37.9660262664815));
#33034=CARTESIAN_POINT('Ctrl Pts',(22.6114159538701,-3.17334534500276,36.1242455215656));
#33035=CARTESIAN_POINT('Ctrl Pts',(22.8263278926835,-3.14345008158506,34.2697199800252));
#33036=CARTESIAN_POINT('Ctrl Pts',(22.9696025185028,-3.12351990598109,33.0333696194841));
#33037=CARTESIAN_POINT('Ctrl Pts',(23.0365723482865,-3.10453051989494,31.7913549048711));
#33038=CARTESIAN_POINT('Ctrl Pts',(23.0273212361039,-3.08752071373526,30.5510624649799));
#33039=CARTESIAN_POINT('Ctrl Pts',(23.0180701239261,-3.07051090758448,29.310770025738));
#33040=CARTESIAN_POINT('Ctrl Pts',(22.9325980698661,-3.0554806813514,28.0721998612096));
#33041=CARTESIAN_POINT('Ctrl Pts',(22.7710068479441,-3.04339100491456,26.842736737895));
#33042=CARTESIAN_POINT('Ctrl Pts',(22.5286200153623,-3.02525649028182,24.9985420552148));
#33043=CARTESIAN_POINT('Ctrl Pts',(22.1149650555836,-3.01373821257335,23.1748382152102));
#33044=CARTESIAN_POINT('Ctrl Pts',(21.5304984053267,-3.01128625574909,21.396513212607));
#33045=CARTESIAN_POINT('Ctrl Pts',(21.1408539727369,-3.00965161787009,20.2109632136553));
#33046=CARTESIAN_POINT('Ctrl Pts',(20.6752932336029,-3.01204645592803,19.0455815867227));
#33047=CARTESIAN_POINT('Ctrl Pts',(20.133973937495,-3.01891855380822,17.9077259948654));
#33048=CARTESIAN_POINT('Ctrl Pts',(19.5926547062943,-3.02579065086441,16.769870539443));
#33049=CARTESIAN_POINT('Ctrl Pts',(18.97557693629,-3.03714000665748,15.6595411124551));
#33050=CARTESIAN_POINT('Ctrl Pts',(18.2829028015464,-3.05321938564873,14.5840810598834));
#33051=CARTESIAN_POINT('Ctrl Pts',(17.9974751370287,-3.05984515577954,14.1409202203334));
#33052=CARTESIAN_POINT('Ctrl Pts',(17.6992113166365,-3.06727406915266,13.703680165412));
#33053=CARTESIAN_POINT('Ctrl Pts',(17.3881232046069,-3.07550335254719,13.2728733070379));
#33054=CARTESIAN_POINT('Ctrl Pts',(20.8964126457139,-3.2713711968523,41.9595783997524));
#33055=CARTESIAN_POINT('Ctrl Pts',(17.2051685289687,1.76302070836308,43.7978652212161));
#33056=CARTESIAN_POINT('Ctrl Pts',(12.2598686672308,6.26298698655195,45.6247956227673));
#33057=CARTESIAN_POINT('Ctrl Pts',(3.58378438842023,12.5188402359751,46.8259364130367));
#33058=CARTESIAN_POINT('Ctrl Pts',(0.582129726745584,14.4577038460462,46.9709992271213));
#33059=CARTESIAN_POINT('Ctrl Pts',(-5.33701510283081,17.8486390793514,46.6585370539501));
#33060=CARTESIAN_POINT('Ctrl Pts',(-8.30844082698423,19.3555621015299,46.2345691905119));
#33061=CARTESIAN_POINT('Ctrl Pts',(-11.284173078362,20.5529756002005,45.4965192546307));
#33062=CARTESIAN_POINT('Ctrl Pts',(-21.7707507075119,21.2883239772394,50.5183817307192));
#33063=CARTESIAN_POINT('Ctrl Pts',(-21.3522076240192,21.2711623310641,50.3520726044098));
#33064=CARTESIAN_POINT('Ctrl Pts',(-20.9350453013657,21.2542807820542,50.1784403181166));
#33065=CARTESIAN_POINT('Ctrl Pts',(-19.1614547553146,21.1834525291307,49.4060644176876));
#33066=CARTESIAN_POINT('Ctrl Pts',(-16.5379429433396,21.0834264338425,48.0919810552141));
#33067=CARTESIAN_POINT('Ctrl Pts',(-12.8944921326136,20.9598507183575,45.7566603943191));
#33068=CARTESIAN_POINT('Ctrl Pts',(-9.00132135085463,20.8461335954997,42.6421286282473));
#33069=CARTESIAN_POINT('Ctrl Pts',(-5.57643150485377,20.7684839093916,39.0838481962268));
#33070=CARTESIAN_POINT('Ctrl Pts',(-2.6518075273083,20.7206230093664,35.1477051131834));
#33071=CARTESIAN_POINT('Ctrl Pts',(-0.144357875366567,20.6916936542703,
30.9445642263901));
#33072=CARTESIAN_POINT('Ctrl Pts',(1.82053721598537,20.6796111419738,26.4518611209923));
#33073=CARTESIAN_POINT('Ctrl Pts',(3.21164056637826,20.6722203558656,21.7361128259805));
#33074=CARTESIAN_POINT('Ctrl Pts',(3.99646962984073,20.6630225594897,17.5715878573721));
#33075=CARTESIAN_POINT('Ctrl Pts',(4.23871507783227,20.6508204531822,14.7339475749565));
#33076=CARTESIAN_POINT('Ctrl Pts',(4.30264169687323,20.6394053700742,12.8537551580576));
#33077=CARTESIAN_POINT('Ctrl Pts',(4.31069886437243,20.6364191357732,12.403140363483));
#33078=CARTESIAN_POINT('Ctrl Pts',(4.31153534930859,20.6332209087108,11.9532190478412));
#33079=CARTESIAN_POINT('Ctrl Pts',(-21.2368317850234,21.2398788304839,50.5241377112808));
#33080=CARTESIAN_POINT('Ctrl Pts',(-20.8200215229436,21.2217224127637,50.3562407150369));
#33081=CARTESIAN_POINT('Ctrl Pts',(-20.4046183737684,21.2038412173392,50.1810308199636));
#33082=CARTESIAN_POINT('Ctrl Pts',(-18.6386486286545,21.1287309618461,49.4019675760705));
#33083=CARTESIAN_POINT('Ctrl Pts',(-16.0274699089574,21.0222253289507,48.0782465856348));
#33084=CARTESIAN_POINT('Ctrl Pts',(-12.4043187325921,20.8890564489947,45.7304459674085));
#33085=CARTESIAN_POINT('Ctrl Pts',(-8.5367091551944,20.7641817659416,42.6038549902468));
#33086=CARTESIAN_POINT('Ctrl Pts',(-5.1394481455897,20.6752847595175,39.0368823073392));
#33087=CARTESIAN_POINT('Ctrl Pts',(-2.24410526599034,20.6159219251614,35.0957729594708));
#33088=CARTESIAN_POINT('Ctrl Pts',(0.232973273656757,20.5752144761384,30.8908341256496));
#33089=CARTESIAN_POINT('Ctrl Pts',(2.16640899202804,20.5509334123338,26.4005312505802));
#33090=CARTESIAN_POINT('Ctrl Pts',(3.52537408730755,20.5308579865904,21.6917378372941));
#33091=CARTESIAN_POINT('Ctrl Pts',(4.28238402432898,20.510426256151,17.5364645633748));
#33092=CARTESIAN_POINT('Ctrl Pts',(4.50600998813618,20.4905046142392,14.7073007255026));
#33093=CARTESIAN_POINT('Ctrl Pts',(4.55770179730602,20.4739374093561,12.8334827801716));
#33094=CARTESIAN_POINT('Ctrl Pts',(4.56283498494982,20.469713411733,12.3844319227925));
#33095=CARTESIAN_POINT('Ctrl Pts',(4.5607603471881,20.4652767483487,11.936108840748));
#33096=CARTESIAN_POINT('Ctrl Pts',(-20.7026953550296,21.1822016013635,50.5298372191554));
#33097=CARTESIAN_POINT('Ctrl Pts',(-20.2876361428746,21.1630886105529,50.360345202981));
#33098=CARTESIAN_POINT('Ctrl Pts',(-19.8740110101105,21.1442460408093,50.1835506652342));
#33099=CARTESIAN_POINT('Ctrl Pts',(-18.1157451993227,21.0650173413637,49.3977706957327));
#33100=CARTESIAN_POINT('Ctrl Pts',(-15.5170269909309,20.9522796229575,48.0643704677906));
#33101=CARTESIAN_POINT('Ctrl Pts',(-11.914371579572,20.8098799445818,45.7040379574521));
#33102=CARTESIAN_POINT('Ctrl Pts',(-8.07256301685713,20.6742608619688,42.5653401166904));
#33103=CARTESIAN_POINT('Ctrl Pts',(-4.70319179318808,20.5745198093833,38.9896454840175));
#33104=CARTESIAN_POINT('Ctrl Pts',(-1.83741971061299,20.5040526001987,35.0435609972412));
#33105=CARTESIAN_POINT('Ctrl Pts',(0.608966176495263,20.4519664047462,30.8368346587396));
#33106=CARTESIAN_POINT('Ctrl Pts',(2.51057796417895,20.4158956934967,26.3489677971651));
#33107=CARTESIAN_POINT('Ctrl Pts',(3.83699263811829,20.3835681705302,21.6471901234823));
#33108=CARTESIAN_POINT('Ctrl Pts',(4.56579136351948,20.3523071857454,17.5012346735257));
#33109=CARTESIAN_POINT('Ctrl Pts',(4.77051650292995,20.3249607749065,14.6805961850593));
#33110=CARTESIAN_POINT('Ctrl Pts',(4.80978218635625,20.3034475984546,12.8131842367604));
#33111=CARTESIAN_POINT('Ctrl Pts',(4.81194485833614,20.2980359714688,12.3657068298895));
#33112=CARTESIAN_POINT('Ctrl Pts',(4.80691198455189,20.29241155197,11.9189933731304));
#33113=CARTESIAN_POINT('Ctrl Pts',(-18.7931495275701,20.942701117012,50.5499825156838));
#33114=CARTESIAN_POINT('Ctrl Pts',(-18.3844104556852,20.9203083949833,50.374767548075));
#33115=CARTESIAN_POINT('Ctrl Pts',(-17.9772051846334,20.898168919688,50.1922871944566));
#33116=CARTESIAN_POINT('Ctrl Pts',(-16.2467663305493,20.8048139743737,49.3824073503764));
#33117=CARTESIAN_POINT('Ctrl Pts',(-13.6930315374653,20.6706999592586,48.0142800257256));
#33118=CARTESIAN_POINT('Ctrl Pts',(-10.1643218718747,20.496623371127,45.6089923970645));
#33119=CARTESIAN_POINT('Ctrl Pts',(-6.41557697784693,20.3241023157428,42.4268731843061));
#33120=CARTESIAN_POINT('Ctrl Pts',(-3.14681387909189,20.1870685788371,38.8199146290123));
#33121=CARTESIAN_POINT('Ctrl Pts',(-0.387764824647273,20.0783595881962,
34.8560273198493));
#33122=CARTESIAN_POINT('Ctrl Pts',(1.94777122640899,19.9870599496472,30.6429562278427));
#33123=CARTESIAN_POINT('Ctrl Pts',(3.73433174589954,19.9103458023656,26.1639249023865));
#33124=CARTESIAN_POINT('Ctrl Pts',(4.9429249685331,19.8358125374395,21.4874335311705));
#33125=CARTESIAN_POINT('Ctrl Pts',(5.56948361862012,19.767331746443,17.3750052192677));
#33126=CARTESIAN_POINT('Ctrl Pts',(5.70564434247915,19.7145309927478,14.5849983059168));
#33127=CARTESIAN_POINT('Ctrl Pts',(5.69981136771872,19.6760973304852,12.7405833232543));
#33128=CARTESIAN_POINT('Ctrl Pts',(5.69118929611297,19.6666248028076,12.298763756689));
#33129=CARTESIAN_POINT('Ctrl Pts',(5.67541272468907,19.6569408091057,11.8578469720222));
#33130=CARTESIAN_POINT('Ctrl Pts',(-16.0729951996959,20.4780024533914,50.577823881251));
#33131=CARTESIAN_POINT('Ctrl Pts',(-15.6734865422844,20.4514551579611,50.3943799261068));
#33132=CARTESIAN_POINT('Ctrl Pts',(-15.2756635218504,20.4251375618498,50.2037236209258));
#33133=CARTESIAN_POINT('Ctrl Pts',(-13.585918711749,20.3138746691076,49.3591889780907));
#33134=CARTESIAN_POINT('Ctrl Pts',(-11.0979122802499,20.1526659052326,47.9411348740909));
#33135=CARTESIAN_POINT('Ctrl Pts',(-7.67711842462297,19.938389785095,45.4712448274525));
#33136=CARTESIAN_POINT('Ctrl Pts',(-4.06407758685823,19.7189203495023,42.2267652427763));
#33137=CARTESIAN_POINT('Ctrl Pts',(-0.941922279639655,19.5342279169114,
38.5749629248337));
#33138=CARTESIAN_POINT('Ctrl Pts',(1.66165202444,19.3763677050182,34.5856193142543));
#33139=CARTESIAN_POINT('Ctrl Pts',(3.83571038720547,19.2344308170631,30.3635908493067));
#33140=CARTESIAN_POINT('Ctrl Pts',(5.45465393399974,19.1049298841923,25.8974565196366));
#33141=CARTESIAN_POINT('Ctrl Pts',(6.49153137845572,18.9752993129734,21.2575392892134));
#33142=CARTESIAN_POINT('Ctrl Pts',(6.96902001911252,18.8580619466085,17.1935174826788));
#33143=CARTESIAN_POINT('Ctrl Pts',(7.00515567331294,18.7718242877839,14.4476953676603));
#33144=CARTESIAN_POINT('Ctrl Pts',(6.93350774385575,18.7111415689428,12.6364417245434));
#33145=CARTESIAN_POINT('Ctrl Pts',(6.90914089038382,18.6963263828107,12.2028004749143));
#33146=CARTESIAN_POINT('Ctrl Pts',(6.87767405528031,18.6812985797984,11.7702816402821));
#33147=CARTESIAN_POINT('Ctrl Pts',(-12.1032860351762,19.4355555088431,50.6164198137043));
#33148=CARTESIAN_POINT('Ctrl Pts',(-11.7178979337882,19.4044605226273,50.4206764214417));
#33149=CARTESIAN_POINT('Ctrl Pts',(-11.3344425025602,19.3735658358572,50.2178005709574));
#33150=CARTESIAN_POINT('Ctrl Pts',(-9.70707833240668,19.2426748194849,49.3214781077038));
#33151=CARTESIAN_POINT('Ctrl Pts',(-7.31971757114185,19.0517849995255,47.8288402064322));
#33152=CARTESIAN_POINT('Ctrl Pts',(-4.06391667596133,18.7933185397158,45.2625228787868));
#33153=CARTESIAN_POINT('Ctrl Pts',(-0.65815408706669,18.5218580841843,41.9250672284237));
#33154=CARTESIAN_POINT('Ctrl Pts',(2.24021981970534,18.2836948825759,38.2065612420059));
#33155=CARTESIAN_POINT('Ctrl Pts',(4.60650328315228,18.0697821020849,34.1795723756759));
#33156=CARTESIAN_POINT('Ctrl Pts',(6.53406799563972,17.8693333343866,29.9446179095315));
#33157=CARTESIAN_POINT('Ctrl Pts',(7.89702239493376,17.6778661310593,25.4982889661853));
#33158=CARTESIAN_POINT('Ctrl Pts',(8.6714190430009,17.4826662284719,20.9136218061456));
#33159=CARTESIAN_POINT('Ctrl Pts',(8.92083514113572,17.3068805329357,16.9224847476292));
#33160=CARTESIAN_POINT('Ctrl Pts',(8.80376329647722,17.1802068447994,14.2430779026764));
#33161=CARTESIAN_POINT('Ctrl Pts',(8.63123896138171,17.0925519552341,12.4816401372632));
#33162=CARTESIAN_POINT('Ctrl Pts',(8.58273039837833,17.0712544126695,12.0603344267302));
#33163=CARTESIAN_POINT('Ctrl Pts',(8.52719757288954,17.0497370990139,11.6405300048787));
#33164=CARTESIAN_POINT('Ctrl Pts',(-7.62272160330697,17.8320672383652,50.6581802616326));
#33165=CARTESIAN_POINT('Ctrl Pts',(-7.25398775498929,17.7976045693245,50.4481370270082));
#33166=CARTESIAN_POINT('Ctrl Pts',(-6.88750202682987,17.7633163796081,50.2310564733353));
#33167=CARTESIAN_POINT('Ctrl Pts',(-5.33391956582982,17.6178640028275,49.2745483347903));
#33168=CARTESIAN_POINT('Ctrl Pts',(-3.06553206003439,17.4049846203341,47.6952600514936));
#33169=CARTESIAN_POINT('Ctrl Pts',(-0.00463583136575324,17.1135517229592,
45.0169995840933));
#33170=CARTESIAN_POINT('Ctrl Pts',(3.15635102645389,16.8027253827761,41.5717186110543));
#33171=CARTESIAN_POINT('Ctrl Pts',(5.7904790976245,16.523022337621,37.7760221244729));
#33172=CARTESIAN_POINT('Ctrl Pts',(7.87647490362216,16.2641978724915,33.7057056652031));
#33173=CARTESIAN_POINT('Ctrl Pts',(9.51275839490381,16.0157341831644,29.4562199413809));
#33174=CARTESIAN_POINT('Ctrl Pts',(10.572992548482,15.7719994721116,25.0334778672443));
#33175=CARTESIAN_POINT('Ctrl Pts',(11.0366764891831,15.5202180684676,20.5136585803792));
#33176=CARTESIAN_POINT('Ctrl Pts',(11.0158502606114,15.2931736272884,16.6078147103202));
#33177=CARTESIAN_POINT('Ctrl Pts',(10.7170384335309,15.130708702949,14.0060109473856));
#33178=CARTESIAN_POINT('Ctrl Pts',(10.424772847932,15.0190926843839,12.3027493029688));
#33179=CARTESIAN_POINT('Ctrl Pts',(10.3476075850064,14.9920326361705,11.8959214149251));
#33180=CARTESIAN_POINT('Ctrl Pts',(10.2635094955229,14.9647422323135,11.4911075898942));
#33181=CARTESIAN_POINT('Ctrl Pts',(-3.35795326833651,15.7638142683891,50.6963817466487));
#33182=CARTESIAN_POINT('Ctrl Pts',(-3.00594729840862,15.7283726072843,50.4720971928266));
#33183=CARTESIAN_POINT('Ctrl Pts',(-2.65653363487031,15.6930928161318,50.2408753340372));
#33184=CARTESIAN_POINT('Ctrl Pts',(-1.17729495989077,15.543379415412,49.2244801690097));
#33185=CARTESIAN_POINT('Ctrl Pts',(0.971223374172476,15.3241289383934,47.55900262026));
#33186=CARTESIAN_POINT('Ctrl Pts',(3.8357234634446,15.0227233638938,44.7694897092564));
#33187=CARTESIAN_POINT('Ctrl Pts',(6.74997776965196,14.6988957424381,41.2171739295578));
#33188=CARTESIAN_POINT('Ctrl Pts',(9.11758018092376,14.4035050799014,37.3450408571422));
#33189=CARTESIAN_POINT('Ctrl Pts',(10.9206141805866,14.1252237593235,33.2320880582171));
#33190=CARTESIAN_POINT('Ctrl Pts',(12.2625916131558,13.8539516979883,28.9686983169118));
#33191=CARTESIAN_POINT('Ctrl Pts',(13.0165992412534,13.5829362127958,24.5700729333908));
#33192=CARTESIAN_POINT('Ctrl Pts',(13.1655210239449,13.2994842764397,20.115507858));
#33193=CARTESIAN_POINT('Ctrl Pts',(12.8705817285104,13.0425486753816,16.295208978186));
#33194=CARTESIAN_POINT('Ctrl Pts',(12.3871650850191,12.8585920936854,13.7711041013664));
#33195=CARTESIAN_POINT('Ctrl Pts',(11.9731744450198,12.7324540777387,12.1260554282844));
#33196=CARTESIAN_POINT('Ctrl Pts',(11.8668941925931,12.7018988467546,11.733793887101));
#33197=CARTESIAN_POINT('Ctrl Pts',(11.7537921409323,12.6711030837425,11.3441365131014));
#33198=CARTESIAN_POINT('Ctrl Pts',(0.649628458040476,13.2592937677246,50.7317627733558));
#33199=CARTESIAN_POINT('Ctrl Pts',(0.985066924078268,13.2252177231213,50.4932939999314));
#33200=CARTESIAN_POINT('Ctrl Pts',(1.31754402223974,13.191306123502,50.2479943303873));
#33201=CARTESIAN_POINT('Ctrl Pts',(2.72290890156926,13.0474600457288,49.1720182643306));
#33202=CARTESIAN_POINT('Ctrl Pts',(4.7522202374985,12.8372075593629,47.4208175921215));
#33203=CARTESIAN_POINT('Ctrl Pts',(7.42110856617907,12.5484949329477,44.5207322457509));
#33204=CARTESIAN_POINT('Ctrl Pts',(10.0892640390092,12.2377054846042,40.8621397595677));
#33205=CARTESIAN_POINT('Ctrl Pts',(12.1905795141142,11.9522310106351,36.9142683953372));
#33206=CARTESIAN_POINT('Ctrl Pts',(13.7104379500398,11.6797819251771,32.7592945131865));
#33207=CARTESIAN_POINT('Ctrl Pts',(14.7575062139052,11.4108111467242,28.4825373574617));
#33208=CARTESIAN_POINT('Ctrl Pts',(15.2041645593447,11.1374939458242,24.1084517121114));
#33209=CARTESIAN_POINT('Ctrl Pts',(15.0366365526659,10.8473681096278,19.7194278841075));
#33210=CARTESIAN_POINT('Ctrl Pts',(14.4657312097101,10.5820480444149,15.9848167741326));
#33211=CARTESIAN_POINT('Ctrl Pts',(13.7961914563873,10.3910369789073,13.5384306970429));
#33212=CARTESIAN_POINT('Ctrl Pts',(13.2593802947326,10.2599216927486,11.9515813330258));
#33213=CARTESIAN_POINT('Ctrl Pts',(13.1237579689611,10.2281653805015,11.5739532609048));
#33214=CARTESIAN_POINT('Ctrl Pts',(12.9814618015971,10.1961599190035,11.1995871689857));
#33215=CARTESIAN_POINT('Ctrl Pts',(4.42912516463123,10.420684636249,50.7652541888306));
#33216=CARTESIAN_POINT('Ctrl Pts',(4.74825780617854,10.3898269637342,50.5126392026911));
#33217=CARTESIAN_POINT('Ctrl Pts',(5.06403756009174,10.3591499865554,50.2533088244876));
#33218=CARTESIAN_POINT('Ctrl Pts',(6.39645270620807,10.2291883131935,49.1179996982607));
#33219=CARTESIAN_POINT('Ctrl Pts',(8.30791494002339,10.0401067219452,47.2814499847572));
#33220=CARTESIAN_POINT('Ctrl Pts',(10.7830309301442,9.78206378055234,44.2713285475977));
#33221=CARTESIAN_POINT('Ctrl Pts',(13.2069767395828,9.50499638561923,40.507046655879));
#33222=CARTESIAN_POINT('Ctrl Pts',(15.0435435138209,9.24981780003299,36.483964634552));
#33223=CARTESIAN_POINT('Ctrl Pts',(16.2813751655171,9.00337535985762,32.2874206634502));
#33224=CARTESIAN_POINT('Ctrl Pts',(17.0343538672163,8.75677479408939,27.9976769484779));
#33225=CARTESIAN_POINT('Ctrl Pts',(17.1740502474811,8.50116890088297,23.6484132748248));
#33226=CARTESIAN_POINT('Ctrl Pts',(16.6900004076409,8.22444592813344,19.3250984247532));
#33227=CARTESIAN_POINT('Ctrl Pts',(15.8427415672468,7.96804930448713,15.6762334080315));
#33228=CARTESIAN_POINT('Ctrl Pts',(14.9865968963869,7.78162503245108,13.3075436526941));
#33229=CARTESIAN_POINT('Ctrl Pts',(14.3265730286372,7.65323614745839,11.7788572968638));
#33230=CARTESIAN_POINT('Ctrl Pts',(14.1615675750574,7.62212996336316,11.4159103189612));
#33231=CARTESIAN_POINT('Ctrl Pts',(13.9900895826365,7.59076668565169,11.0569364769952));
#33232=CARTESIAN_POINT('Ctrl Pts',(7.89549180552655,7.18298363715391,50.7967927897824));
#33233=CARTESIAN_POINT('Ctrl Pts',(8.19878346721173,7.15763661423686,50.5300854115103));
#33234=CARTESIAN_POINT('Ctrl Pts',(8.49831389186478,7.13250342173354,50.2567869804956));
#33235=CARTESIAN_POINT('Ctrl Pts',(9.75961916607793,7.02634360727853,49.0624579541012));
#33236=CARTESIAN_POINT('Ctrl Pts',(11.5559647746267,6.87350147707393,47.1410278166122));
#33237=CARTESIAN_POINT('Ctrl Pts',(13.8411235870497,6.66841421880391,44.0215306056881));
#33238=CARTESIAN_POINT('Ctrl Pts',(16.0249513960127,6.45075222930465,40.1522690131667));
#33239=CARTESIAN_POINT('Ctrl Pts',(17.6003804394465,6.25122984378583,36.0545969342759));
#33240=CARTESIAN_POINT('Ctrl Pts',(18.5592768296093,6.05595707526583,31.8169952215559));
#33241=CARTESIAN_POINT('Ctrl Pts',(19.0208253379016,5.8568061689083,27.5146808861226));
#33242=CARTESIAN_POINT('Ctrl Pts',(18.8556599138234,5.64398234710963,23.1905225310631));
#33243=CARTESIAN_POINT('Ctrl Pts',(18.0566069174411,5.40587468584602,18.9330502545293));
#33244=CARTESIAN_POINT('Ctrl Pts',(16.9338900015705,5.18017895256177,15.3699358641023));
#33245=CARTESIAN_POINT('Ctrl Pts',(15.8914626446178,5.01301666232781,13.0788676150056));
#33246=CARTESIAN_POINT('Ctrl Pts',(15.1083470249008,4.89707445701614,11.6082681357848));
#33247=CARTESIAN_POINT('Ctrl Pts',(14.9140516856407,4.86894780999335,11.2600237011743));
#33248=CARTESIAN_POINT('Ctrl Pts',(14.7135487892971,4.84055053954568,10.9165003544731));
#33249=CARTESIAN_POINT('Ctrl Pts',(11.0060924800857,3.57357815210241,50.8268930609901));
#33250=CARTESIAN_POINT('Ctrl Pts',(11.2942348360949,3.55599962931061,50.5461528505987));
#33251=CARTESIAN_POINT('Ctrl Pts',(11.5781977781179,3.53868515668548,50.2589525717582));
#33252=CARTESIAN_POINT('Ctrl Pts',(12.7712619273494,3.46609807861293,49.0059215208389));
#33253=CARTESIAN_POINT('Ctrl Pts',(14.4567798870219,3.36435917107101,47.0000807098697));
#33254=CARTESIAN_POINT('Ctrl Pts',(16.5580799000384,3.23426720235262,43.7718526676594));
#33255=CARTESIAN_POINT('Ctrl Pts',(18.5084918938618,3.10147907156715,39.7982847372331));
#33256=CARTESIAN_POINT('Ctrl Pts',(19.8289470704012,2.98285053627008,35.6265858547269));
#33257=CARTESIAN_POINT('Ctrl Pts',(20.5145093436472,2.86388130857434,31.3483637201532));
#33258=CARTESIAN_POINT('Ctrl Pts',(20.6897703805126,2.73730530568202,27.0338075077601));
#33259=CARTESIAN_POINT('Ctrl Pts',(20.2243046828408,2.59247375589619,22.7349380039858));
#33260=CARTESIAN_POINT('Ctrl Pts',(19.1142246129334,2.41842603756845,18.5433338285095));
#33261=CARTESIAN_POINT('Ctrl Pts',(17.71905778023,2.24547053120763,15.0658785351744));
#33262=CARTESIAN_POINT('Ctrl Pts',(16.492089181663,2.11246131963295,12.8522922345518));
#33263=CARTESIAN_POINT('Ctrl Pts',(15.5869422351719,2.01884144332686,11.4396612518973));
#33264=CARTESIAN_POINT('Ctrl Pts',(15.3636796831515,1.99605339732081,11.1061079698993));
#33265=CARTESIAN_POINT('Ctrl Pts',(15.1345413251225,1.9729679754383,10.7780380956973));
#33266=CARTESIAN_POINT('Ctrl Pts',(13.4086040565199,0.237308438758995,50.8518932795148));
#33267=CARTESIAN_POINT('Ctrl Pts',(13.6843431150251,0.227921876287717,50.5591653280353));
#33268=CARTESIAN_POINT('Ctrl Pts',(13.955539055312,0.218854274805993,50.2600946828327));
#33269=CARTESIAN_POINT('Ctrl Pts',(15.092550531276,0.181679983795775,48.9569680233745));
#33270=CARTESIAN_POINT('Ctrl Pts',(16.6867297894324,0.133848323063104,46.8790983035039));
#33271=CARTESIAN_POINT('Ctrl Pts',(18.6356692131024,0.0830496793456984,
43.558108432264));
#33272=CARTESIAN_POINT('Ctrl Pts',(20.391809639507,0.0403924264632703,39.4955813035581));
#33273=CARTESIAN_POINT('Ctrl Pts',(21.499121492597,0.00837005963384143,
35.2607922709484));
#33274=CARTESIAN_POINT('Ctrl Pts',(21.9553996260992,-0.0279539839125438,
30.9480199544426));
#33275=CARTESIAN_POINT('Ctrl Pts',(21.8899491514933,-0.0750512999789021,
26.6231583667432));
#33276=CARTESIAN_POINT('Ctrl Pts',(21.1713548702409,-0.14423024726241,22.3460478681646));
#33277=CARTESIAN_POINT('Ctrl Pts',(19.7985513468811,-0.245792879606331,
18.210873465606));
#33278=CARTESIAN_POINT('Ctrl Pts',(18.172904950709,-0.358291148292244,14.8067369437337));
#33279=CARTESIAN_POINT('Ctrl Pts',(16.7896161629616,-0.451704594358635,
12.659441105225));
#33280=CARTESIAN_POINT('Ctrl Pts',(15.7810380374713,-0.519340602547392,
11.2963988201152));
#33281=CARTESIAN_POINT('Ctrl Pts',(15.5332807033662,-0.535923052101836,
10.9754131301141));
#33282=CARTESIAN_POINT('Ctrl Pts',(15.2799843900674,-0.552841667182328,
10.6605612070475));
#33283=CARTESIAN_POINT('Ctrl Pts',(14.8211913517824,-2.14030259993981,50.8681119118098));
#33284=CARTESIAN_POINT('Ctrl Pts',(15.0891137342418,-2.14321532053782,50.5674285935912));
#33285=CARTESIAN_POINT('Ctrl Pts',(15.3522519677804,-2.14576465810466,50.2604798846934));
#33286=CARTESIAN_POINT('Ctrl Pts',(16.4538380030325,-2.15494826818845,48.9241050232901));
#33287=CARTESIAN_POINT('Ctrl Pts',(17.9900417596044,-2.16016260296573,46.7984325485291));
#33288=CARTESIAN_POINT('Ctrl Pts',(19.841600565389,-2.1481556077715,43.4158887130568));
#33289=CARTESIAN_POINT('Ctrl Pts',(21.4729001795181,-2.11918777525101,39.2943434845245));
#33290=CARTESIAN_POINT('Ctrl Pts',(22.4425122487173,-2.08197924289826,35.0177196733706));
#33291=CARTESIAN_POINT('Ctrl Pts',(22.7500500882429,-2.05170003121316,30.6820714739305));
#33292=CARTESIAN_POINT('Ctrl Pts',(22.5280186102684,-2.03426137368081,26.3504407431274));
#33293=CARTESIAN_POINT('Ctrl Pts',(21.6442903605272,-2.04135770257883,22.0878641606114));
#33294=CARTESIAN_POINT('Ctrl Pts',(20.0996909490575,-2.08278583441843,17.9902613908005));
#33295=CARTESIAN_POINT('Ctrl Pts',(18.3230901845701,-2.14471303148954,14.6349096946119));
#33296=CARTESIAN_POINT('Ctrl Pts',(16.8372754744228,-2.20477046252904,12.5317089640345));
#33297=CARTESIAN_POINT('Ctrl Pts',(15.7608189202074,-2.25046208753918,11.2016493161336));
#33298=CARTESIAN_POINT('Ctrl Pts',(15.4970132544121,-2.26180965939547,10.8890156234971));
#33299=CARTESIAN_POINT('Ctrl Pts',(15.2279154659668,-2.27353152926925,10.582940513715));
#33300=CARTESIAN_POINT('Ctrl Pts',(15.7277767926436,-3.83428286431684,50.8791923579944));
#33301=CARTESIAN_POINT('Ctrl Pts',(15.9904775111148,-3.83237339034492,50.5730212587592));
#33302=CARTESIAN_POINT('Ctrl Pts',(16.2482277522975,-3.83006698099443,50.2606381905767));
#33303=CARTESIAN_POINT('Ctrl Pts',(17.3261040612264,-3.81839846831683,48.9013292866715));
#33304=CARTESIAN_POINT('Ctrl Pts',(18.8234014267205,-3.79185933798401,46.7426835888032));
#33305=CARTESIAN_POINT('Ctrl Pts',(20.6093307672563,-3.73301479320489,43.3176825681743));
#33306=CARTESIAN_POINT('Ctrl Pts',(22.1562183974292,-3.65055513724086,39.1554316071207));
#33307=CARTESIAN_POINT('Ctrl Pts',(23.0324273075003,-3.56151400652134,34.8499580812955));
#33308=CARTESIAN_POINT('Ctrl Pts',(23.2388288624445,-3.48120332570528,30.4985424034584));
#33309=CARTESIAN_POINT('Ctrl Pts',(22.9101616831314,-3.41513875248544,26.1622590588885));
#33310=CARTESIAN_POINT('Ctrl Pts',(21.9137885476468,-3.37526128513496,21.9097314946167));
#33311=CARTESIAN_POINT('Ctrl Pts',(20.2518478400219,-3.37099617994084,17.8380781703545));
#33312=CARTESIAN_POINT('Ctrl Pts',(18.3720514471088,-3.39437469848804,14.516413522755));
#33313=CARTESIAN_POINT('Ctrl Pts',(16.8160965878723,-3.42893690611626,12.443658949834));
#33314=CARTESIAN_POINT('Ctrl Pts',(15.6931888427596,-3.45783930783476,11.1363723028377));
#33315=CARTESIAN_POINT('Ctrl Pts',(15.4184128726594,-3.46518513130081,10.8295005505935));
#33316=CARTESIAN_POINT('Ctrl Pts',(15.1385252299473,-3.47293757911652,10.5294756446789));
#33317=CARTESIAN_POINT('Ctrl Pts',(15.9701665800735,-4.30636894546118,50.8822308776832));
#33318=CARTESIAN_POINT('Ctrl Pts',(16.2314548017925,-4.3031084050989,50.5745495731437));
#33319=CARTESIAN_POINT('Ctrl Pts',(16.4877466093682,-4.29944065268701,50.260670552203));
#33320=CARTESIAN_POINT('Ctrl Pts',(17.5592011847449,-4.28192251284736,48.8950465059731));
#33321=CARTESIAN_POINT('Ctrl Pts',(19.0459352980637,-4.24645759656194,46.7273192303219));
#33322=CARTESIAN_POINT('Ctrl Pts',(20.8139790917651,-4.17439213330946,43.290622721956));
#33323=CARTESIAN_POINT('Ctrl Pts',(22.3377993873479,-4.07676875425951,39.1171604186841));
#33324=CARTESIAN_POINT('Ctrl Pts',(23.1884224645965,-3.97294922980807,34.8037494417951));
#33325=CARTESIAN_POINT('Ctrl Pts',(23.3670805064487,-3.87828739688684,30.4480108044923));
#33326=CARTESIAN_POINT('Ctrl Pts',(23.0091488885558,-3.79820251809058,26.1104754031575));
#33327=CARTESIAN_POINT('Ctrl Pts',(21.9818628449813,-3.74469501429227,21.8607506502009));
#33328=CARTESIAN_POINT('Ctrl Pts',(20.2877455250282,-3.72710099262819,17.7962731039455));
#33329=CARTESIAN_POINT('Ctrl Pts',(18.379688708248,-3.7392015362719,14.4838944016608));
#33330=CARTESIAN_POINT('Ctrl Pts',(16.8045486295666,-3.76629674044718,12.4195139572451));
#33331=CARTESIAN_POINT('Ctrl Pts',(15.6689453809918,-3.79028538091932,11.1184838099602));
#33332=CARTESIAN_POINT('Ctrl Pts',(15.3911733460635,-3.79646095010219,10.8131933790853));
#33333=CARTESIAN_POINT('Ctrl Pts',(15.1083410178804,-3.80305340259771,10.5148273212522));
#33334=CARTESIAN_POINT('Ctrl Pts',(16.2040281833702,-4.78145508078572,50.8852370446122));
#33335=CARTESIAN_POINT('Ctrl Pts',(16.4639362979632,-4.77682808742727,50.5760559448111));
#33336=CARTESIAN_POINT('Ctrl Pts',(16.7188024266086,-4.7717826224726,50.260690536201));
#33337=CARTESIAN_POINT('Ctrl Pts',(17.7839765354645,-4.74834091216943,48.8887884576835));
#33338=CARTESIAN_POINT('Ctrl Pts',(19.2603541657225,-4.70381966688121,46.7120309167521));
#33339=CARTESIAN_POINT('Ctrl Pts',(21.0107955623606,-4.61828583278682,43.2637031873351));
#33340=CARTESIAN_POINT('Ctrl Pts',(22.5118507531063,-4.50515190400754,39.0790928379428));
#33341=CARTESIAN_POINT('Ctrl Pts',(23.3371620822167,-4.38613315046716,34.7577977729984));
#33342=CARTESIAN_POINT('Ctrl Pts',(23.488334854988,-4.27662792828432,30.3977805929722));
#33343=CARTESIAN_POINT('Ctrl Pts',(23.1013992673138,-4.18197237106197,26.0590299164957));
#33344=CARTESIAN_POINT('Ctrl Pts',(22.0434765995787,-4.11421750462538,21.8121276651408));
#33345=CARTESIAN_POINT('Ctrl Pts',(20.3174958444881,-4.08262421860679,17.7548145479695));
#33346=CARTESIAN_POINT('Ctrl Pts',(18.3814912904369,-4.0828488851085,14.4516774578153));
#33347=CARTESIAN_POINT('Ctrl Pts',(16.7874012762348,-4.10207414795096,12.3956126071312));
#33348=CARTESIAN_POINT('Ctrl Pts',(15.639268392688,-4.12088738197538,11.1007880383459));
#33349=CARTESIAN_POINT('Ctrl Pts',(15.3585405257443,-4.12583098108427,10.7970646604656));
#33350=CARTESIAN_POINT('Ctrl Pts',(15.0728040607247,-4.13120272145022,10.5003411970122));
#33351=CARTESIAN_POINT('Ctrl Pts',(-11.2641171037461,20.7105311502992,45.5014889049172));
#33352=CARTESIAN_POINT('Ctrl Pts',(-8.19359489044161,19.964194825681,46.2616123376652));
#33353=CARTESIAN_POINT('Ctrl Pts',(-5.14011995665627,18.7336174305176,46.6827377201639));
#33354=CARTESIAN_POINT('Ctrl Pts',(1.02851041262146,15.6437709209759,46.9777867249755));
#33355=CARTESIAN_POINT('Ctrl Pts',(4.2178450202458,13.6706054870974,46.7792896653727));
#33356=CARTESIAN_POINT('Ctrl Pts',(9.98319411871419,9.45712578824497,45.8889713600162));
#33357=CARTESIAN_POINT('Ctrl Pts',(12.6385843053104,7.18268858965248,45.2073292047804));
#33358=CARTESIAN_POINT('Ctrl Pts',(17.2824959903431,2.26699035497259,43.6397205033547));
#33359=CARTESIAN_POINT('Ctrl Pts',(19.2859044761697,-0.365223927781814,
42.7616321300472));
#33360=CARTESIAN_POINT('Ctrl Pts',(20.8964136033761,-3.27137043593021,41.9595779228243));
#33361=CARTESIAN_POINT('Ctrl Pts',(-53.0706963107889,21.2883239772394,14.476633177513));
#33362=CARTESIAN_POINT('Ctrl Pts',(-52.6797132558222,21.2711623310641,14.7001712927468));
#33363=CARTESIAN_POINT('Ctrl Pts',(-52.2838656141311,21.2542807820542,14.9180639701196));
#33364=CARTESIAN_POINT('Ctrl Pts',(-50.5741822007401,21.1834525291307,15.8231443989111));
#33365=CARTESIAN_POINT('Ctrl Pts',(-47.9110575975486,21.0834264338425,17.0549709528455));
#33366=CARTESIAN_POINT('Ctrl Pts',(-43.8135759591412,20.9598507183575,18.4474868853566));
#33367=CARTESIAN_POINT('Ctrl Pts',(-38.9511846919585,20.8461335954997,19.5494115754497));
#33368=CARTESIAN_POINT('Ctrl Pts',(-34.0338251352838,20.7684839093916,20.0085467195199));
#33369=CARTESIAN_POINT('Ctrl Pts',(-29.1329513291906,20.7206230093664,19.8409647486116));
#33370=CARTESIAN_POINT('Ctrl Pts',(-24.2834341719871,20.6916936542703,19.180752348512));
#33371=CARTESIAN_POINT('Ctrl Pts',(-19.545805391625,20.6796111419738,17.9158146216833));
#33372=CARTESIAN_POINT('Ctrl Pts',(-14.9915461588884,20.6722203558656,16.0632020463146));
#33373=CARTESIAN_POINT('Ctrl Pts',(-11.2462565116349,20.6630225594897,14.0802672689721));
#33374=CARTESIAN_POINT('Ctrl Pts',(-8.87666243655348,20.6508204531822,12.5004226092667));
#33375=CARTESIAN_POINT('Ctrl Pts',(-7.36681121688492,20.6394053700742,11.3781216551321));
#33376=CARTESIAN_POINT('Ctrl Pts',(-7.00948282225308,20.6364191357732,11.1034672733586));
#33377=CARTESIAN_POINT('Ctrl Pts',(-6.65719863322378,20.6332209087108,10.8235999116748));
#33378=CARTESIAN_POINT('Ctrl Pts',(-52.7423035144133,21.2398788304839,14.8976565953797));
#33379=CARTESIAN_POINT('Ctrl Pts',(-52.3511594092213,21.2217224127637,15.1188499155687));
#33380=CARTESIAN_POINT('Ctrl Pts',(-51.9551751700423,21.2038412173392,15.3343835927472));
#33381=CARTESIAN_POINT('Ctrl Pts',(-50.2450148726635,21.1287309618461,16.229336348993));
#33382=CARTESIAN_POINT('Ctrl Pts',(-47.5820448257753,21.0222253289507,17.4455115403598));
#33383=CARTESIAN_POINT('Ctrl Pts',(-43.4874625788319,20.8890564489947,18.8143754535216));
#33384=CARTESIAN_POINT('Ctrl Pts',(-38.6315801910077,20.7641817659416,19.8887967941821));
#33385=CARTESIAN_POINT('Ctrl Pts',(-33.7246510566663,20.6752847595175,20.3209113143506));
#33386=CARTESIAN_POINT('Ctrl Pts',(-28.8381509343392,20.6159219251614,20.127340043755));
#33387=CARTESIAN_POINT('Ctrl Pts',(-24.0061641643323,20.5752144761384,19.4422615502697));
#33388=CARTESIAN_POINT('Ctrl Pts',(-19.2900265578325,20.5509334123338,18.1542244143579));
#33389=CARTESIAN_POINT('Ctrl Pts',(-14.7612427448985,20.5308579865904,16.2808214371791));
#33390=CARTESIAN_POINT('Ctrl Pts',(-11.0405313054518,20.510426256151,14.2819051282588));
#33391=CARTESIAN_POINT('Ctrl Pts',(-8.68917344007867,20.4905046142392,12.6927881463597));
#33392=CARTESIAN_POINT('Ctrl Pts',(-7.19193426214825,20.4739374093561,11.5648960507006));
#33393=CARTESIAN_POINT('Ctrl Pts',(-6.8376516744731,20.469713411733,11.2889307083142));
#33394=CARTESIAN_POINT('Ctrl Pts',(-6.48843209010061,20.4652767483487,11.0077838216047));
#33395=CARTESIAN_POINT('Ctrl Pts',(-52.413730952202,21.1822016013635,15.3188148573173));
#33396=CARTESIAN_POINT('Ctrl Pts',(-52.0224315719836,21.1630886105529,15.5376446728873));
#33397=CARTESIAN_POINT('Ctrl Pts',(-51.6263169843739,21.1442460408093,15.7508002323129));
#33398=CARTESIAN_POINT('Ctrl Pts',(-49.9157086639418,21.0650173413637,16.6355420002449));
#33399=CARTESIAN_POINT('Ctrl Pts',(-47.2529400861698,20.9522796229575,17.8359402657105));
#33400=CARTESIAN_POINT('Ctrl Pts',(-43.1613389119008,20.8098799445818,19.180966437603));
#33401=CARTESIAN_POINT('Ctrl Pts',(-38.3120776664927,20.6742608619688,20.2276672267179));
#33402=CARTESIAN_POINT('Ctrl Pts',(-33.4157184343431,20.5745198093833,20.6325385874716));
#33403=CARTESIAN_POINT('Ctrl Pts',(-28.5437656821657,20.5040526001987,20.4127459884288));
#33404=CARTESIAN_POINT('Ctrl Pts',(-23.7295179405745,20.4519664047462,19.7025565219692));
#33405=CARTESIAN_POINT('Ctrl Pts',(-19.0351267823555,20.4158956934967,18.3911572647212));
#33406=CARTESIAN_POINT('Ctrl Pts',(-14.5321229512679,20.3835681705302,16.4966795854662));
#33407=CARTESIAN_POINT('Ctrl Pts',(-10.8362858826867,20.3523071857454,14.4815164313589));
#33408=CARTESIAN_POINT('Ctrl Pts',(-8.50337787513608,20.3249607749065,12.8829376583136));
#33409=CARTESIAN_POINT('Ctrl Pts',(-7.01889467003979,20.3034475984546,11.7493245001634));
#33410=CARTESIAN_POINT('Ctrl Pts',(-6.66769434173069,20.2980359714688,11.4720177454573));
#33411=CARTESIAN_POINT('Ctrl Pts',(-6.32157764307285,20.29241155197,11.1895616016432));
#33412=CARTESIAN_POINT('Ctrl Pts',(-51.2388988296486,20.942701117012,16.8243182893816));
#33413=CARTESIAN_POINT('Ctrl Pts',(-50.8470656088309,20.9203083949833,17.0346386184588));
#33414=CARTESIAN_POINT('Ctrl Pts',(-50.4505083896763,20.898168919688,17.2392298796734));
#33415=CARTESIAN_POINT('Ctrl Pts',(-48.7384078522966,20.8048139743737,18.0871896307673));
#33416=CARTESIAN_POINT('Ctrl Pts',(-46.0765352377201,20.6706999592586,19.2307664553104));
#33417=CARTESIAN_POINT('Ctrl Pts',(-41.995891155026,20.496623371127,20.4899504573511));
#33418=CARTESIAN_POINT('Ctrl Pts',(-37.1707059623287,20.3241023157428,21.4368183577897));
#33419=CARTESIAN_POINT('Ctrl Pts',(-32.3126317510767,20.1870685788371,21.7435383821734));
#33420=CARTESIAN_POINT('Ctrl Pts',(-27.4933009115434,20.0783595881962,21.4292064816315));
#33421=CARTESIAN_POINT('Ctrl Pts',(-22.7432063842296,19.9870599496472,20.6283952344143));
#33422=CARTESIAN_POINT('Ctrl Pts',(-18.1274564187216,19.9103458023656,19.2325541402588));
#33423=CARTESIAN_POINT('Ctrl Pts',(-13.7176826883073,19.8358125374395,17.2617256927776));
#33424=CARTESIAN_POINT('Ctrl Pts',(-10.1118038360732,19.767331746443,15.1875318576818));
#33425=CARTESIAN_POINT('Ctrl Pts',(-7.84559377217224,19.7145309927478,13.5544457406808));
#33426=CARTESIAN_POINT('Ctrl Pts',(-6.40720887226862,19.6760973304852,12.3999114052912));
#33427=CARTESIAN_POINT('Ctrl Pts',(-6.06715619927451,19.6666248028076,12.1177004042506));
#33428=CARTESIAN_POINT('Ctrl Pts',(-5.73227010726454,19.6569408091057,11.8304586653179));
#33429=CARTESIAN_POINT('Ctrl Pts',(-49.5646776028525,20.4780024533914,18.9683793875862));
#33430=CARTESIAN_POINT('Ctrl Pts',(-49.172165769802,20.4514551579611,19.166352398224));
#33431=CARTESIAN_POINT('Ctrl Pts',(-48.7750660718952,20.4251375618498,19.3585106981095));
#33432=CARTESIAN_POINT('Ctrl Pts',(-47.0612436432498,20.3138746691076,20.1530476508596));
#33433=CARTESIAN_POINT('Ctrl Pts',(-44.4013176639012,20.1526659052326,21.2141071352607));
#33434=CARTESIAN_POINT('Ctrl Pts',(-40.3374497839604,19.938389785095,22.3486402108316));
#33435=CARTESIAN_POINT('Ctrl Pts',(-35.5481193843904,19.7189203495023,23.1505293518543));
#33436=CARTESIAN_POINT('Ctrl Pts',(-30.7463933706032,19.5342279169114,23.3146671605512));
#33437=CARTESIAN_POINT('Ctrl Pts',(-26.0040969144944,19.3763677050182,22.8629084611189));
#33438=CARTESIAN_POINT('Ctrl Pts',(-21.3476789228923,19.2344308170631,21.9302640427997));
#33439=CARTESIAN_POINT('Ctrl Pts',(-16.8465197078137,19.1049298841923,20.4114158677415));
#33440=CARTESIAN_POINT('Ctrl Pts',(-12.5724038286273,18.9752993129734,18.3291382226407));
#33441=CARTESIAN_POINT('Ctrl Pts',(-9.09731433688908,18.8580619466085,16.1685777235212));
#33442=CARTESIAN_POINT('Ctrl Pts',(-6.92801395023321,18.7718242877839,14.4848376291825));
#33443=CARTESIAN_POINT('Ctrl Pts',(-5.5565905826503,18.7111415689428,13.2995228472163));
#33444=CARTESIAN_POINT('Ctrl Pts',(-5.23274868623665,18.6963263828107,13.0101011772342));
#33445=CARTESIAN_POINT('Ctrl Pts',(-4.91421109534465,18.6812985797984,12.7158283323917));
#33446=CARTESIAN_POINT('Ctrl Pts',(-47.1197799375165,19.4355555088431,22.0960871589275));
#33447=CARTESIAN_POINT('Ctrl Pts',(-46.7264560399874,19.4044605226273,22.2753517007042));
#33448=CARTESIAN_POINT('Ctrl Pts',(-46.3287607622083,19.3735658358572,22.4486582051412));
#33449=CARTESIAN_POINT('Ctrl Pts',(-44.6133426779924,19.2426748194849,23.1621348317923));
#33450=CARTESIAN_POINT('Ctrl Pts',(-41.9578562868468,19.0517849995255,24.0980041256472));
#33451=CARTESIAN_POINT('Ctrl Pts',(-37.9214699510629,18.7933185397158,25.0434190840267));
#33452=CARTESIAN_POINT('Ctrl Pts',(-33.1886838105404,18.5218580841843,25.6252819356792));
#33453=CARTESIAN_POINT('Ctrl Pts',(-28.4743321897673,18.2836948825759,25.5728713432753));
#33454=CARTESIAN_POINT('Ctrl Pts',(-23.8505519067561,18.0697821020849,24.9121197610862));
#33455=CARTESIAN_POINT('Ctrl Pts',(-19.3377142376472,17.8693333343866,23.7786996168262));
#33456=CARTESIAN_POINT('Ctrl Pts',(-15.011646119972,17.6778661310593,22.0720595234769));
#33457=CARTESIAN_POINT('Ctrl Pts',(-10.9443805849522,17.4826662284719,19.8190139836521));
#33458=CARTESIAN_POINT('Ctrl Pts',(-7.66847558815272,17.3068805329357,17.5255820876028));
#33459=CARTESIAN_POINT('Ctrl Pts',(-5.6466240636577,17.1802068447994,15.7634687908796));
#33460=CARTESIAN_POINT('Ctrl Pts',(-4.377043727754,17.0925519552341,14.5303453508661));
#33461=CARTESIAN_POINT('Ctrl Pts',(-4.07789825385118,17.0712544126695,14.2297400151586));
#33462=CARTESIAN_POINT('Ctrl Pts',(-3.78430609072903,17.0497370990139,13.9245789280815));
#33463=CARTESIAN_POINT('Ctrl Pts',(-44.3588433405874,17.8320672383652,25.6251707043937));
#33464=CARTESIAN_POINT('Ctrl Pts',(-43.9647231330525,17.7976045693245,25.7824986209223));
#33465=CARTESIAN_POINT('Ctrl Pts',(-43.5665026079252,17.7633163796081,25.9336811896756));
#33466=CARTESIAN_POINT('Ctrl Pts',(-41.8500316111937,17.6178640028275,26.551947798518));
#33467=CARTESIAN_POINT('Ctrl Pts',(-39.2009778348922,17.4049846203341,27.3407744261555));
#33468=CARTESIAN_POINT('Ctrl Pts',(-35.1985919001064,17.1135517229592,28.0640113741508));
#33469=CARTESIAN_POINT('Ctrl Pts',(-30.5341196997764,16.8027253827761,28.3872728640342));
#33470=CARTESIAN_POINT('Ctrl Pts',(-25.9241726995091,16.523022337621,28.0801390685936));
#33471=CARTESIAN_POINT('Ctrl Pts',(-21.4412740362845,16.2641978724915,27.1732354593264));
#33472=CARTESIAN_POINT('Ctrl Pts',(-17.0986862433379,16.0157341831644,25.8030223951057));
#33473=CARTESIAN_POINT('Ctrl Pts',(-12.9798020686036,15.7719994721116,23.8744122556853));
#33474=CARTESIAN_POINT('Ctrl Pts',(-9.1569628467535,15.5202180684676,21.4188737268354));
#33475=CARTESIAN_POINT('Ctrl Pts',(-6.11623608466224,15.2931736272884,18.9673373050427));
#33476=CARTESIAN_POINT('Ctrl Pts',(-4.26837011845563,15.130708702949,17.11151869867));
#33477=CARTESIAN_POINT('Ctrl Pts',(-3.11893115402554,15.0190926843839,15.8210499974158));
#33478=CARTESIAN_POINT('Ctrl Pts',(-2.84897205769882,14.9920326361705,15.5070667262007));
#33479=CARTESIAN_POINT('Ctrl Pts',(-2.58491016590009,14.9647422323135,15.1889189006689));
#33480=CARTESIAN_POINT('Ctrl Pts',(-41.7296709001059,15.7638142683891,28.9833190904297));
#33481=CARTESIAN_POINT('Ctrl Pts',(-41.3348460424531,15.7283726072843,29.1186893077136));
#33482=CARTESIAN_POINT('Ctrl Pts',(-40.9362136579705,15.6930928161318,29.2477074393503));
#33483=CARTESIAN_POINT('Ctrl Pts',(-39.2192736909589,15.543379415412,29.7705107854804));
#33484=CARTESIAN_POINT('Ctrl Pts',(-36.5775716396078,15.3241289383934,30.4118817928407));
#33485=CARTESIAN_POINT('Ctrl Pts',(-32.6106560319495,15.0227233638938,30.9122052920021));
#33486=CARTESIAN_POINT('Ctrl Pts',(-28.01633587977,14.6988957424381,30.9758283948891));
#33487=CARTESIAN_POINT('Ctrl Pts',(-23.5128043811657,14.4035050799014,30.4126590158976));
#33488=CARTESIAN_POINT('Ctrl Pts',(-19.1729950858667,14.1252237593235,29.2579436351381));
#33489=CARTESIAN_POINT('Ctrl Pts',(-15.0030335205516,13.8539516979883,27.6489638156294));
#33490=CARTESIAN_POINT('Ctrl Pts',(-11.0939336494892,13.5829362127958,25.4959726484748));
#33491=CARTESIAN_POINT('Ctrl Pts',(-7.51836322006334,13.2994842764397,22.8350284903861));
#33492=CARTESIAN_POINT('Ctrl Pts',(-4.71542492625827,13.0425486753816,20.2225182721821));
#33493=CARTESIAN_POINT('Ctrl Pts',(-3.04340561577518,12.8585920936854,18.2708142716326));
#33494=CARTESIAN_POINT('Ctrl Pts',(-2.01537371507192,12.7324540777387,16.9214722846062));
#33495=CARTESIAN_POINT('Ctrl Pts',(-1.77495594634031,12.7018988467546,16.5938079667051));
#33496=CARTESIAN_POINT('Ctrl Pts',(-1.54082751975146,12.6711030837425,16.2624338230772));
#33497=CARTESIAN_POINT('Ctrl Pts',(-39.2586465641561,13.2592937677246,32.138632362006));
#33498=CARTESIAN_POINT('Ctrl Pts',(-38.8630617067816,13.2252177231213,32.2522058668933));
#33499=CARTESIAN_POINT('Ctrl Pts',(-38.4639826224378,13.191306123502,32.3592050870755));
#33500=CARTESIAN_POINT('Ctrl Pts',(-36.7465199894602,13.0474600457288,32.7871034898597));
#33501=CARTESIAN_POINT('Ctrl Pts',(-34.1121212490597,12.8372075593629,33.281827219888));
#33502=CARTESIAN_POINT('Ctrl Pts',(-30.1807185681909,12.5484949329477,33.5602745004599));
#33503=CARTESIAN_POINT('Ctrl Pts',(-25.6567480538887,12.2377054846042,33.3652273449456));
#33504=CARTESIAN_POINT('Ctrl Pts',(-21.2600291633834,11.9522310106351,32.5466444033322));
#33505=CARTESIAN_POINT('Ctrl Pts',(-17.063923538417,11.6797819251771,31.1443337349231));
#33506=CARTESIAN_POINT('Ctrl Pts',(-13.0673837668308,11.4108111467242,29.2964501962854));
#33507=CARTESIAN_POINT('Ctrl Pts',(-9.36909897898788,11.1374939458242,26.9184639603245));
#33508=CARTESIAN_POINT('Ctrl Pts',(-6.04207397664205,10.8473681096278,24.0509736936325));
#33509=CARTESIAN_POINT('Ctrl Pts',(-3.4781910952484,10.5820480444149,21.2761299820227));
#33510=CARTESIAN_POINT('Ctrl Pts',(-1.98298065004395,10.3910369789073,19.2273659536365));
#33511=CARTESIAN_POINT('Ctrl Pts',(-1.0770281441367,10.2599216927486,17.818285691764));
#33512=CARTESIAN_POINT('Ctrl Pts',(-0.866345765711677,10.2281653805015,
17.4768046358873));
#33513=CARTESIAN_POINT('Ctrl Pts',(-0.662374778275869,10.1961599190035,
17.1321395719343));
#33514=CARTESIAN_POINT('Ctrl Pts',(-36.9283535544487,10.420684636249,35.1144434311013));
#33515=CARTESIAN_POINT('Ctrl Pts',(-36.5318752578966,10.3898269637342,35.2064485096914));
#33516=CARTESIAN_POINT('Ctrl Pts',(-36.1322371476585,10.3591499865554,35.2916452167048));
#33517=CARTESIAN_POINT('Ctrl Pts',(-34.4138694749954,10.2291883131935,35.6255156634962));
#33518=CARTESIAN_POINT('Ctrl Pts',(-31.7862198804387,10.0401067219452,35.9748869984656));
#33519=CARTESIAN_POINT('Ctrl Pts',(-27.8896025965576,9.78206378055234,36.0332305838768));
#33520=CARTESIAN_POINT('Ctrl Pts',(-23.4352630122845,9.50499638561923,35.5813563586842));
#33521=CARTESIAN_POINT('Ctrl Pts',(-19.1448101772899,9.24981780003299,34.5088914700998));
#33522=CARTESIAN_POINT('Ctrl Pts',(-15.0920445718706,9.00337535985762,32.8601648563575));
#33523=CARTESIAN_POINT('Ctrl Pts',(-11.2687133422595,8.75677479408939,30.774255852101));
#33524=CARTESIAN_POINT('Ctrl Pts',(-7.78122280819138,8.50116890088297,28.1717533340615));
#33525=CARTESIAN_POINT('Ctrl Pts',(-4.70291928851549,8.22444592813344,25.0977652109468));
#33526=CARTESIAN_POINT('Ctrl Pts',(-2.37837898968668,7.96804930448713,22.1603214494423));
#33527=CARTESIAN_POINT('Ctrl Pts',(-1.06026023796119,7.78162503245108,20.0141066859967));
#33528=CARTESIAN_POINT('Ctrl Pts',(-0.276603268679021,7.65323614745839,
18.5449588939088));
#33529=CARTESIAN_POINT('Ctrl Pts',(-0.0957191124462417,7.62212996336316,
18.1896586961835));
#33530=CARTESIAN_POINT('Ctrl Pts',(0.0780231590676284,7.59076668565169,
17.8317752735585));
#33531=CARTESIAN_POINT('Ctrl Pts',(-34.7917671754843,7.18298363715391,37.8442219967885));
#33532=CARTESIAN_POINT('Ctrl Pts',(-34.3941476924951,7.15763661423686,37.9150556358309));
#33533=CARTESIAN_POINT('Ctrl Pts',(-33.9937202099012,7.13250342173354,37.97883916718));
#33534=CARTESIAN_POINT('Ctrl Pts',(-32.2735452011381,7.02634360727853,38.2203153715421));
#33535=CARTESIAN_POINT('Ctrl Pts',(-29.6513074607424,6.87350147707393,38.4267628259902));
#33536=CARTESIAN_POINT('Ctrl Pts',(-25.7876131165973,6.66841421880391,38.2683972300439));
#33537=CARTESIAN_POINT('Ctrl Pts',(-21.4009082217558,6.45075222930465,37.5633374197196));
#33538=CARTESIAN_POINT('Ctrl Pts',(-17.2149552435157,6.25122984378583,36.2402006917209));
#33539=CARTESIAN_POINT('Ctrl Pts',(-13.3040026940452,6.05595707526583,34.3477946257551));
#33540=CARTESIAN_POINT('Ctrl Pts',(-9.6525471111465,5.8568061689083,32.0261986676909));
#33541=CARTESIAN_POINT('Ctrl Pts',(-6.37476293151624,5.64398234710963,29.2009985033296));
#33542=CARTESIAN_POINT('Ctrl Pts',(-3.54433846437633,5.40587468584602,25.9217831684824));
#33543=CARTESIAN_POINT('Ctrl Pts',(-1.45858600572521,5.18017895256177,22.822442252468));
#33544=CARTESIAN_POINT('Ctrl Pts',(-0.31729954633703,5.01301666232781,20.5789820379423));
#33545=CARTESIAN_POINT('Ctrl Pts',(0.344196822049049,4.89707445701614,19.0498138141221));
#33546=CARTESIAN_POINT('Ctrl Pts',(0.495324122044482,4.86894780999335,18.6807807474581));
#33547=CARTESIAN_POINT('Ctrl Pts',(0.638889978344851,4.84055053954568,18.3098379674021));
#33548=CARTESIAN_POINT('Ctrl Pts',(-32.8758727169027,3.57357815210241,40.2949547456763));
#33549=CARTESIAN_POINT('Ctrl Pts',(-32.4767273615688,3.55599962931061,40.3451948528862));
#33550=CARTESIAN_POINT('Ctrl Pts',(-32.0751371433406,3.53868515668548,40.3881395758659));
#33551=CARTESIAN_POINT('Ctrl Pts',(-30.3516146892127,3.46609807861293,40.5396626066785));
#33552=CARTESIAN_POINT('Ctrl Pts',(-27.7324819356722,3.36435917107101,40.6068323220244));
#33553=CARTESIAN_POINT('Ctrl Pts',(-23.8984124909247,3.23426720235262,40.2369275639187));
#33554=CARTESIAN_POINT('Ctrl Pts',(-19.5756899976202,3.10147907156715,39.2843419828594));
#33555=CARTESIAN_POINT('Ctrl Pts',(-15.4908341395163,2.98285053627008,37.7157037013977));
#33556=CARTESIAN_POINT('Ctrl Pts',(-11.718544299807,2.86388130857434,35.5842699988208));
#33557=CARTESIAN_POINT('Ctrl Pts',(-8.23601495093128,2.73730530568202,33.0312127971187));
#33558=CARTESIAN_POINT('Ctrl Pts',(-5.16523654947227,2.59247375589619,29.9869957655452));
#33559=CARTESIAN_POINT('Ctrl Pts',(-2.58023204587429,2.41842603756845,26.5056777619934));
#33560=CARTESIAN_POINT('Ctrl Pts',(-0.731320310752,2.24547053120763,23.2467344970765));
#33561=CARTESIAN_POINT('Ctrl Pts',(0.234328739827367,2.11246131963295,20.9073033347448));
#33562=CARTESIAN_POINT('Ctrl Pts',(0.774418224855581,2.01884144332686,19.3188699442435));
#33563=CARTESIAN_POINT('Ctrl Pts',(0.895998757480463,1.99605339732081,18.9363491825155));
#33564=CARTESIAN_POINT('Ctrl Pts',(1.0096286841352,1.9729679754383,18.5526533795054));
#33565=CARTESIAN_POINT('Ctrl Pts',(-31.3974772080596,0.237308438758995,
42.1889013144209));
#33566=CARTESIAN_POINT('Ctrl Pts',(-30.9966927888425,0.227921876287717,
42.2219698988398));
#33567=CARTESIAN_POINT('Ctrl Pts',(-30.5937820398667,0.218854274805993,
42.2475319255546));
#33568=CARTESIAN_POINT('Ctrl Pts',(-28.866041531999,0.181679983795775,42.3239971106882));
#33569=CARTESIAN_POINT('Ctrl Pts',(-26.2475430587419,0.133848323063104,
42.274846063482));
#33570=CARTESIAN_POINT('Ctrl Pts',(-22.4359447693504,0.0830496793456984,
41.7279849455362));
#33571=CARTESIAN_POINT('Ctrl Pts',(-18.1647975152526,0.0403924264632703,
40.5680465840115));
#33572=CARTESIAN_POINT('Ctrl Pts',(-14.1635084800691,0.00837005963384143,
38.7934300768119));
#33573=CARTESIAN_POINT('Ctrl Pts',(-10.5071625432585,-0.0279539839125438,
36.4611931292656));
#33574=CARTESIAN_POINT('Ctrl Pts',(-7.16665730012202,-0.0750512999789021,
33.7135147932952));
#33575=CARTESIAN_POINT('Ctrl Pts',(-4.27071386437358,-0.14423024726241,
30.4849603838039));
#33576=CARTESIAN_POINT('Ctrl Pts',(-1.89363332772792,-0.245792879606331,
26.8334203010956));
#33577=CARTESIAN_POINT('Ctrl Pts',(-0.245746173750661,-0.358291148292244,
23.4399943636853));
#33578=CARTESIAN_POINT('Ctrl Pts',(0.570610862782009,-0.451704594358635,
21.0196785831955));
#33579=CARTESIAN_POINT('Ctrl Pts',(1.00744205759503,-0.519340602547392,
19.3812974878904));
#33580=CARTESIAN_POINT('Ctrl Pts',(1.10392460430938,-0.535923052101836,
18.9874616998164));
#33581=CARTESIAN_POINT('Ctrl Pts',(1.19215808188825,-0.552841667182328,
18.5931197045587));
#33582=CARTESIAN_POINT('Ctrl Pts',(-30.5294236725591,-2.14030259993981,
43.3034186854275));
#33583=CARTESIAN_POINT('Ctrl Pts',(-30.1272931149697,-2.14321532053782,
43.3254158563938));
#33584=CARTESIAN_POINT('Ctrl Pts',(-29.72324694576,-2.14576465810466,43.3397662219238));
#33585=CARTESIAN_POINT('Ctrl Pts',(-27.9915993478864,-2.15494826818845,
43.3678047673857));
#33586=CARTESIAN_POINT('Ctrl Pts',(-25.3718743099029,-2.16016260296573,
43.2435221176539));
#33587=CARTESIAN_POINT('Ctrl Pts',(-21.572867015554,-2.1481556077715,42.5821474979001));
#33588=CARTESIAN_POINT('Ctrl Pts',(-17.333414526286,-2.11918777525101,41.2878074756749));
#33589=CARTESIAN_POINT('Ctrl Pts',(-13.3852721551486,-2.08197924289826,
39.379449384515));
#33590=CARTESIAN_POINT('Ctrl Pts',(-9.80377918929066,-2.05170003121316,
36.9166597127083));
#33591=CARTESIAN_POINT('Ctrl Pts',(-6.55560827573149,-2.03426137368081,
34.0423409270553));
#33592=CARTESIAN_POINT('Ctrl Pts',(-3.77398725841762,-2.04135770257883,
30.6937413306207));
#33593=CARTESIAN_POINT('Ctrl Pts',(-1.53339439133958,-2.08278583441843,
26.9313113438869));
#33594=CARTESIAN_POINT('Ctrl Pts',(-0.0177672591392232,-2.14471303148954,
23.4502813702109));
#33595=CARTESIAN_POINT('Ctrl Pts',(0.700190966747434,-2.20477046252904,
20.9773004459268));
#33596=CARTESIAN_POINT('Ctrl Pts',(1.06891378933942,-2.25046208753918,19.3064141960021));
#33597=CARTESIAN_POINT('Ctrl Pts',(1.14886051042696,-2.26180965939547,18.9052387021536));
#33598=CARTESIAN_POINT('Ctrl Pts',(1.22037994045603,-2.27353152926925,18.5040148697326));
#33599=CARTESIAN_POINT('Ctrl Pts',(-29.9728399373354,-3.83428286431684,
44.0191242698361));
#33600=CARTESIAN_POINT('Ctrl Pts',(-29.5696745140238,-3.83237339034492,
44.0336174040068));
#33601=CARTESIAN_POINT('Ctrl Pts',(-29.1647389499247,-3.83006698099443,
44.0403669998921));
#33602=CARTESIAN_POINT('Ctrl Pts',(-27.4299435681702,-3.81839846831683,
44.0355693932585));
#33603=CARTESIAN_POINT('Ctrl Pts',(-24.808696764347,-3.79185933798401,43.860310033771));
#33604=CARTESIAN_POINT('Ctrl Pts',(-21.0174144082698,-3.73301479320489,
43.1211526099474));
#33605=CARTESIAN_POINT('Ctrl Pts',(-16.7987669069511,-3.65055513724086,
41.7354370320634));
#33606=CARTESIAN_POINT('Ctrl Pts',(-12.8863048378013,-3.56151400652134,
39.7360659076511));
#33607=CARTESIAN_POINT('Ctrl Pts',(-9.35554180296775,-3.48120332570528,
37.1843738425572));
#33608=CARTESIAN_POINT('Ctrl Pts',(-6.17021960178868,-3.41513875248544,
34.2237830512071));
#33609=CARTESIAN_POINT('Ctrl Pts',(-3.46668816079854,-3.37526128513496,
30.7933795971532));
#33610=CARTESIAN_POINT('Ctrl Pts',(-1.31954448869267,-3.37099617994084,
26.9553877055552));
#33611=CARTESIAN_POINT('Ctrl Pts',(0.105403626449547,-3.39437469848804,
23.4146796719729));
#33612=CARTESIAN_POINT('Ctrl Pts',(0.7558264201022,-3.42893690611626,20.9058438397504));
#33613=CARTESIAN_POINT('Ctrl Pts',(1.07778274982802,-3.45783930783476,19.2128393202058));
#33614=CARTESIAN_POINT('Ctrl Pts',(1.14638473165933,-3.46518513130081,18.806679408153));
#33615=CARTESIAN_POINT('Ctrl Pts',(1.20644655773061,-3.47293757911652,18.4007919683856));
#33616=CARTESIAN_POINT('Ctrl Pts',(-29.8240879871509,-4.30636894546118,
44.2105267227162));
#33617=CARTESIAN_POINT('Ctrl Pts',(-29.4206225151076,-4.3031084050989,44.2229739248513));
#33618=CARTESIAN_POINT('Ctrl Pts',(-29.0154266865265,-4.29944065268701,
44.2276505601386));
#33619=CARTESIAN_POINT('Ctrl Pts',(-27.2796978130663,-4.28192251284736,
44.2138948132052));
#33620=CARTESIAN_POINT('Ctrl Pts',(-24.6579368258278,-4.24645759656194,
44.0247144994774));
#33621=CARTESIAN_POINT('Ctrl Pts',(-20.8686620252869,-4.17439213330946,
43.2642815747257));
#33622=CARTESIAN_POINT('Ctrl Pts',(-16.6556313915342,-4.07676875425951,
41.8535410709043));
#33623=CARTESIAN_POINT('Ctrl Pts',(-12.752916079089,-3.97294922980807,39.8292172170953));
#33624=CARTESIAN_POINT('Ctrl Pts',(-9.23607101592842,-3.87828739688684,
37.2531390788911));
#33625=CARTESIAN_POINT('Ctrl Pts',(-6.06801599636428,-3.79820251809058,
34.2688877835182));
#33626=CARTESIAN_POINT('Ctrl Pts',(-3.38594976443961,-3.74469501429227,
30.8160631689765));
#33627=CARTESIAN_POINT('Ctrl Pts',(-1.26447813113574,-3.72710099262819,
26.9573886132689));
#33628=CARTESIAN_POINT('Ctrl Pts',(0.135589853537579,-3.7392015362719,23.4003753828037));
#33629=CARTESIAN_POINT('Ctrl Pts',(0.767503701216293,-3.76629674044718,
20.8817611257437));
#33630=CARTESIAN_POINT('Ctrl Pts',(1.07665298555957,-3.79028538091932,19.182731725672));
#33631=CARTESIAN_POINT('Ctrl Pts',(1.14215062469445,-3.79646095010219,18.7752153335603));
#33632=CARTESIAN_POINT('Ctrl Pts',(1.19907952975018,-3.80305340259771,18.3680599208473));
#33633=CARTESIAN_POINT('Ctrl Pts',(-29.6806279783958,-4.78145508078572,
44.3952414011369));
#33634=CARTESIAN_POINT('Ctrl Pts',(-29.2768504019181,-4.77682808742727,
44.4056744850212));
#33635=CARTESIAN_POINT('Ctrl Pts',(-28.8713813649358,-4.7717826224726,44.4083097320835));
#33636=CARTESIAN_POINT('Ctrl Pts',(-27.1346599350118,-4.74834091216943,
44.3857294295924));
#33637=CARTESIAN_POINT('Ctrl Pts',(-24.5122959636537,-4.70381966688121,
44.1828218130499));
#33638=CARTESIAN_POINT('Ctrl Pts',(-20.7249024233729,-4.61828583278682,
43.4013748323987));
#33639=CARTESIAN_POINT('Ctrl Pts',(-16.5173497068994,-4.50515190400754,
41.9658851598471));
#33640=CARTESIAN_POINT('Ctrl Pts',(-12.6242519830332,-4.38613315046716,
39.9168561359679));
#33641=CARTESIAN_POINT('Ctrl Pts',(-9.12119860544565,-4.27662792828432,
37.3166215213372));
#33642=CARTESIAN_POINT('Ctrl Pts',(-5.97027712488791,-4.18197237106197,
34.3089362976155));
#33643=CARTESIAN_POINT('Ctrl Pts',(-3.30951923630238,-4.11421750462538,
30.833918806753));
#33644=CARTESIAN_POINT('Ctrl Pts',(-1.21351550607071,-4.08262421860679,
26.9547993627852));
#33645=CARTESIAN_POINT('Ctrl Pts',(0.161901966116654,-4.0828488851085,23.381697762374));
#33646=CARTESIAN_POINT('Ctrl Pts',(0.775499329277603,-4.10207414795096,
20.8534525370212));
#33647=CARTESIAN_POINT('Ctrl Pts',(1.07198479735696,-4.12088738197538,19.1484961887738));
#33648=CARTESIAN_POINT('Ctrl Pts',(1.13441433400836,-4.12583098108427,18.7396458756966));
#33649=CARTESIAN_POINT('Ctrl Pts',(1.18824830736423,-4.13120272145022,18.3312440582198));
#33650=CARTESIAN_POINT('',(-42.5975526516,20.7105311502984,19.56306858979));
#33651=CARTESIAN_POINT('Ctrl Pts',(-42.5975526516,20.7105311502984,19.56306858979));
#33652=CARTESIAN_POINT('Ctrl Pts',(-37.5762221249469,20.5483438544848,20.8499577962863));
#33653=CARTESIAN_POINT('Ctrl Pts',(-32.3097534431554,20.4520245495079,21.1410367283647));
#33654=CARTESIAN_POINT('Ctrl Pts',(-22.0288042740374,20.3052748660675,19.8252715829174));
#33655=CARTESIAN_POINT('Ctrl Pts',(-17.0125234745079,20.248474007324,18.2209789914172));
#33656=CARTESIAN_POINT('Ctrl Pts',(-12.4794056444224,20.1925493450898,15.715137789166));
#33657=CARTESIAN_POINT('',(-19.776612741422,-3.27137091447503,42.4988384174391));
#33658=CARTESIAN_POINT('Ctrl Pts',(-42.5975526515946,20.7105311502992,19.5630685897878));
#33659=CARTESIAN_POINT('Ctrl Pts',(-41.2774004556305,19.9641940681955,22.4376316497411));
#33660=CARTESIAN_POINT('Ctrl Pts',(-39.7028421419984,18.733618922395,25.0874965293065));
#33661=CARTESIAN_POINT('Ctrl Pts',(-36.0874408763569,15.6437709263415,30.09428841202));
#33662=CARTESIAN_POINT('Ctrl Pts',(-33.9437320263055,13.6706054953475,32.4640497220532));
#33663=CARTESIAN_POINT('Ctrl Pts',(-29.6530167610139,9.45712578015136,36.416476789843));
#33664=CARTESIAN_POINT('Ctrl Pts',(-27.4644787406163,7.18268855808106,38.0675475180451));
#33665=CARTESIAN_POINT('Ctrl Pts',(-23.3434412931498,2.26699026933705,40.7209158524528));
#33666=CARTESIAN_POINT('Ctrl Pts',(-21.4078194194595,-0.365223992194613,
41.73976451752));
#33667=CARTESIAN_POINT('Ctrl Pts',(-19.7766121648793,-3.27137053313467,
42.4988386384589));
#33668=CARTESIAN_POINT('Ctrl Pts',(-19.7766128803973,-3.27137100135121,
42.4988379590673));
#33669=CARTESIAN_POINT('Ctrl Pts',(-19.0339274479275,-3.25992112204952,
42.2714904731699));
#33670=CARTESIAN_POINT('Ctrl Pts',(-18.3028671461025,-3.24789096533568,
42.0167733291065));
#33671=CARTESIAN_POINT('Ctrl Pts',(-17.5847573966283,-3.23555894384663,
41.7357426201857));
#33672=CARTESIAN_POINT('Ctrl Pts',(-15.82608090219,-3.2053573815679,41.047488349364));
#33673=CARTESIAN_POINT('Ctrl Pts',(-14.1450790808029,-3.17334534347451,
40.201411150032));
#33674=CARTESIAN_POINT('Ctrl Pts',(-12.561157306208,-3.14345008158506,39.2131583578373));
#33675=CARTESIAN_POINT('Ctrl Pts',(-11.5052094029128,-3.12351990598109,
38.5543231296199));
#33676=CARTESIAN_POINT('Ctrl Pts',(-10.4924081914375,-3.10453051989494,
37.8322987426006));
#33677=CARTESIAN_POINT('Ctrl Pts',(-9.52847648856522,-3.08752071373526,
37.0517562442537));
#33678=CARTESIAN_POINT('Ctrl Pts',(-8.56454478619749,-3.07051090758448,
36.2712137463155));
#33679=CARTESIAN_POINT('Ctrl Pts',(-7.64948259237388,-3.0554806813514,35.4321531371102));
#33680=CARTESIAN_POINT('Ctrl Pts',(-6.78900009497131,-3.04339100491455,
34.5392583133731));
#33681=CARTESIAN_POINT('Ctrl Pts',(-5.49827635047142,-3.02525649028182,
33.1999160794317));
#33682=CARTESIAN_POINT('Ctrl Pts',(-4.33035692256822,-3.01373821257335,
31.7394468631442));
#33683=CARTESIAN_POINT('Ctrl Pts',(-3.30441544543477,-3.01128625574909,
30.1737249320072));
#33684=CARTESIAN_POINT('Ctrl Pts',(-2.62045446228512,-3.00965161787009,
29.1299103137002));
#33685=CARTESIAN_POINT('Ctrl Pts',(-1.99959479025531,-3.01204645592803,
28.0393167111781));
#33686=CARTESIAN_POINT('Ctrl Pts',(-1.44749052671152,-3.01891855380822,
26.9066548859025));
#33687=CARTESIAN_POINT('Ctrl Pts',(-0.895386329367994,-3.02579065086441,
25.7739931964392));
#33688=CARTESIAN_POINT('Ctrl Pts',(-0.412037523989561,-3.03714000665748,
24.5992632942881));
#33689=CARTESIAN_POINT('Ctrl Pts',(-0.00308425577624904,-3.05321938564873,
23.3871704735693));
#33690=CARTESIAN_POINT('Ctrl Pts',(0.165431602385786,-3.05984515577954,
22.8877078754395));
#33691=CARTESIAN_POINT('Ctrl Pts',(0.321315192441404,-3.06727406915266,
22.381901115368));
#33692=CARTESIAN_POINT('Ctrl Pts',(0.464173291851462,-3.07550335254719,
21.8700789527947));
#33693=CARTESIAN_POINT('Ctrl Pts',(-29.5860843849178,-4.68328060676847,
44.5216251990609));
#33694=CARTESIAN_POINT('Ctrl Pts',(-29.1809745858381,-4.67927906663786,
44.5315997635342));
#33695=CARTESIAN_POINT('Ctrl Pts',(-28.7741766395213,-4.67486342687383,
44.5337119281872));
#33696=CARTESIAN_POINT('Ctrl Pts',(-27.0369350215887,-4.65418501649615,
44.5086929582487));
#33697=CARTESIAN_POINT('Ctrl Pts',(-24.416253162149,-4.61395560865182,44.3020849732412));
#33698=CARTESIAN_POINT('Ctrl Pts',(-20.6316091853443,-4.53496565777432,
43.5151118207757));
#33699=CARTESIAN_POINT('Ctrl Pts',(-16.4275307990086,-4.42959393838223,
42.0732275761618));
#33700=CARTESIAN_POINT('Ctrl Pts',(-12.5382448797194,-4.31850354734918,
40.0179024219213));
#33701=CARTESIAN_POINT('Ctrl Pts',(-9.03935092612681,-4.2170896233612,37.4115163382363));
#33702=CARTESIAN_POINT('Ctrl Pts',(-5.89288171525852,-4.13063759391767,
34.3978116754749));
#33703=CARTESIAN_POINT('Ctrl Pts',(-3.23694972107052,-4.07121155600733,
30.9169763478869));
#33704=CARTESIAN_POINT('Ctrl Pts',(-1.14615791734321,-4.04803120464602,
27.0322881721863));
#33705=CARTESIAN_POINT('Ctrl Pts',(0.224522517554149,-4.055480889925,23.4546075941498));
#33706=CARTESIAN_POINT('Ctrl Pts',(0.834789683250672,-4.07952578289679,
20.9234587390748));
#33707=CARTESIAN_POINT('Ctrl Pts',(1.12940732404397,-4.10152925776619,19.214455857901));
#33708=CARTESIAN_POINT('Ctrl Pts',(1.19158024061946,-4.1072571624472,18.8029939189201));
#33709=CARTESIAN_POINT('Ctrl Pts',(1.2450644513097,-4.11341014061892,18.3920080529356));
#33710=CARTESIAN_POINT('Ctrl Pts',(-29.7642796229678,-4.24009445412503,
44.2925926955476));
#33711=CARTESIAN_POINT('Ctrl Pts',(-29.359411518692,-4.23725223817857,44.3047887517873));
#33712=CARTESIAN_POINT('Ctrl Pts',(-28.9528099886829,-4.23400446880359,
44.3091515696117));
#33713=CARTESIAN_POINT('Ctrl Pts',(-27.2162036125542,-4.21832863439708,
44.2938289943612));
#33714=CARTESIAN_POINT('Ctrl Pts',(-24.5955479639773,-4.18572164472913,
44.1022702841641));
#33715=CARTESIAN_POINT('Ctrl Pts',(-20.8080715768724,-4.11799618192084,
43.3382863119255));
#33716=CARTESIAN_POINT('Ctrl Pts',(-16.5973033266347,-4.02550335874969,
41.9234398290087));
#33717=CARTESIAN_POINT('Ctrl Pts',(-12.697056845913,-3.92690475481451,39.8950785227414));
#33718=CARTESIAN_POINT('Ctrl Pts',(-9.18289043977616,-3.83755718932749,
37.3150628289422));
#33719=CARTESIAN_POINT('Ctrl Pts',(-6.01768716647963,-3.76285616468038,
34.3269670070901));
#33720=CARTESIAN_POINT('Ctrl Pts',(-3.33869209457895,-3.71481495977278,
30.8704356073741));
#33721=CARTESIAN_POINT('Ctrl Pts',(-1.2205165590504,-3.70275434803773,27.0082200856332));
#33722=CARTESIAN_POINT('Ctrl Pts',(0.176569306956024,-3.71962751323487,
23.4482980813067));
#33723=CARTESIAN_POINT('Ctrl Pts',(0.806392352236958,-3.74992063397164,
20.9278383983267));
#33724=CARTESIAN_POINT('Ctrl Pts',(1.11452777256288,-3.77604797989279,19.2254460436222));
#33725=CARTESIAN_POINT('Ctrl Pts',(1.17998786511121,-3.78276245762616,18.815479564919));
#33726=CARTESIAN_POINT('Ctrl Pts',(1.23678687530853,-3.78989370687861,18.4058928046142));
#33727=CARTESIAN_POINT('Ctrl Pts',(-29.9461184866339,-3.80075287541765,
44.0589752842181));
#33728=CARTESIAN_POINT('Ctrl Pts',(-29.5414810641717,-3.79905339336963,
44.0734114048756));
#33729=CARTESIAN_POINT('Ctrl Pts',(-29.1350644418468,-3.79695621683146,
44.0800431213998));
#33730=CARTESIAN_POINT('Ctrl Pts',(-27.3990422401927,-3.78620663871065,
44.0744931264123));
#33731=CARTESIAN_POINT('Ctrl Pts',(-24.7783398189311,-3.76109400159902,
43.8980891928852));
#33732=CARTESIAN_POINT('Ctrl Pts',(-20.9879390718351,-3.70440674399875,
43.1572232592788));
#33733=CARTESIAN_POINT('Ctrl Pts',(-16.7703956156188,-3.62448835210827,
41.7695337527048));
#33734=CARTESIAN_POINT('Ctrl Pts',(-12.8591316466056,-3.53802316526296,
39.7682243997015));
#33735=CARTESIAN_POINT('Ctrl Pts',(-9.32966070272471,-3.46032715355504,
37.2146458262608));
#33736=CARTESIAN_POINT('Ctrl Pts',(-6.14570601219839,-3.39690914788247,
34.2522176672827));
#33737=CARTESIAN_POINT('Ctrl Pts',(-3.44363678759394,-3.35971861494906,
30.820047545745));
#33738=CARTESIAN_POINT('Ctrl Pts',(-1.29805125064107,-3.35817927654809,
26.9803719825628));
#33739=CARTESIAN_POINT('Ctrl Pts',(0.125494730687221,-3.38391914529348,
23.4382826058056));
#33740=CARTESIAN_POINT('Ctrl Pts',(0.774937722763661,-3.42007079724739,
20.9285700499322));
#33741=CARTESIAN_POINT('Ctrl Pts',(1.09664683736935,-3.45006162272336,19.2328302145806));
#33742=CARTESIAN_POINT('Ctrl Pts',(1.16540949069431,-3.45770043113048,18.8243690332114));
#33743=CARTESIAN_POINT('Ctrl Pts',(1.22554046200446,-3.46574819271174,18.4161908869355));
#33744=CARTESIAN_POINT('Ctrl Pts',(-30.6001603149859,-2.2653457359543,43.2190559709685));
#33745=CARTESIAN_POINT('Ctrl Pts',(-30.1962920925288,-2.26761569662348,
43.2414546676051));
#33746=CARTESIAN_POINT('Ctrl Pts',(-29.790483177066,-2.26951335386862,43.2561496325629));
#33747=CARTESIAN_POINT('Ctrl Pts',(-28.056332027324,-2.27586002752392,43.2853222550732));
#33748=CARTESIAN_POINT('Ctrl Pts',(-25.4351951428781,-2.27671432942662,
43.1627196453144));
#33749=CARTESIAN_POINT('Ctrl Pts',(-21.6341437305441,-2.25814179129592,
42.5038126448418));
#33750=CARTESIAN_POINT('Ctrl Pts',(-17.3923960901783,-2.2214798205824,41.2122877014012));
#33751=CARTESIAN_POINT('Ctrl Pts',(-13.4420746485557,-2.17652897108851,
39.3066630970881));
#33752=CARTESIAN_POINT('Ctrl Pts',(-9.85852300070146,-2.13845241575724,
36.8465264101127));
#33753=CARTESIAN_POINT('Ctrl Pts',(-6.60839102281067,-2.11316923258448,
33.9747989860199));
#33754=CARTESIAN_POINT('Ctrl Pts',(-3.82493207095045,-2.11235831802136,
30.6287183522426));
#33755=CARTESIAN_POINT('Ctrl Pts',(-1.58262415787283,-2.14581153060268,
26.8687460420206));
#33756=CARTESIAN_POINT('Ctrl Pts',(-0.0656103164190895,-2.20085463389179,
23.3897875019218));
#33757=CARTESIAN_POINT('Ctrl Pts',(0.653217774137632,-2.25628908058851,
20.9181693846315));
#33758=CARTESIAN_POINT('Ctrl Pts',(1.02296935998166,-2.29898278275007,19.2460320909997));
#33759=CARTESIAN_POINT('Ctrl Pts',(1.10343093441437,-2.30966173471912,18.842915305665));
#33760=CARTESIAN_POINT('Ctrl Pts',(1.17537432901808,-2.32072459453129,18.4397418535062));
#33761=CARTESIAN_POINT('Ctrl Pts',(-31.8292095903569,0.42091842584111,41.6423330468386));
#33762=CARTESIAN_POINT('Ctrl Pts',(-31.426588380617,0.412015546281074,41.6791686699069));
#33763=CARTESIAN_POINT('Ctrl Pts',(-31.0217428525285,0.403442573942463,
41.7084816508355));
#33764=CARTESIAN_POINT('Ctrl Pts',(-29.2904348792228,0.368526239150617,
41.8006000821719));
#33765=CARTESIAN_POINT('Ctrl Pts',(-26.6677579163665,0.324281374370589,
41.7754850488311));
#33766=CARTESIAN_POINT('Ctrl Pts',(-22.8465337117467,0.279215865745994,
41.2649689473965));
#33767=CARTESIAN_POINT('Ctrl Pts',(-18.5602087327645,0.243759038204317,
40.147435296854));
#33768=CARTESIAN_POINT('Ctrl Pts',(-14.5387725951337,0.21967725703067,38.4148047775327));
#33769=CARTESIAN_POINT('Ctrl Pts',(-10.8572617892506,0.192114722189047,
36.1235067085039));
#33770=CARTESIAN_POINT('Ctrl Pts',(-7.48755331988048,0.154437491851918,
33.4155983170629));
#33771=CARTESIAN_POINT('Ctrl Pts',(-4.55732909655327,0.0954817696064694,
30.2249414587457));
#33772=CARTESIAN_POINT('Ctrl Pts',(-2.14084655383702,0.0048363712043943,
26.6088223096227));
#33773=CARTESIAN_POINT('Ctrl Pts',(-0.455654318055976,-0.0979118428630517,
23.2437893603337));
#33774=CARTESIAN_POINT('Ctrl Pts',(0.387941255052986,-0.184631554593919,
20.8409136479811));
#33775=CARTESIAN_POINT('Ctrl Pts',(0.844059787599826,-0.247909792323189,
19.2113700902569));
#33776=CARTESIAN_POINT('Ctrl Pts',(0.945576151375779,-0.263520166061751,
18.8179166382569));
#33777=CARTESIAN_POINT('Ctrl Pts',(1.03880163967271,-0.279478515480188,
18.423810774743));
#33778=CARTESIAN_POINT('Ctrl Pts',(-33.7395940988688,3.93922736422659,39.1963288075476));
#33779=CARTESIAN_POINT('Ctrl Pts',(-33.338359123107,3.92273017306588,39.2538975757074));
#33780=CARTESIAN_POINT('Ctrl Pts',(-32.9345110720053,3.90651491483579,39.3041976635156));
#33781=CARTESIAN_POINT('Ctrl Pts',(-31.2057260147983,3.83888692720806,39.4866672841393));
#33782=CARTESIAN_POINT('Ctrl Pts',(-28.5787152339974,3.74496038387833,39.6013457126449));
#33783=CARTESIAN_POINT('Ctrl Pts',(-24.7261416632,3.6271896762232,39.3032423032837));
#33784=CARTESIAN_POINT('Ctrl Pts',(-20.3739691877485,3.50969140214063,38.4343783563741));
#33785=CARTESIAN_POINT('Ctrl Pts',(-16.2497646181535,3.40771510315772,36.9485603352936));
#33786=CARTESIAN_POINT('Ctrl Pts',(-12.4281284545972,3.30695483103527,34.8977873111395));
#33787=CARTESIAN_POINT('Ctrl Pts',(-8.88820541265663,3.1998573133211,32.4229990482932));
#33788=CARTESIAN_POINT('Ctrl Pts',(-5.74991377138373,3.07607789704229,29.4532363326592));
#33789=CARTESIAN_POINT('Ctrl Pts',(-3.08718802358192,2.92448144596071,26.0413441207066));
#33790=CARTESIAN_POINT('Ctrl Pts',(-1.16461755079814,2.77158317941627,22.8379182506629));
#33791=CARTESIAN_POINT('Ctrl Pts',(-0.145141170452875,2.65236568914073,
20.5324826814612));
#33792=CARTESIAN_POINT('Ctrl Pts',(0.432661725556691,2.56779645721963,18.9632953151811));
#33793=CARTESIAN_POINT('Ctrl Pts',(0.563887154443276,2.54707902977605,18.5835837371794));
#33794=CARTESIAN_POINT('Ctrl Pts',(0.687186542465773,2.52604544176493,18.2024213506929));
#33795=CARTESIAN_POINT('Ctrl Pts',(-36.1213273778177,7.64857049485316,36.1506600847068));
#33796=CARTESIAN_POINT('Ctrl Pts',(-35.7213655257733,7.62538079009264,36.2323665893927));
#33797=CARTESIAN_POINT('Ctrl Pts',(-35.318370358813,7.6024320797305,36.3070907747722));
#33798=CARTESIAN_POINT('Ctrl Pts',(-33.5913541783468,7.50598047950645,36.594676968361));
#33799=CARTESIAN_POINT('Ctrl Pts',(-30.9577397928421,7.36825978906471,36.8718667276266));
#33800=CARTESIAN_POINT('Ctrl Pts',(-27.0670307767398,7.18657585481396,36.8203372030951));
#33801=CARTESIAN_POINT('Ctrl Pts',(-22.6371118575503,6.99739878870591,36.2397466988013));
#33802=CARTESIAN_POINT('Ctrl Pts',(-18.3932178061842,6.82819742189185,35.0395940680358));
#33803=CARTESIAN_POINT('Ctrl Pts',(-14.4094498834431,6.66543158101024,33.2667925298684));
#33804=CARTESIAN_POINT('Ctrl Pts',(-10.6732059289801,6.50060855796851,31.0610971404567));
#33805=CARTESIAN_POINT('Ctrl Pts',(-7.29557708527982,6.32441606849526,28.3459245289215));
#33806=CARTESIAN_POINT('Ctrl Pts',(-4.35011979267042,6.12505774886043,25.1690331245211));
#33807=CARTESIAN_POINT('Ctrl Pts',(-2.1552924018102,5.93384517916791,22.1512975283732));
#33808=CARTESIAN_POINT('Ctrl Pts',(-0.934264384510294,5.79035915091665,
19.9576366206874));
#33809=CARTESIAN_POINT('Ctrl Pts',(-0.217066032849526,5.69001969995687,
18.4576188984149));
#33810=CARTESIAN_POINT('Ctrl Pts',(-0.0517570763689102,5.66551509710643,
18.0937381573601));
#33811=CARTESIAN_POINT('Ctrl Pts',(0.106095228629841,5.64071489355821,17.7275698974483));
#33812=CARTESIAN_POINT('Ctrl Pts',(-38.3661892429674,10.6050661536892,33.2823591784344));
#33813=CARTESIAN_POINT('Ctrl Pts',(-37.9671384846144,10.5777689837161,33.3854884036947));
#33814=CARTESIAN_POINT('Ctrl Pts',(-37.5647102405911,10.5506896266998,33.4818781105384));
#33815=CARTESIAN_POINT('Ctrl Pts',(-35.838584594256,10.4365567481294,33.8626670870572));
#33816=CARTESIAN_POINT('Ctrl Pts',(-33.1982305732567,10.2719415070743,34.2838556108487));
#33817=CARTESIAN_POINT('Ctrl Pts',(-29.2728489305625,10.0511774947007,34.4505393124499));
#33818=CARTESIAN_POINT('Ctrl Pts',(-24.7735462962233,9.81863871620139,34.1247592769514));
#33819=CARTESIAN_POINT('Ctrl Pts',(-20.423779822698,9.60967367489776,33.1767389206439));
#33820=CARTESIAN_POINT('Ctrl Pts',(-16.2972164409564,9.41153176383594,31.6489144657926));
#33821=CARTESIAN_POINT('Ctrl Pts',(-12.3884323729163,9.21500541081661,29.6800767690944));
#33822=CARTESIAN_POINT('Ctrl Pts',(-8.80083669338724,9.01175979868378,27.1886192523672));
#33823=CARTESIAN_POINT('Ctrl Pts',(-5.6076513402522,8.78956564702969,24.2178312637806));
#33824=CARTESIAN_POINT('Ctrl Pts',(-3.17445016977068,8.58124477590158,21.3626542097078));
#33825=CARTESIAN_POINT('Ctrl Pts',(-1.77705695674595,8.42762540105217,19.2666254426567));
#33826=CARTESIAN_POINT('Ctrl Pts',(-0.937912040084691,8.32086564673385,
17.8269442237021));
#33827=CARTESIAN_POINT('Ctrl Pts',(-0.74276181745419,8.29482075310626,17.476953167516));
#33828=CARTESIAN_POINT('Ctrl Pts',(-0.554631609392133,8.26849188852043,
17.1240221481785));
#33829=CARTESIAN_POINT('Ctrl Pts',(-41.0932888255619,13.6252616883324,29.7990058126645));
#33830=CARTESIAN_POINT('Ctrl Pts',(-40.6951709804398,13.5952855444977,29.926812980099));
#33831=CARTESIAN_POINT('Ctrl Pts',(-40.2933116112545,13.5655149131873,30.0481434512788));
#33832=CARTESIAN_POINT('Ctrl Pts',(-38.5680000299751,13.4398628522405,30.5361601005493));
#33833=CARTESIAN_POINT('Ctrl Pts',(-35.919675614011,13.2576618204372,31.122937703186));
#33834=CARTESIAN_POINT('Ctrl Pts',(-31.9544063765669,13.0115743729063,31.5403078753727));
#33835=CARTESIAN_POINT('Ctrl Pts',(-27.3756745048881,12.751644575675,31.5069624080352));
#33836=CARTESIAN_POINT('Ctrl Pts',(-22.9050004035097,12.5189796899122,30.8479170967634));
#33837=CARTESIAN_POINT('Ctrl Pts',(-18.6155631238519,12.301865256328,29.6004493920025));
#33838=CARTESIAN_POINT('Ctrl Pts',(-14.5100993266258,12.0904144587841,27.9023158041159));
#33839=CARTESIAN_POINT('Ctrl Pts',(-10.6832885815738,11.8774764455751,25.6660504730613));
#33840=CARTESIAN_POINT('Ctrl Pts',(-7.20797317660949,11.6504923923572,22.9297998250813));
#33841=CARTESIAN_POINT('Ctrl Pts',(-4.5033571253319,11.4410171343385,20.2591620206668));
#33842=CARTESIAN_POINT('Ctrl Pts',(-2.90518917804047,11.2882220371981,18.273624202455));
#33843=CARTESIAN_POINT('Ctrl Pts',(-1.92723052845132,11.1823584691134,16.9020932343301));
#33844=CARTESIAN_POINT('Ctrl Pts',(-1.69811217151328,11.1565388193505,16.5678840962628));
#33845=CARTESIAN_POINT('Ctrl Pts',(-1.47551448673721,11.1304479812224,16.2300888450915));
#33846=CARTESIAN_POINT('Ctrl Pts',(-43.607077734618,15.9398275064074,26.5881648420301));
#33847=CARTESIAN_POINT('Ctrl Pts',(-43.2097562832355,15.9092719019138,26.7376510428101));
#33848=CARTESIAN_POINT('Ctrl Pts',(-42.8083994921326,15.8789225535602,26.8808736318176));
#33849=CARTESIAN_POINT('Ctrl Pts',(-41.0839333013364,15.7507918597713,27.4629402111696));
#33850=CARTESIAN_POINT('Ctrl Pts',(-38.4288723650909,15.5646999212503,28.1949050547109));
#33851=CARTESIAN_POINT('Ctrl Pts',(-34.4291690696808,15.3133344724918,28.8319001558766));
#33852=CARTESIAN_POINT('Ctrl Pts',(-29.7816206639597,15.0487502016962,29.054528697458));
#33853=CARTESIAN_POINT('Ctrl Pts',(-25.2060188107135,14.8142492774957,28.648116309137));
#33854=CARTESIAN_POINT('Ctrl Pts',(-20.7751262600391,14.5991383033468,27.6453833399041));
#33855=CARTESIAN_POINT('Ctrl Pts',(-16.4987857843687,14.3930646018661,26.183231029547));
#33856=CARTESIAN_POINT('Ctrl Pts',(-12.4640832639393,14.1899609567462,24.168963069841));
#33857=CARTESIAN_POINT('Ctrl Pts',(-8.74353496671818,13.977122935371,21.6361869570784));
#33858=CARTESIAN_POINT('Ctrl Pts',(-5.80297495936802,13.7824369346935,19.1251989416204));
#33859=CARTESIAN_POINT('Ctrl Pts',(-4.03025747473542,13.6409944051188,17.2348975933744));
#33860=CARTESIAN_POINT('Ctrl Pts',(-2.9316130946012,13.5429643472183,15.9219687959923));
#33861=CARTESIAN_POINT('Ctrl Pts',(-2.67298639300328,13.5190447294408,15.6014060795513));
#33862=CARTESIAN_POINT('Ctrl Pts',(-2.42046701738913,13.4948677704672,15.2767757095819));
#33863=CARTESIAN_POINT('Ctrl Pts',(-46.600622033322,18.188947172369,22.7630606377021));
#33864=CARTESIAN_POINT('Ctrl Pts',(-46.2043140287326,18.1597316481657,22.9372716024946));
#33865=CARTESIAN_POINT('Ctrl Pts',(-45.8036618532788,18.1307342364494,23.1054387932091));
#33866=CARTESIAN_POINT('Ctrl Pts',(-44.0808392894361,18.0083786966032,23.794574813762));
#33867=CARTESIAN_POINT('Ctrl Pts',(-41.4191469418867,17.830846834045,24.6917945378714));
#33868=CARTESIAN_POINT('Ctrl Pts',(-37.3817973723991,17.5925027676131,25.5786367906797));
#33869=CARTESIAN_POINT('Ctrl Pts',(-32.6577288281998,17.3443426911773,26.0922604044553));
#33870=CARTESIAN_POINT('Ctrl Pts',(-27.9645205180292,17.1289494695207,25.9727307503254));
#33871=CARTESIAN_POINT('Ctrl Pts',(-23.3744766463726,16.9369213116231,25.2475009189749));
#33872=CARTESIAN_POINT('Ctrl Pts',(-18.9055289559508,16.7575317657622,24.0525348461015));
#33873=CARTESIAN_POINT('Ctrl Pts',(-14.6361364276617,16.5859876106103,22.2890423286866));
#33874=CARTESIAN_POINT('Ctrl Pts',(-10.6384560691178,16.4095763329362,19.9853865921915));
#33875=CARTESIAN_POINT('Ctrl Pts',(-7.43109834396335,16.2491906636996,17.6535628588228));
#33876=CARTESIAN_POINT('Ctrl Pts',(-5.46091214715191,16.1323920433636,15.8696510460116));
#33877=CARTESIAN_POINT('Ctrl Pts',(-4.22570859084968,16.0510402241362,14.6219906158099));
#33878=CARTESIAN_POINT('Ctrl Pts',(-3.93374351400571,16.0311583490605,14.3166984129188));
#33879=CARTESIAN_POINT('Ctrl Pts',(-3.64746550911542,16.01103806515,14.006873262723));
#33880=CARTESIAN_POINT('Ctrl Pts',(-49.3109039376438,19.7983627848149,19.2977258249977));
#33881=CARTESIAN_POINT('Ctrl Pts',(-48.9156505478665,19.7720645135703,19.4934389062555));
#33882=CARTESIAN_POINT('Ctrl Pts',(-48.5158032965208,19.7460021313493,19.6832775632098));
#33883=CARTESIAN_POINT('Ctrl Pts',(-46.795314972639,19.6361820466171,20.465343757841));
#33884=CARTESIAN_POINT('Ctrl Pts',(-44.1292133031455,19.4774394485581,21.5059848500062));
#33885=CARTESIAN_POINT('Ctrl Pts',(-40.0610920842694,19.2670183310104,22.6095856728884));
#33886=CARTESIAN_POINT('Ctrl Pts',(-35.2727034384221,19.0520629838802,23.3755210446417));
#33887=CARTESIAN_POINT('Ctrl Pts',(-30.4793692627444,18.8717166252608,23.5044879484745));
#33888=CARTESIAN_POINT('Ctrl Pts',(-25.7530104929066,18.7178122962125,23.0192735306984));
#33889=CARTESIAN_POINT('Ctrl Pts',(-21.1186127047416,18.5794411422907,22.0550466235913));
#33890=CARTESIAN_POINT('Ctrl Pts',(-16.6471314095342,18.4529446490623,20.5075853478614));
#33891=CARTESIAN_POINT('Ctrl Pts',(-12.4104243963383,18.3257380682571,18.4006076730228));
#33892=CARTESIAN_POINT('Ctrl Pts',(-8.97273113596811,18.2102139945187,16.2219895556944));
#33893=CARTESIAN_POINT('Ctrl Pts',(-6.83193517130343,18.1249152482566,14.5285728120039));
#33894=CARTESIAN_POINT('Ctrl Pts',(-5.47870989582417,18.064727637235,13.3362339645435));
#33895=CARTESIAN_POINT('Ctrl Pts',(-5.15799058549254,18.0499634327475,13.0439317858091));
#33896=CARTESIAN_POINT('Ctrl Pts',(-4.84265063443571,18.0349776243875,12.746749095832));
#33897=CARTESIAN_POINT('Ctrl Pts',(-51.2947920922114,20.6836496418694,16.758668506747));
#33898=CARTESIAN_POINT('Ctrl Pts',(-50.90049041867,20.6606519170286,16.9695486618146));
#33899=CARTESIAN_POINT('Ctrl Pts',(-50.5014277827748,20.6379063239872,17.1746607300667));
#33900=CARTESIAN_POINT('Ctrl Pts',(-48.7835507278465,20.5422448076096,18.0221667953519));
#33901=CARTESIAN_POINT('Ctrl Pts',(-46.1157541596014,20.4047755971079,19.1638130647008));
#33902=CARTESIAN_POINT('Ctrl Pts',(-42.0278763659724,20.225761668211,20.420052715765));
#33903=CARTESIAN_POINT('Ctrl Pts',(-37.1961968561338,20.0475517349526,21.3635952152001));
#33904=CARTESIAN_POINT('Ctrl Pts',(-32.3340808857814,19.9048724048602,21.6673350763271));
#33905=CARTESIAN_POINT('Ctrl Pts',(-27.5131912254386,19.790507905872,21.3506809605032));
#33906=CARTESIAN_POINT('Ctrl Pts',(-22.7635395442217,19.6935273080542,20.5482405652461));
#33907=CARTESIAN_POINT('Ctrl Pts',(-18.1507531781766,19.6110850660289,19.1518448697928));
#33908=CARTESIAN_POINT('Ctrl Pts',(-13.746490413364,19.530779076001,17.18184705429));
#33909=CARTESIAN_POINT('Ctrl Pts',(-10.1470937090947,19.4573327991495,15.1094559205455));
#33910=CARTESIAN_POINT('Ctrl Pts',(-7.88638509780635,19.4012238336331,13.4783919538666));
#33911=CARTESIAN_POINT('Ctrl Pts',(-6.45016872863384,19.3605693891818,12.3240081054347));
#33912=CARTESIAN_POINT('Ctrl Pts',(-6.10927013923073,19.3505226070412,12.0406358031095));
#33913=CARTESIAN_POINT('Ctrl Pts',(-5.77357313580776,19.3402634731691,11.7521626271329));
#33914=CARTESIAN_POINT('Ctrl Pts',(-52.4105767042207,21.117312799858,15.3299514418919));
#33915=CARTESIAN_POINT('Ctrl Pts',(-52.016860569711,21.0964267127388,15.5492448456817));
#33916=CARTESIAN_POINT('Ctrl Pts',(-51.6182931914354,21.0758020890032,15.7628245248212));
#33917=CARTESIAN_POINT('Ctrl Pts',(-49.9021313977145,20.9891913310095,16.6465912195786));
#33918=CARTESIAN_POINT('Ctrl Pts',(-47.2337840991246,20.8653273744228,17.8442101454984));
#33919=CARTESIAN_POINT('Ctrl Pts',(-43.1354771375862,20.7063681300896,19.1850388218609));
#33920=CARTESIAN_POINT('Ctrl Pts',(-38.280340820171,20.5515335415639,20.2269975195059));
#33921=CARTESIAN_POINT('Ctrl Pts',(-33.3805535763787,20.4326519806542,20.6275542276719));
#33922=CARTESIAN_POINT('Ctrl Pts',(-28.5076379384233,20.3430531321453,20.4042206960657));
#33923=CARTESIAN_POINT('Ctrl Pts',(-23.6944093857262,20.2718184169426,19.6912911988527));
#33924=CARTESIAN_POINT('Ctrl Pts',(-19.0035276350953,20.2165549432469,18.3783788785326));
#33925=CARTESIAN_POINT('Ctrl Pts',(-14.5065432410363,20.164982094833,16.4839472490078));
#33926=CARTESIAN_POINT('Ctrl Pts',(-10.8175964077287,20.117197691553,14.4700412096342));
#33927=CARTESIAN_POINT('Ctrl Pts',(-8.49044235789128,20.0788282397779,12.8732097710812));
#33928=CARTESIAN_POINT('Ctrl Pts',(-7.00822822710744,20.0500302875854,11.739623233971));
#33929=CARTESIAN_POINT('Ctrl Pts',(-6.65615891828568,20.0428451797642,11.4611482226922));
#33930=CARTESIAN_POINT('Ctrl Pts',(-6.30920577514685,20.0354515632684,11.1774559872003));
#33931=CARTESIAN_POINT('Ctrl Pts',(-52.7278698567105,21.2334813897109,14.9235928820212));
#33932=CARTESIAN_POINT('Ctrl Pts',(-52.3343225101278,21.2132228077857,15.1452703485296));
#33933=CARTESIAN_POINT('Ctrl Pts',(-51.9358984377363,21.1932283095702,15.36124888794));
#33934=CARTESIAN_POINT('Ctrl Pts',(-50.2202359374443,21.1093059289188,16.2552855690169));
#33935=CARTESIAN_POINT('Ctrl Pts',(-47.5517532779547,20.9894835119608,17.4687550424721));
#33936=CARTESIAN_POINT('Ctrl Pts',(-43.4505266608392,20.8364792943525,18.8335283196105));
#33937=CARTESIAN_POINT('Ctrl Pts',(-38.5887936562049,20.6885792302246,19.9033309706188));
#33938=CARTESIAN_POINT('Ctrl Pts',(-33.6783987418936,20.5767478260626,20.3312569091985));
#33939=CARTESIAN_POINT('Ctrl Pts',(-28.7908305503325,20.4944756050622,20.1342769298014));
#33940=CARTESIAN_POINT('Ctrl Pts',(-23.9597012807767,20.4308554028779,19.4465967898802));
#33941=CARTESIAN_POINT('Ctrl Pts',(-19.2468366897852,20.3836340081555,18.1571940901283));
#33942=CARTESIAN_POINT('Ctrl Pts',(-14.7237552627977,20.340580727313,16.2839937133523));
#33943=CARTESIAN_POINT('Ctrl Pts',(-11.0096023037979,20.3004356869138,14.2864756931423));
#33944=CARTESIAN_POINT('Ctrl Pts',(-8.66373522866924,20.2673681898868,12.6992039590105));
#33945=CARTESIAN_POINT('Ctrl Pts',(-7.16856047765098,20.2421246596599,11.5714116141598));
#33946=CARTESIAN_POINT('Ctrl Pts',(-6.81334606473223,20.2357981340653,11.2943015263024));
#33947=CARTESIAN_POINT('Ctrl Pts',(-6.46322607776776,20.2292648564311,11.0119422811286));
#33948=CARTESIAN_POINT('Ctrl Pts',(-53.0460482247937,21.3428689572265,14.5160304606263));
#33949=CARTESIAN_POINT('Ctrl Pts',(-52.6526722617868,21.323266505305,14.7400892699525));
#33950=CARTESIAN_POINT('Ctrl Pts',(-52.2543941113152,21.303930781031,14.9584636434814));
#33951=CARTESIAN_POINT('Ctrl Pts',(-50.5392422512964,21.2228186866547,15.862756102697));
#33952=CARTESIAN_POINT('Ctrl Pts',(-47.870642759627,21.1072213437662,17.0920520597779));
#33953=CARTESIAN_POINT('Ctrl Pts',(-43.7665309694762,20.9604400919523,18.4807247967744));
#33954=CARTESIAN_POINT('Ctrl Pts',(-38.8982526035527,20.819779963638,19.5783050883969));
#33955=CARTESIAN_POINT('Ctrl Pts',(-33.9773212172862,20.7152993064879,20.0335139845838));
#33956=CARTESIAN_POINT('Ctrl Pts',(-29.075197419158,20.6406553883908,19.8627783242788));
#33957=CARTESIAN_POINT('Ctrl Pts',(-24.226291838715,20.5849601975755,19.2002153983462));
#33958=CARTESIAN_POINT('Ctrl Pts',(-19.4916041416705,20.5461109852346,17.9341609933042));
#33959=CARTESIAN_POINT('Ctrl Pts',(-14.9426199184388,20.5119420676311,16.0819985993253));
#33960=CARTESIAN_POINT('Ctrl Pts',(-11.2034485633272,20.4797911688045,14.1006759877594));
#33961=CARTESIAN_POINT('Ctrl Pts',(-8.83899898851629,20.4522911786996,12.5228195121512));
#33962=CARTESIAN_POINT('Ctrl Pts',(-7.33094843090817,20.4307901345004,11.4007202313913));
#33963=CARTESIAN_POINT('Ctrl Pts',(-6.97261113714822,20.4253683033402,11.1249514482168));
#33964=CARTESIAN_POINT('Ctrl Pts',(-6.61934824302656,20.4197421663948,10.8439022877958));
#33965=CARTESIAN_POINT('',(-42.6061719181885,20.5529756002067,19.5442896711374));
#33966=CARTESIAN_POINT('Ctrl Pts',(-19.7766131277702,-3.27137127985417,
42.4988381903824));
#33967=CARTESIAN_POINT('Ctrl Pts',(-23.5152967093788,1.76302065360711,40.7590604194676));
#33968=CARTESIAN_POINT('Ctrl Pts',(-28.0269925336501,6.26298702224561,38.031741717945));
#33969=CARTESIAN_POINT('Ctrl Pts',(-34.3755322884386,12.51884027248,31.997404897986));
#33970=CARTESIAN_POINT('Ctrl Pts',(-36.3604480222897,14.4577038717082,29.7410619772352));
#33971=CARTESIAN_POINT('Ctrl Pts',(-39.8066816790496,17.8486390891638,24.9184712381644));
#33972=CARTESIAN_POINT('Ctrl Pts',(-41.3278638860567,19.3555621054309,22.33097742788));
#33973=CARTESIAN_POINT('Ctrl Pts',(-42.6061719181886,20.5529756002057,19.544289671137));
#33974=CARTESIAN_POINT('Ctrl Pts',(-13.0430026535592,19.9464420456703,15.9970821676198));
#33975=CARTESIAN_POINT('Ctrl Pts',(-17.5281049508455,20.0189549105364,18.3838569009211));
#33976=CARTESIAN_POINT('Ctrl Pts',(-22.4637387366771,20.0954766247834,19.8995121675166));
#33977=CARTESIAN_POINT('Ctrl Pts',(-32.54594053874,20.2752040736289,21.1067813092147));
#33978=CARTESIAN_POINT('Ctrl Pts',(-37.6925271019862,20.3824974081049,20.8003325400241));
#33979=CARTESIAN_POINT('Ctrl Pts',(-42.6061719181885,20.5529756002056,19.5442896711373));
#33980=CARTESIAN_POINT('Ctrl Pts',(-51.3108334676861,20.9435908393615,16.1511536729868));
#33981=CARTESIAN_POINT('Ctrl Pts',(-51.1733425720729,20.9358615047579,16.2234493647249));
#33982=CARTESIAN_POINT('Ctrl Pts',(-51.0358516764597,20.9281321701544,16.295745056463));
#33983=CARTESIAN_POINT('Ctrl Pts',(-50.8983607808465,20.9204028355509,16.3680407482011));
#33984=CARTESIAN_POINT('Ctrl Pts',(-37.1492712195272,20.1474693751975,23.5976099220123));
#33985=CARTESIAN_POINT('Ctrl Pts',(-19.3601378042676,20.0812550388979,21.8299835873915));
#33986=CARTESIAN_POINT('Ctrl Pts',(-7.20423930084636,19.8399463130827,12.1777561381709));
#33987=CARTESIAN_POINT('Ctrl Pts',(-51.3107798237275,20.9469886892296,16.1512322048296));
#33988=CARTESIAN_POINT('Ctrl Pts',(-51.1732906434227,20.9392720585054,16.2235357813434));
#33989=CARTESIAN_POINT('Ctrl Pts',(-51.0358014631179,20.9315554277811,16.2958393578572));
#33990=CARTESIAN_POINT('Ctrl Pts',(-50.8983122828131,20.9238387970569,16.368142934371));
#33991=CARTESIAN_POINT('Ctrl Pts',(-37.149394252333,20.1521757246323,23.5985005857523));
#33992=CARTESIAN_POINT('Ctrl Pts',(-19.3601421168584,20.0873688943554,21.8304317652129));
#33993=CARTESIAN_POINT('Ctrl Pts',(-7.20415446045915,19.8474084919615,12.1784397513226));
#33994=CARTESIAN_POINT('Ctrl Pts',(-51.310726179769,20.9503865390978,16.1513107366724));
#33995=CARTESIAN_POINT('Ctrl Pts',(-51.1732387147725,20.9426826122528,16.2236221979619));
#33996=CARTESIAN_POINT('Ctrl Pts',(-51.0357512497761,20.9349786854078,16.2959336592514));
#33997=CARTESIAN_POINT('Ctrl Pts',(-50.8982637847797,20.9272747585629,16.3682451205409));
#33998=CARTESIAN_POINT('Ctrl Pts',(-37.1495172851389,20.1568820740671,23.5993912494923));
#33999=CARTESIAN_POINT('Ctrl Pts',(-19.3601464294492,20.093482749813,21.8308799430342));
#34000=CARTESIAN_POINT('Ctrl Pts',(-7.20406962007193,19.8548706708402,12.1791233644742));
#34001=CARTESIAN_POINT('Ctrl Pts',(-51.3106725358104,20.9537843889659,16.1513892685152));
#34002=CARTESIAN_POINT('Ctrl Pts',(-51.1731867861224,20.9460931660003,16.2237086145804));
#34003=CARTESIAN_POINT('Ctrl Pts',(-51.0357010364343,20.9384019430346,16.2960279606456));
#34004=CARTESIAN_POINT('Ctrl Pts',(-50.8982152867463,20.9307107200689,16.3683473067109));
#34005=CARTESIAN_POINT('Ctrl Pts',(-37.1496403179447,20.1615884235019,23.6002819132323));
#34006=CARTESIAN_POINT('Ctrl Pts',(-19.36015074204,20.0995966052706,21.8313281208555));
#34007=CARTESIAN_POINT('Ctrl Pts',(-7.20398477968471,19.862332849719,12.1798069776258));
#34008=CARTESIAN_POINT('Ctrl Pts',(-51.3105096332532,20.9641027630587,16.1516277490143));
#34009=CARTESIAN_POINT('Ctrl Pts',(-51.1730290925045,20.9564501184246,16.2239710390642));
#34010=CARTESIAN_POINT('Ctrl Pts',(-51.0355485517558,20.9487974737906,16.2963143291142));
#34011=CARTESIAN_POINT('Ctrl Pts',(-50.898068011007,20.9411448291565,16.3686576191641));
#34012=CARTESIAN_POINT('Ctrl Pts',(-37.1500139361344,20.1758803657488,23.6029866241575));
#34013=CARTESIAN_POINT('Ctrl Pts',(-19.360163838241,20.1181627721728,21.8326891187219));
#34014=CARTESIAN_POINT('Ctrl Pts',(-7.20372714179975,19.8849935193208,12.1818829305098));
#34015=CARTESIAN_POINT('Ctrl Pts',(-51.3101838278559,20.9847395112521,16.1521047099983));
#34016=CARTESIAN_POINT('Ctrl Pts',(-51.1727137050801,20.9771640232786,16.2244958880224));
#34017=CARTESIAN_POINT('Ctrl Pts',(-51.0352435823044,20.9695885353052,16.2968870660465));
#34018=CARTESIAN_POINT('Ctrl Pts',(-50.8977734595286,20.9620130473318,16.3692782440705));
#34019=CARTESIAN_POINT('Ctrl Pts',(-37.1507611819551,20.2044642499886,23.6083960464791));
#34020=CARTESIAN_POINT('Ctrl Pts',(-19.3601900256785,20.1552951062578,21.8354111160267));
#34021=CARTESIAN_POINT('Ctrl Pts',(-7.20321186602976,19.9303148585245,12.1860348362777));
#34022=CARTESIAN_POINT('Ctrl Pts',(-51.3096951007816,21.0156946339229,16.1528201510927));
#34023=CARTESIAN_POINT('Ctrl Pts',(-51.1722406112913,21.0082348808134,16.2252831612052));
#34024=CARTESIAN_POINT('Ctrl Pts',(-51.034786121801,21.000775127704,16.2977461713177));
#34025=CARTESIAN_POINT('Ctrl Pts',(-50.8973316323108,20.9933153745945,16.3702091814302));
#34026=CARTESIAN_POINT('Ctrl Pts',(-37.151882683285,20.2473400636495,23.616510192681));
#34027=CARTESIAN_POINT('Ctrl Pts',(-19.3602290009807,20.2109936225946,21.8394942155879));
#34028=CARTESIAN_POINT('Ctrl Pts',(-7.20243895237484,19.9982968673298,12.1922626949296));
#34029=CARTESIAN_POINT('Ctrl Pts',(-51.3092063487451,21.0466497571015,16.1535355916576));
#34030=CARTESIAN_POINT('Ctrl Pts',(-51.1717675008611,21.0393057386868,16.226070434035));
#34031=CARTESIAN_POINT('Ctrl Pts',(-51.0343286529771,21.0319617202721,16.2986052764125));
#34032=CARTESIAN_POINT('Ctrl Pts',(-50.8968898050931,21.0246177018574,16.3711401187899));
#34033=CARTESIAN_POINT('Ctrl Pts',(-37.1530050166935,20.2902158603888,23.6246243565344));
#34034=CARTESIAN_POINT('Ctrl Pts',(-19.3602675711725,20.2666921589687,21.8435774500921));
#34035=CARTESIAN_POINT('Ctrl Pts',(-7.20166603871989,20.0662788761352,12.1984905535815));
#34036=CARTESIAN_POINT('Ctrl Pts',(-51.3088805014622,21.0672865061488,16.1540125517431));
#34037=CARTESIAN_POINT('Ctrl Pts',(-51.171452085513,21.0600196441101,16.2265952823942));
#34038=CARTESIAN_POINT('Ctrl Pts',(-51.0340236695638,21.0527527820714,16.2991780130453));
#34039=CARTESIAN_POINT('Ctrl Pts',(-50.8965952536146,21.0454859200326,16.3717607436964));
#34040=CARTESIAN_POINT('Ctrl Pts',(-37.1537536586921,20.3187997161584,23.6300338088058));
#34041=CARTESIAN_POINT('Ctrl Pts',(-19.3602930783192,20.3038245267329,21.8462996737943));
#34042=CARTESIAN_POINT('Ctrl Pts',(-7.20115076294994,20.1116002153389,12.2026424593494));
#34043=CARTESIAN_POINT('Ctrl Pts',(-51.3087175776821,21.0776048806767,16.154251031777));
#34044=CARTESIAN_POINT('Ctrl Pts',(-51.1712943777465,21.0703765968246,16.2268577065679));
#34045=CARTESIAN_POINT('Ctrl Pts',(-51.0338711778109,21.0631483129724,16.2994643813587));
#34046=CARTESIAN_POINT('Ctrl Pts',(-50.8964479778753,21.0559200291202,16.3720710561496));
#34047=CARTESIAN_POINT('Ctrl Pts',(-37.1541279843181,20.3330916439037,23.6327385352381));
#34048=CARTESIAN_POINT('Ctrl Pts',(-19.3603058292958,20.3223907107576,21.847660786348));
#34049=CARTESIAN_POINT('Ctrl Pts',(-7.20089312506496,20.1342608849406,12.2047184122334));
#34050=CARTESIAN_POINT('Ctrl Pts',(-51.3087018783124,21.0785991614118,16.1542740117631));
#34051=CARTESIAN_POINT('Ctrl Pts',(-51.171279180993,21.0713745949617,16.2268829938163));
#34052=CARTESIAN_POINT('Ctrl Pts',(-51.0338564836736,21.0641500285117,16.2994919758695));
#34053=CARTESIAN_POINT('Ctrl Pts',(-50.8964337863542,21.0569254620617,16.3721009579227));
#34054=CARTESIAN_POINT('Ctrl Pts',(-37.154164054414,20.3344688170607,23.6329991632448));
#34055=CARTESIAN_POINT('Ctrl Pts',(-19.3603070579826,20.3241797521467,21.8477919434393));
#34056=CARTESIAN_POINT('Ctrl Pts',(-7.20086829902429,20.1364444718193,12.204918451489));
#34057=CARTESIAN_POINT('Ctrl Pts',(-51.3086861789428,21.0795934421468,16.1542969917492));
#34058=CARTESIAN_POINT('Ctrl Pts',(-51.1712639842395,21.0723725930989,16.2269082810647));
#34059=CARTESIAN_POINT('Ctrl Pts',(-51.0338417895363,21.0651517440511,16.2995195703803));
#34060=CARTESIAN_POINT('Ctrl Pts',(-50.8964195948331,21.0579308950032,16.3721308596959));
#34061=CARTESIAN_POINT('Ctrl Pts',(-37.1542001245098,20.3358459902176,23.6332597912515));
#34062=CARTESIAN_POINT('Ctrl Pts',(-19.3603082866694,20.3259687935359,21.8479231005306));
#34063=CARTESIAN_POINT('Ctrl Pts',(-7.20084347298362,20.1386280586979,12.2051184907446));
#34064=CARTESIAN_POINT('Ctrl Pts',(-51.3086704795731,21.0805877228818,16.1543199717353));
#34065=CARTESIAN_POINT('Ctrl Pts',(-51.171248787486,21.0733705912361,16.2269335683132));
#34066=CARTESIAN_POINT('Ctrl Pts',(-51.033827095399,21.0661534595904,16.2995471648911));
#34067=CARTESIAN_POINT('Ctrl Pts',(-50.8964054033119,21.0589363279447,16.372160761469));
#34068=CARTESIAN_POINT('Ctrl Pts',(-37.1542361946057,20.3372231633746,23.6335204192581));
#34069=CARTESIAN_POINT('Ctrl Pts',(-19.3603095153562,20.327757834925,21.848054257622));
#34070=CARTESIAN_POINT('Ctrl Pts',(-7.20081864694295,20.1408116455766,12.2053185300001));
#34071=CARTESIAN_POINT('',(-42.6061719181885,20.5529756002067,19.5442896711374));
#34072=CARTESIAN_POINT('Ctrl Pts',(-44.4073194910718,21.2883239772394,-32.4663123587466));
#34073=CARTESIAN_POINT('Ctrl Pts',(-44.3383146796219,21.2711623310641,-32.0212557620871));
#34074=CARTESIAN_POINT('Ctrl Pts',(-44.261863066907,21.2542807820542,-31.5759157513107));
#34075=CARTESIAN_POINT('Ctrl Pts',(-43.9035132676456,21.1834525291307,-29.6749230164548));
#34076=CARTESIAN_POINT('Ctrl Pts',(-43.2061630172825,21.0834264338425,-26.8247770659076));
#34077=CARTESIAN_POINT('Ctrl Pts',(-41.7401377983077,20.9598507183575,-22.7530174393195));
#34078=CARTESIAN_POINT('Ctrl Pts',(-39.5700058445959,20.8461335954997,-18.2644080598691));
#34079=CARTESIAN_POINT('Ctrl Pts',(-36.8630486192783,20.7684839093916,-14.133595467843));
#34080=CARTESIAN_POINT('Ctrl Pts',(-33.6763829202324,20.7206230093664,-10.4064236844732));
#34081=CARTESIAN_POINT('Ctrl Pts',(-30.1365835892634,20.6916936542703,-7.02655419472538));
#34082=CARTESIAN_POINT('Ctrl Pts',(-26.1937522215189,20.6796111419738,-4.11120263465573));
#34083=CARTESIAN_POINT('Ctrl Pts',(-21.9057871986473,20.6722203558656,-1.70562443471912));
#34084=CARTESIAN_POINT('Ctrl Pts',(-18.0203164619706,20.6630225594897,-0.0137786889588934));
#34085=CARTESIAN_POINT('Ctrl Pts',(-15.3077264292458,20.6508204531822,0.853827525762252));
#34086=CARTESIAN_POINT('Ctrl Pts',(-13.4888993727121,20.6394053700742,1.33453354362263));
#34087=CARTESIAN_POINT('Ctrl Pts',(-13.0513753202763,20.6364191357732,1.44265992605398));
#34088=CARTESIAN_POINT('Ctrl Pts',(-12.6129206067808,20.6332209087108,1.54359234992982));
#34089=CARTESIAN_POINT('Ctrl Pts',(-44.5317392944723,21.2398788304839,-31.9470607245409));
#34090=CARTESIAN_POINT('Ctrl Pts',(-44.4608008352633,21.2217224127637,-31.5033401695429));
#34091=CARTESIAN_POINT('Ctrl Pts',(-44.3824197147887,21.2038412173392,-31.0593641751136));
#34092=CARTESIAN_POINT('Ctrl Pts',(-44.0158544499838,21.1287309618461,-29.1643130978913));
#34093=CARTESIAN_POINT('Ctrl Pts',(-43.3063638359009,21.0222253289507,-26.3240464492741));
#34094=CARTESIAN_POINT('Ctrl Pts',(-41.8236544645841,20.8890564489947,-22.2693004510702));
#34095=CARTESIAN_POINT('Ctrl Pts',(-39.6360777463142,20.7641817659416,-17.802927976306));
#34096=CARTESIAN_POINT('Ctrl Pts',(-36.9144982085081,20.6752847595175,-13.6971173002781));
#34097=CARTESIAN_POINT('Ctrl Pts',(-33.7164751020028,20.6159219251614,-9.99738737870817));
#34098=CARTESIAN_POINT('Ctrl Pts',(-30.1681646940186,20.5752144761384,-6.64672745320853));
#34099=CARTESIAN_POINT('Ctrl Pts',(-26.2206730087597,20.5509334123338,-3.76258061545188));
#34100=CARTESIAN_POINT('Ctrl Pts',(-21.9323370596648,20.5308579865904,-1.38988250425128));
#34101=CARTESIAN_POINT('Ctrl Pts',(-18.0496957203779,20.510426256151,0.272782902906163));
#34102=CARTESIAN_POINT('Ctrl Pts',(-15.3412263850242,20.4905046142392,1.12035027642913));
#34103=CARTESIAN_POINT('Ctrl Pts',(-13.5258914774281,20.4739374093561,1.58770978327916));
#34104=CARTESIAN_POINT('Ctrl Pts',(-13.0892415042887,20.469713411733,1.69263748736944));
#34105=CARTESIAN_POINT('Ctrl Pts',(-12.6516971675958,20.4652767483487,1.79037613603859));
#34106=CARTESIAN_POINT('Ctrl Pts',(-44.6561524410473,21.1822016013635,-31.4275844698422));
#34107=CARTESIAN_POINT('Ctrl Pts',(-44.5832693071228,21.1630886105529,-30.9852161369667));
#34108=CARTESIAN_POINT('Ctrl Pts',(-44.5029476284026,21.1442460408093,-30.5426209641973));
#34109=CARTESIAN_POINT('Ctrl Pts',(-44.1281197536622,21.0650173413637,-28.6535860555276));
#34110=CARTESIAN_POINT('Ctrl Pts',(-43.4064198561525,20.9522796229575,-25.8233136742122));
#34111=CARTESIAN_POINT('Ctrl Pts',(-41.9069320566516,20.8098799445818,-21.7857609610574));
#34112=CARTESIAN_POINT('Ctrl Pts',(-39.701810753245,20.6742608619688,-17.3418485850746));
#34113=CARTESIAN_POINT('Ctrl Pts',(-36.9655218819498,20.5745198093833,-13.2612876234125));
#34114=CARTESIAN_POINT('Ctrl Pts',(-33.7560682522845,20.5040526001987,-9.58928002469061));
#34115=CARTESIAN_POINT('Ctrl Pts',(-30.1991853983857,20.4519664047462,-6.26814546563906));
#34116=CARTESIAN_POINT('Ctrl Pts',(-26.2469871598986,20.4158956934967,-3.4155667301831));
#34117=CARTESIAN_POINT('Ctrl Pts',(-21.9582479010102,20.3835681705302,-1.07616408222921));
#34118=CARTESIAN_POINT('Ctrl Pts',(-18.0784131832276,20.3523071857454,0.55692401639258));
#34119=CARTESIAN_POINT('Ctrl Pts',(-15.3740496198733,20.3249607749065,1.38416737993585));
#34120=CARTESIAN_POINT('Ctrl Pts',(-13.5621950244834,20.3034475984546,1.83798684151568));
#34121=CARTESIAN_POINT('Ctrl Pts',(-13.126418050243,20.2980359714688,1.93966838129505));
#34122=CARTESIAN_POINT('Ctrl Pts',(-12.6897847127264,20.29241155197,2.03416478777318));
#34123=CARTESIAN_POINT('Ctrl Pts',(-45.1007065738908,20.942701117012,-29.5703976932599));
#34124=CARTESIAN_POINT('Ctrl Pts',(-45.0208376113571,20.9203083949833,-29.1329175650445));
#34125=CARTESIAN_POINT('Ctrl Pts',(-44.9335441184161,20.898168919688,-28.6953160815928));
#34126=CARTESIAN_POINT('Ctrl Pts',(-44.5290285228739,20.8048139743737,-26.8280477231251));
#34127=CARTESIAN_POINT('Ctrl Pts',(-43.7634624578871,20.6706999592586,-24.0339034229851));
#34128=CARTESIAN_POINT('Ctrl Pts',(-42.2036921823277,20.496623371127,-20.0584390264519));
#34129=CARTESIAN_POINT('Ctrl Pts',(-39.9355295569025,20.3241023157428,-15.6955948544318));
#34130=CARTESIAN_POINT('Ctrl Pts',(-37.1463732008804,20.1870685788371,-11.7061626846798));
#34131=CARTESIAN_POINT('Ctrl Pts',(-33.8958149948604,20.0783595881962,-8.13424084429036));
#34132=CARTESIAN_POINT('Ctrl Pts',(-30.3080800546265,19.9870599496472,-4.91976504399102));
#34133=CARTESIAN_POINT('Ctrl Pts',(-26.338894511269,19.9103458023656,-2.1813190929775));
#34134=CARTESIAN_POINT('Ctrl Pts',(-22.0485898350668,19.8358125374395,0.0375894018033821));
#34135=CARTESIAN_POINT('Ctrl Pts',(-18.1786911029417,19.767331746443,1.56354030718519));
#34136=CARTESIAN_POINT('Ctrl Pts',(-15.4889340993771,19.7145309927478,2.31712214152166));
#34137=CARTESIAN_POINT('Ctrl Pts',(-13.6894644921416,19.6760973304852,2.72185635616174));
#34138=CARTESIAN_POINT('Ctrl Pts',(-13.2568036731226,19.6666248028076,2.81176456048477));
#34139=CARTESIAN_POINT('Ctrl Pts',(-12.8234309753936,19.6569408091057,2.89449675536615));
#34140=CARTESIAN_POINT('Ctrl Pts',(-45.7331411798393,20.4780024533914,-26.9246386002418));
#34141=CARTESIAN_POINT('Ctrl Pts',(-45.643195587219,20.4514551579611,-26.4943263387457));
#34142=CARTESIAN_POINT('Ctrl Pts',(-45.545843383721,20.4251375618498,-26.0640525529226));
#34143=CARTESIAN_POINT('Ctrl Pts',(-45.0984865809081,20.3138746691076,-24.2287465356082));
#34144=CARTESIAN_POINT('Ctrl Pts',(-44.2696195687612,20.1526659052326,-21.4875728962292));
#34145=CARTESIAN_POINT('Ctrl Pts',(-42.6228530658995,19.938389785095,-17.602943244611));
#34146=CARTESIAN_POINT('Ctrl Pts',(-40.2636965799363,19.7189203495023,-13.3585242566371));
#34147=CARTESIAN_POINT('Ctrl Pts',(-37.3981974853228,19.5342279169114,-9.50204543905061));
#34148=CARTESIAN_POINT('Ctrl Pts',(-34.0882248338531,19.3763677050182,-6.07603571246518));
#34149=CARTESIAN_POINT('Ctrl Pts',(-30.4558249347077,19.2344308170631,-3.01699581468252));
#34150=CARTESIAN_POINT('Ctrl Pts',(-26.4619147472141,19.1049298841923,-0.444834180453594));
#34151=CARTESIAN_POINT('Ctrl Pts',(-22.1690568663997,18.9752993129734,1.5985252972521));
#34152=CARTESIAN_POINT('Ctrl Pts',(-18.313179789766,18.8580619466085,2.96837222878708));
#34153=CARTESIAN_POINT('Ctrl Pts',(-15.6442421074702,18.7718242877839,3.61460478820385));
#34154=CARTESIAN_POINT('Ctrl Pts',(-13.8624572105756,18.7111415689428,3.94779507422417));
#34155=CARTESIAN_POINT('Ctrl Pts',(-13.4342661174466,18.6963263828107,4.02053340451179));
#34156=CARTESIAN_POINT('Ctrl Pts',(-13.0055894034835,18.6812985797984,4.0861000036974));
#34157=CARTESIAN_POINT('Ctrl Pts',(-46.6541128225086,19.4355555088431,-23.0630467354439));
#34158=CARTESIAN_POINT('Ctrl Pts',(-46.5490340460232,19.4044605226273,-22.643764115916));
#34159=CARTESIAN_POINT('Ctrl Pts',(-46.4365715773658,19.3735658358572,-22.2247785892071));
#34160=CARTESIAN_POINT('Ctrl Pts',(-45.924844384654,19.2426748194849,-20.4387653247907));
#34161=CARTESIAN_POINT('Ctrl Pts',(-45.0008677782111,19.0517849995255,-17.7791175023364));
#34162=CARTESIAN_POINT('Ctrl Pts',(-43.2233772399451,18.7933185397158,-14.0338870045424));
#34163=CARTESIAN_POINT('Ctrl Pts',(-40.7274520428515,18.5218580841843,-9.97086024600777));
#34164=CARTESIAN_POINT('Ctrl Pts',(-37.7471256337672,18.2836948825759,-6.3177091993364));
#34165=CARTESIAN_POINT('Ctrl Pts',(-34.3476493922282,18.0697821020849,-3.11466407912025));
#34166=CARTESIAN_POINT('Ctrl Pts',(-30.6477975764489,17.8693333343866,-0.293061415310591));
#34167=CARTESIAN_POINT('Ctrl Pts',(-26.6162332687096,17.6778661310593,2.02512214074259));
#34168=CARTESIAN_POINT('Ctrl Pts',(-22.318832751704,17.4826662284719,3.80028746637419));
#34169=CARTESIAN_POINT('Ctrl Pts',(-18.4832621351138,17.3068805329357,4.93156172800206));
#34170=CARTESIAN_POINT('Ctrl Pts',(-15.844982677665,17.1802068447994,5.4136492325017));
#34171=CARTESIAN_POINT('Ctrl Pts',(-14.0893175584168,17.0925519552341,5.63740721935216));
#34172=CARTESIAN_POINT('Ctrl Pts',(-13.6677806909122,17.0712544126695,5.68386420748927));
#34173=CARTESIAN_POINT('Ctrl Pts',(-13.2461444261988,17.0497370990139,5.72313897790732));
#34174=CARTESIAN_POINT('Ctrl Pts',(-47.6918456308501,17.8320672383652,-18.704111982361));
#34175=CARTESIAN_POINT('Ctrl Pts',(-47.5691196189588,17.7976045693245,-18.29788404473));
#34176=CARTESIAN_POINT('Ctrl Pts',(-47.4390324745029,17.7633163796081,-17.8922819113841));
#34177=CARTESIAN_POINT('Ctrl Pts',(-46.8522106122062,17.6178640028275,-16.1648079219532));
#34178=CARTESIAN_POINT('Ctrl Pts',(-45.817282089803,17.4049846203341,-13.6018689231232));
#34179=CARTESIAN_POINT('Ctrl Pts',(-43.887284691588,17.1135517229592,-10.0217467329179));
#34180=CARTESIAN_POINT('Ctrl Pts',(-41.231769853489,16.8027253827761,-6.17336527532705));
#34181=CARTESIAN_POINT('Ctrl Pts',(-38.1173880411078,16.523022337621,-2.76065836727235));
#34182=CARTESIAN_POINT('Ctrl Pts',(-34.6133006485321,16.2641978724915,0.178767788703479));
#34183=CARTESIAN_POINT('Ctrl Pts',(-30.8344657346569,16.0157341831644,2.71962576869524));
#34184=CARTESIAN_POINT('Ctrl Pts',(-26.7585353322669,15.7719994721116,4.73743033545191));
#34185=CARTESIAN_POINT('Ctrl Pts',(-22.4552167350297,15.5202180684676,6.19524316069885));
#34186=CARTESIAN_POINT('Ctrl Pts',(-18.6426662536523,15.2931736272884,7.04407111501189));
#34187=CARTESIAN_POINT('Ctrl Pts',(-16.0396032563085,15.130708702949,7.33170692760031));
#34188=CARTESIAN_POINT('Ctrl Pts',(-14.3140107263472,15.0190926843839,7.42578042231738));
#34189=CARTESIAN_POINT('Ctrl Pts',(-13.9002119764642,14.9920326361705,7.44107757524737));
#34190=CARTESIAN_POINT('Ctrl Pts',(-13.4868340937886,14.9647422323135,7.44916755087306));
#34191=CARTESIAN_POINT('Ctrl Pts',(-48.6780895578841,15.7638142683891,-14.5547709237334));
#34192=CARTESIAN_POINT('Ctrl Pts',(-48.5377569832782,15.7283726072843,-14.1616824700076));
#34193=CARTESIAN_POINT('Ctrl Pts',(-48.3900841939855,15.6930928161318,-13.7695776325575));
#34194=CARTESIAN_POINT('Ctrl Pts',(-47.7283337492943,15.543379415412,-12.1012573581504));
#34195=CARTESIAN_POINT('Ctrl Pts',(-46.5827035062241,15.3241289383934,-9.63600324480673));
#34196=CARTESIAN_POINT('Ctrl Pts',(-44.5005407430779,15.0227233638938,-6.22259713508827));
#34197=CARTESIAN_POINT('Ctrl Pts',(-41.6857715265693,14.6988957424381,-2.59094464376435));
#34198=CARTESIAN_POINT('Ctrl Pts',(-38.4375620143823,14.4035050799014,0.578927699610593));
#34199=CARTESIAN_POINT('Ctrl Pts',(-34.8289423387839,14.1252237593235,3.25197397062977));
#34200=CARTESIAN_POINT('Ctrl Pts',(-30.9710627511194,13.8539516979883,5.50899869421461));
#34201=CARTESIAN_POINT('Ctrl Pts',(-26.8505025711077,13.5829362127958,7.22288800531011));
#34202=CARTESIAN_POINT('Ctrl Pts',(-22.5407609566498,13.2994842764397,8.35930998893307));
#34203=CARTESIAN_POINT('Ctrl Pts',(-18.7506147783617,13.0425486753816,8.92186191214317));
#34204=CARTESIAN_POINT('Ctrl Pts',(-16.1822241576763,12.8585920936854,9.01223170778387));
#34205=CARTESIAN_POINT('Ctrl Pts',(-14.4862987055291,12.7324540777387,8.97467844460437));
#34206=CARTESIAN_POINT('Ctrl Pts',(-14.0802223991229,12.7018988467546,8.95834926449915));
#34207=CARTESIAN_POINT('Ctrl Pts',(-13.6751669748553,12.6711030837425,8.93478984019534));
#34208=CARTESIAN_POINT('Ctrl Pts',(-49.6043543370422,13.2592937677246,-10.6555406574459));
#34209=CARTESIAN_POINT('Ctrl Pts',(-49.4465065543946,13.2252177231213,-10.2754480399043));
#34210=CARTESIAN_POINT('Ctrl Pts',(-49.281340174109,13.191306123502,-9.89672252517936));
#34211=CARTESIAN_POINT('Ctrl Pts',(-48.5450641799685,13.0474600457288,-8.2871658783874));
#34212=CARTESIAN_POINT('Ctrl Pts',(-47.2893340185595,12.8372075593629,-5.91905480535809));
#34213=CARTESIAN_POINT('Ctrl Pts',(-45.0558433901964,12.5484949329477,-2.6717513794037));
#34214=CARTESIAN_POINT('Ctrl Pts',(-42.0826999038725,12.2377054846042,0.7436212820901));
#34215=CARTESIAN_POINT('Ctrl Pts',(-38.7013965992381,11.9522310106351,3.67073641417757));
#34216=CARTESIAN_POINT('Ctrl Pts',(-34.9887969057865,11.6797819251771,6.0770574947467));
#34217=CARTESIAN_POINT('Ctrl Pts',(-31.0522615890383,11.4108111467242,8.04954156774515));
#34218=CARTESIAN_POINT('Ctrl Pts',(-26.887234235299,11.1374939458242,9.45832687893132));
#34219=CARTESIAN_POINT('Ctrl Pts',(-22.5709739096369,10.8473681096278,10.2716488305119));
#34220=CARTESIAN_POINT('Ctrl Pts',(-18.8029589072629,10.5820480444149,10.5460864286058));
#34221=CARTESIAN_POINT('Ctrl Pts',(-16.2689222255049,10.3910369789073,10.4377055494679));
#34222=CARTESIAN_POINT('Ctrl Pts',(-14.6024067670471,10.2599216927486,10.267460566929));
#34223=CARTESIAN_POINT('Ctrl Pts',(-14.2040678125169,10.2281653805015,10.2192687273159));
#34224=CARTESIAN_POINT('Ctrl Pts',(-13.8074239840703,10.1961599190035,10.1638445143716));
#34225=CARTESIAN_POINT('Ctrl Pts',(-50.4780231898425,10.420684636249,-6.97825636524223));
#34226=CARTESIAN_POINT('Ctrl Pts',(-50.3027554822726,10.3898269637342,-6.61091292266229));
#34227=CARTESIAN_POINT('Ctrl Pts',(-50.1201946638507,10.3591499865554,-6.24534398850934));
#34228=CARTESIAN_POINT('Ctrl Pts',(-49.3098403704687,10.2291883131935,-4.69370522484957));
#34229=CARTESIAN_POINT('Ctrl Pts',(-47.9446771541553,10.0401067219452,-2.42149658251557));
#34230=CARTESIAN_POINT('Ctrl Pts',(-45.5607908677836,9.78206378055234,0.661378115659448));
#34231=CARTESIAN_POINT('Ctrl Pts',(-42.4302660676023,9.50499638561923,3.86218206511734));
#34232=CARTESIAN_POINT('Ctrl Pts',(-38.9167256658903,9.24981780003299,6.5479222446764));
#34233=CARTESIAN_POINT('Ctrl Pts',(-35.1008412689809,9.00337535985762,8.68853775633541));
#34234=CARTESIAN_POINT('Ctrl Pts',(-31.0862039090992,8.75677479408939,10.3771954877894));
#34235=CARTESIAN_POINT('Ctrl Pts',(-26.8770707252232,8.50116890088297,11.4811916028238));
#34236=CARTESIAN_POINT('Ctrl Pts',(-22.5544391822955,8.22444592813344,11.9713059613016));
#34237=CARTESIAN_POINT('Ctrl Pts',(-18.8085260012426,7.96804930448713,11.95723852036));
#34238=CARTESIAN_POINT('Ctrl Pts',(-16.3087141317035,7.78162503245108,11.6496422404835));
#34239=CARTESIAN_POINT('Ctrl Pts',(-14.6714860069479,7.65323614745839,11.3463312647337));
#34240=CARTESIAN_POINT('Ctrl Pts',(-14.2809216999101,7.62212996336316,11.266226142876));
#34241=CARTESIAN_POINT('Ctrl Pts',(-13.8927906386079,7.59076668565169,11.1789266563201));
#34242=CARTESIAN_POINT('Ctrl Pts',(-51.2801101945885,7.18298363715391,-3.6058167721169));
#34243=CARTESIAN_POINT('Ctrl Pts',(-51.0875784709456,7.15763661423686,-3.25078129070187));
#34244=CARTESIAN_POINT('Ctrl Pts',(-50.887783992036,7.13250342173354,-2.89794609704175));
#34245=CARTESIAN_POINT('Ctrl Pts',(-50.0040661154971,7.02634360727853,-1.40250116902478));
#34246=CARTESIAN_POINT('Ctrl Pts',(-48.5305347456743,6.87350147707393,0.776364733400529));
#34247=CARTESIAN_POINT('Ctrl Pts',(-45.9977455159499,6.66841421880391,3.69838327624897));
#34248=CARTESIAN_POINT('Ctrl Pts',(-42.7114417935179,6.45075222930465,6.68844966589508));
#34249=CARTESIAN_POINT('Ctrl Pts',(-39.067072850966,6.25122984378583,9.13619723204205));
#34250=CARTESIAN_POINT('Ctrl Pts',(-35.1490911808322,6.05595707526583,11.0140071785515));
#34251=CARTESIAN_POINT('Ctrl Pts',(-31.0573490533695,5.8568061689083,12.4213387062058));
#34252=CARTESIAN_POINT('Ctrl Pts',(-26.8048536119047,5.64398234710963,13.2225300798875));
#34253=CARTESIAN_POINT('Ctrl Pts',(-22.476319035136,5.40587468584602,13.3908877176693));
#34254=CARTESIAN_POINT('Ctrl Pts',(-18.7527113449239,5.18017895256177,13.0891872008594));
#34255=CARTESIAN_POINT('Ctrl Pts',(-16.2871230511152,5.01301666232781,12.582706320691));
#34256=CARTESIAN_POINT('Ctrl Pts',(-14.6791349520876,4.89707445701614,12.1464642141551));
#34257=CARTESIAN_POINT('Ctrl Pts',(-14.2963869521683,4.86894780999335,12.0345319415383));
#34258=CARTESIAN_POINT('Ctrl Pts',(-13.9168603612279,4.84055053954568,11.9154972073634));
#34259=CARTESIAN_POINT('Ctrl Pts',(-52.0016295564212,3.57357815210241,-0.579903291299028));
#34260=CARTESIAN_POINT('Ctrl Pts',(-51.7920457954104,3.55599962931061,-0.236514691928469));
#34261=CARTESIAN_POINT('Ctrl Pts',(-51.5752339262503,3.53868515668548,0.104236780555091));
#34262=CARTESIAN_POINT('Ctrl Pts',(-50.6191007286354,3.46609807861293,1.54621396039117));
#34263=CARTESIAN_POINT('Ctrl Pts',(-49.0386135652145,3.36435917107101,3.63581403638429));
#34264=CARTESIAN_POINT('Ctrl Pts',(-46.3589071813945,3.23426720235262,6.40277838991865));
#34265=CARTESIAN_POINT('Ctrl Pts',(-42.9189723935365,3.10147907156715,9.1884915299686));
#34266=CARTESIAN_POINT('Ctrl Pts',(-39.1456956308945,2.98285053627008,11.4041304698817));
#34267=CARTESIAN_POINT('Ctrl Pts',(-35.1272894147124,2.86388130857434,13.024498250666));
#34268=CARTESIAN_POINT('Ctrl Pts',(-30.9599073841823,2.73730530568202,14.1554442054127));
#34269=CARTESIAN_POINT('Ctrl Pts',(-26.665243652355,2.59247375589619,14.6582371615255));
#34270=CARTESIAN_POINT('Ctrl Pts',(-22.3317156909432,2.41842603756845,14.5087087925182));
#34271=CARTESIAN_POINT('Ctrl Pts',(-18.6309936354684,2.24547053120763,13.9223283048296));
#34272=CARTESIAN_POINT('Ctrl Pts',(-16.1998803664798,2.11246131963295,13.2186916617235));
#34273=CARTESIAN_POINT('Ctrl Pts',(-14.6212528479762,2.01884144332686,12.6505786045591));
#34274=CARTESIAN_POINT('Ctrl Pts',(-14.2463818515635,1.99605339732081,12.5071362986838));
#34275=CARTESIAN_POINT('Ctrl Pts',(-13.8755492926242,1.9729679754383,12.3567453325002));
#34276=CARTESIAN_POINT('Ctrl Pts',(-52.5606120871006,0.237308438758995,
1.7568092319314));
#34277=CARTESIAN_POINT('Ctrl Pts',(-52.3365811493543,0.227921876287717,
2.09077303370513));
#34278=CARTESIAN_POINT('Ctrl Pts',(-52.1053556035498,0.218854274805993,
2.42171900485068));
#34279=CARTESIAN_POINT('Ctrl Pts',(-51.0879099056863,0.181679983795775,
3.82019619056501));
#34280=CARTESIAN_POINT('Ctrl Pts',(-49.4168749753258,0.133848323063104,
5.83677555706815));
#34281=CARTESIAN_POINT('Ctrl Pts',(-46.6128290745602,0.0830496793456984,
8.47584076816339));
#34282=CARTESIAN_POINT('Ctrl Pts',(-43.042935990631,0.0403924264632703,
11.0919484184786));
#34283=CARTESIAN_POINT('Ctrl Pts',(-39.1607220282688,0.00837005963384143,
13.1138268621901));
#34284=CARTESIAN_POINT('Ctrl Pts',(-35.057611354433,-0.0279539839125438,
14.5183472740695));
#34285=CARTESIAN_POINT('Ctrl Pts',(-30.8266189755247,-0.0750512999789021,
15.4169100192373));
#34286=CARTESIAN_POINT('Ctrl Pts',(-26.4968422963745,-0.14423024726241,
15.6680790196882));
#34287=CARTESIAN_POINT('Ctrl Pts',(-22.1598678274238,-0.245792879606331,
15.2498574169528));
#34288=CARTESIAN_POINT('Ctrl Pts',(-18.479339761014,-0.358291148292244,
14.4224610081486));
#34289=CARTESIAN_POINT('Ctrl Pts',(-16.0780703993592,-0.451704594358635,
13.551672433831));
#34290=CARTESIAN_POINT('Ctrl Pts',(-14.5247726836695,-0.519340602547392,
12.8716869099791));
#34291=CARTESIAN_POINT('Ctrl Pts',(-14.1567035816969,-0.535923052101836,
12.7015674050379));
#34292=CARTESIAN_POINT('Ctrl Pts',(-13.7933819214922,-0.552841667182328,
12.5246829031289));
#34293=CARTESIAN_POINT('Ctrl Pts',(-52.890754328659,-2.14030259993981,3.13037102927048));
#34294=CARTESIAN_POINT('Ctrl Pts',(-52.657228107773,-2.14321532053782,3.45848437102345));
#34295=CARTESIAN_POINT('Ctrl Pts',(-52.4165290093469,-2.14576465810466,
3.78332769304311));
#34296=CARTESIAN_POINT('Ctrl Pts',(-51.3587858092243,-2.15494826818845,
5.15466604875529));
#34297=CARTESIAN_POINT('Ctrl Pts',(-49.6282458760827,-2.16016260296573,
7.12536059420484));
#34298=CARTESIAN_POINT('Ctrl Pts',(-46.7425200714405,-2.1481556077715,9.68318376842775));
#34299=CARTESIAN_POINT('Ctrl Pts',(-43.0873089005232,-2.11918777525101,
12.1907133889699));
#34300=CARTESIAN_POINT('Ctrl Pts',(-39.1336679603413,-2.08197924289826,
14.0876535838583));
#34301=CARTESIAN_POINT('Ctrl Pts',(-34.9751571205844,-2.05170003121316,
15.3522532943094));
#34302=CARTESIAN_POINT('Ctrl Pts',(-30.7027227640134,-2.03426137368081,
16.0996671248213));
#34303=CARTESIAN_POINT('Ctrl Pts',(-26.3503698404099,-2.04135770257883,
16.1866083095668));
#34304=CARTESIAN_POINT('Ctrl Pts',(-22.0117968234591,-2.08278583441843,
15.5925376255057));
#34305=CARTESIAN_POINT('Ctrl Pts',(-18.345239938277,-2.14471303148954,14.6071159445911));
#34306=CARTESIAN_POINT('Ctrl Pts',(-15.9641459641279,-2.20477046252904,
13.6265599022038));
#34307=CARTESIAN_POINT('Ctrl Pts',(-14.4278995707152,-2.25046208753918,
12.8730584763167));
#34308=CARTESIAN_POINT('Ctrl Pts',(-14.0644019743396,-2.26180965939547,
12.6854345106128));
#34309=CARTESIAN_POINT('Ctrl Pts',(-13.7061209153785,-2.27353152926925,
12.4911916848406));
#34310=CARTESIAN_POINT('Ctrl Pts',(-53.1032912039355,-3.83428286431684,
4.01176084911006));
#34311=CARTESIAN_POINT('Ctrl Pts',(-52.8632528626129,-3.83237339034492,
4.33600459105002));
#34312=CARTESIAN_POINT('Ctrl Pts',(-52.6160567145443,-3.83006698099443,
4.65680426763478));
#34313=CARTESIAN_POINT('Ctrl Pts',(-51.530678565802,-3.81839846831683,6.01013065392125));
#34314=CARTESIAN_POINT('Ctrl Pts',(-49.759334630619,-3.79185933798401,7.95023150514814));
#34315=CARTESIAN_POINT('Ctrl Pts',(-46.8176122011927,-3.73301479320489,
10.4535182943327));
#34316=CARTESIAN_POINT('Ctrl Pts',(-43.1039324419476,-3.65055513724086,
12.8878101932113));
#34317=CARTESIAN_POINT('Ctrl Pts',(-39.1013809514705,-3.56151400652134,
14.7001087066328));
#34318=CARTESIAN_POINT('Ctrl Pts',(-34.9049930164177,-3.48120332570528,
15.8696164243301));
#34319=CARTESIAN_POINT('Ctrl Pts',(-30.6042940209659,-3.41513875248544,
16.5141034371326));
#34320=CARTESIAN_POINT('Ctrl Pts',(-26.2366723205577,-3.37526128513496,
16.4889878616773));
#34321=CARTESIAN_POINT('Ctrl Pts',(-21.8972872475658,-3.37099617994084,
15.7747435778838));
#34322=CARTESIAN_POINT('Ctrl Pts',(-18.2406096187147,-3.39437469848804,
14.6812175248876));
#34323=CARTESIAN_POINT('Ctrl Pts',(-15.8735908020004,-3.42893690611626,
13.6255049859516));
#34324=CARTESIAN_POINT('Ctrl Pts',(-14.3492100804318,-3.45783930783476,
12.8216495280743));
#34325=CARTESIAN_POINT('Ctrl Pts',(-13.9888888382134,-3.46518513130081,
12.622048154141));
#34326=CARTESIAN_POINT('Ctrl Pts',(-13.6341053234284,-3.47293757911652,
12.4159397012604));
#34327=CARTESIAN_POINT('Ctrl Pts',(-53.1601903434721,-4.30636894546118,
4.2473972842643));
#34328=CARTESIAN_POINT('Ctrl Pts',(-52.9183653507488,-4.3031084050989,4.57059999598952));
#34329=CARTESIAN_POINT('Ctrl Pts',(-52.6693862245725,-4.29944065268701,
4.89031068574757));
#34330=CARTESIAN_POINT('Ctrl Pts',(-51.5764222971609,-4.28192251284736,
6.23878159611758));
#34331=CARTESIAN_POINT('Ctrl Pts',(-49.7938739335711,-4.24645759656194,
8.1706048791254));
#34332=CARTESIAN_POINT('Ctrl Pts',(-46.8367693381174,-4.17439213330946,
10.6590570403307));
#34333=CARTESIAN_POINT('Ctrl Pts',(-43.1070263635738,-4.07676875425951,
13.0733547091991));
#34334=CARTESIAN_POINT('Ctrl Pts',(-39.0910430470873,-3.97294922980807,
14.8624751290696));
#34335=CARTESIAN_POINT('Ctrl Pts',(-34.8842670257438,-3.87828739688684,
16.0058968704492));
#34336=CARTESIAN_POINT('Ctrl Pts',(-30.5758354149997,-3.79820251809058,
16.6221317740867));
#34337=CARTESIAN_POINT('Ctrl Pts',(-26.2040674843958,-3.74469501429227,
16.5662546574962));
#34338=CARTESIAN_POINT('Ctrl Pts',(-21.8645183078476,-3.72710099262819,
15.8190437354006));
#34339=CARTESIAN_POINT('Ctrl Pts',(-18.210605270362,-3.7392015362719,14.6958994891422));
#34340=CARTESIAN_POINT('Ctrl Pts',(-15.8474815123186,-3.76629674044718,
13.6196193253719));
#34341=CARTESIAN_POINT('Ctrl Pts',(-14.3263754116638,-3.79028538091932,
12.8019944646511));
#34342=CARTESIAN_POINT('Ctrl Pts',(-13.9669291566427,-3.79646095010219,
12.5991202663822));
#34343=CARTESIAN_POINT('Ctrl Pts',(-13.6131076449932,-3.80305340259771,
12.3897718290191));
#34344=CARTESIAN_POINT('Ctrl Pts',(-53.215160241902,-4.78145508078572,4.47472655383311));
#34345=CARTESIAN_POINT('Ctrl Pts',(-52.9715659541889,-4.77682808742727,
4.79691749644181));
#34346=CARTESIAN_POINT('Ctrl Pts',(-52.7208204637783,-4.7717826224726,5.11556900438931));
#34347=CARTESIAN_POINT('Ctrl Pts',(-51.62033837218,-4.74834091216943,6.45931390625469));
#34348=CARTESIAN_POINT('Ctrl Pts',(-49.826681616631,-4.70381966688121,8.38304978791861));
#34349=CARTESIAN_POINT('Ctrl Pts',(-46.8543205172875,-4.61828583278682,
10.8569290710769));
#34350=CARTESIAN_POINT('Ctrl Pts',(-43.1086432890248,-4.50515190400754,
13.2515130774504));
#34351=CARTESIAN_POINT('Ctrl Pts',(-39.0793411611953,-4.38613315046716,
15.0177107421923));
#34352=CARTESIAN_POINT('Ctrl Pts',(-34.8622778213812,-4.27662792828432,
16.1352883928939));
#34353=CARTESIAN_POINT('Ctrl Pts',(-30.5462074145363,-4.18197237106197,
16.7235169409871));
#34354=CARTESIAN_POINT('Ctrl Pts',(-26.1703739293047,-4.11421750462538,
16.6371432586749));
#34355=CARTESIAN_POINT('Ctrl Pts',(-21.8307192732995,-4.08262421860679,
15.8572735488346));
#34356=CARTESIAN_POINT('Ctrl Pts',(-18.179597184834,-4.0828488851085,14.7048258212658));
#34357=CARTESIAN_POINT('Ctrl Pts',(-15.8203637738754,-4.10207414795096,
13.6082204427389));
#34358=CARTESIAN_POINT('Ctrl Pts',(-14.3025195588351,-4.12088738197538,
12.776999220031));
#34359=CARTESIAN_POINT('Ctrl Pts',(-13.9439433330175,-4.12583098108427,
12.5708945965306));
#34360=CARTESIAN_POINT('Ctrl Pts',(-13.5910770012361,-4.13120272145022,
12.3583493234692));
#34361=CARTESIAN_POINT('',(-41.8541565650246,20.7105311502984,-21.1067383182144));
#34362=CARTESIAN_POINT('Ctrl Pts',(-41.8541606617387,20.7105314630301,-21.1067474351839));
#34363=CARTESIAN_POINT('Ctrl Pts',(-39.7295427826956,20.5483441672165,-16.3785508491963));
#34364=CARTESIAN_POINT('Ctrl Pts',(-36.6735238440582,20.4520245495079,-12.0795659696835));
#34365=CARTESIAN_POINT('Ctrl Pts',(-29.2347502694402,20.3052748660675,-4.861962389441));
#34366=CARTESIAN_POINT('Ctrl Pts',(-24.8528638925488,20.248474007324,-1.94033620546688));
#34367=CARTESIAN_POINT('Ctrl Pts',(-20.067365612881,20.1925493450898,0.0414315931501192));
#34368=CARTESIAN_POINT('',(-45.5574401880941,-3.27137091447505,11.0356095483923));
#34369=CARTESIAN_POINT('Ctrl Pts',(-41.8541565650195,20.7105311502992,-21.1067383182116));
#34370=CARTESIAN_POINT('Ctrl Pts',(-43.2784775859439,19.9641948262067,-18.2823438856532));
#34371=CARTESIAN_POINT('Ctrl Pts',(-44.3685065694085,18.7336174322537,-15.3991351590888));
#34372=CARTESIAN_POINT('Ctrl Pts',(-46.0288074700108,15.6437709263416,-9.45081981765083));
#34373=CARTESIAN_POINT('Ctrl Pts',(-46.544980861968,13.6706054953477,-6.29727873979032));
#34374=CARTESIAN_POINT('Ctrl Pts',(-46.9598955651361,9.45712578015162,-0.478364493721878));
#34375=CARTESIAN_POINT('Ctrl Pts',(-46.8862235035279,7.18268855808127,2.2621291923848));
#34376=CARTESIAN_POINT('Ctrl Pts',(-46.3912855803782,2.26699026933625,7.13843410632294));
#34377=CARTESIAN_POINT('Ctrl Pts',(-45.9810130440977,-0.365223992195544,
9.28700597763431));
#34378=CARTESIAN_POINT('Ctrl Pts',(-45.5574400014258,-3.27137053313469,
11.0356101369551));
#34379=CARTESIAN_POINT('Ctrl Pts',(-45.5574399163743,-3.27137100135121,
11.0356091539468));
#34380=CARTESIAN_POINT('Ctrl Pts',(-44.9166357013057,-3.25992112204952,
11.4745151676869));
#34381=CARTESIAN_POINT('Ctrl Pts',(-44.261681176221,-3.24789096533568,11.8872675855542));
#34382=CARTESIAN_POINT('Ctrl Pts',(-43.5942284150339,-3.23555894384663,
12.2734886145391));
#34383=CARTESIAN_POINT('Ctrl Pts',(-41.9596126991115,-3.2053573815679,13.2193577464244));
#34384=CARTESIAN_POINT('Ctrl Pts',(-40.2500354155345,-3.17334534347451,
14.0060973871022));
#34385=CARTESIAN_POINT('Ctrl Pts',(-38.4898291965579,-3.14345008158506,
14.6282917586553));
#34386=CARTESIAN_POINT('Ctrl Pts',(-37.3163583243798,-3.12351990598108,
15.0430880273988));
#34387=CARTESIAN_POINT('Ctrl Pts',(-36.1203857008334,-3.10453051989493,
15.3847530580121));
#34388=CARTESIAN_POINT('Ctrl Pts',(-34.9091314157924,-3.08752071373525,
15.6517249226301));
#34389=CARTESIAN_POINT('Ctrl Pts',(-33.6978771313855,-3.07051090758448,
15.9186967871083));
#34390=CARTESIAN_POINT('Ctrl Pts',(-32.4713411854945,-3.0554806813514,16.110975485675));
#34391=CARTESIAN_POINT('Ctrl Pts',(-31.2367458399556,-3.04339100491456,
16.2270169755245));
#34392=CARTESIAN_POINT('Ctrl Pts',(-29.3848528239486,-3.02525649028182,
16.4010792100824));
#34393=CARTESIAN_POINT('Ctrl Pts',(-27.5148261587893,-3.01373821257335,
16.4036077255193));
#34394=CARTESIAN_POINT('Ctrl Pts',(-25.6510314119391,-3.01128625574909,
16.2295094149015));
#34395=CARTESIAN_POINT('Ctrl Pts',(-24.4085015836232,-3.00965161787009,
16.1134438747622));
#34396=CARTESIAN_POINT('Ctrl Pts',(-23.1687414966973,-3.01204645592803,
15.918877523405));
#34397=CARTESIAN_POINT('Ctrl Pts',(-21.9389594448249,-3.01891855380822,
15.6443269212343));
#34398=CARTESIAN_POINT('Ctrl Pts',(-20.70917754041,-3.02579065086441,15.3697763519838));
#34399=CARTESIAN_POINT('Ctrl Pts',(-19.4893736686176,-3.03714000665748,
15.0152415511123));
#34400=CARTESIAN_POINT('Ctrl Pts',(-18.2867431495384,-3.05321938564873,
14.5792465784353));
#34401=CARTESIAN_POINT('Ctrl Pts',(-17.7911796469897,-3.05984515577954,
14.3995877452977));
#34402=CARTESIAN_POINT('Ctrl Pts',(-17.2985321692438,-3.06727406915266,
14.2060970869875));
#34403=CARTESIAN_POINT('Ctrl Pts',(-16.809302921024,-3.07550335254719,13.9986721479021));
#34404=CARTESIAN_POINT('Ctrl Pts',(-53.2550241076282,-4.68328060676847,
4.62744272080562));
#34405=CARTESIAN_POINT('Ctrl Pts',(-53.0102407077981,-4.67927906663786,
4.9503893548096));
#34406=CARTESIAN_POINT('Ctrl Pts',(-52.7582576936744,-4.67486342687383,
5.26975370936434));
#34407=CARTESIAN_POINT('Ctrl Pts',(-51.655544643172,-4.65418501649615,6.6123848263081));
#34408=CARTESIAN_POINT('Ctrl Pts',(-49.8600436026871,-4.61395560865182,
8.53249843791617));
#34409=CARTESIAN_POINT('Ctrl Pts',(-46.8850762930286,-4.53496565777432,
11.0007825140162));
#34410=CARTESIAN_POINT('Ctrl Pts',(-43.1365657964198,-4.42959393838223,
13.3886632292394));
#34411=CARTESIAN_POINT('Ctrl Pts',(-39.1047177769365,-4.31850354734918,
15.1479551320865));
#34412=CARTESIAN_POINT('Ctrl Pts',(-34.8854383833948,-4.2170896233612,16.2584454359381));
#34413=CARTESIAN_POINT('Ctrl Pts',(-30.5674377343485,-4.13063759391767,
16.8394400005655));
#34414=CARTESIAN_POINT('Ctrl Pts',(-26.1900645771467,-4.07121155600733,
16.7456659202151));
#34415=CARTESIAN_POINT('Ctrl Pts',(-21.8493056943788,-4.04803120464602,
15.9582493147047));
#34416=CARTESIAN_POINT('Ctrl Pts',(-18.1975571114897,-4.055480889925,14.7992430763966));
#34417=CARTESIAN_POINT('Ctrl Pts',(-15.8381298955582,-4.07952578289679,
13.698223661129));
#34418=CARTESIAN_POINT('Ctrl Pts',(-14.3182865449456,-4.10152925776619,
12.8630191402326));
#34419=CARTESIAN_POINT('Ctrl Pts',(-13.9578284677764,-4.1072571624472,12.6550855609606));
#34420=CARTESIAN_POINT('Ctrl Pts',(-13.6031599189745,-4.11341014061892,
12.4406557045438));
#34421=CARTESIAN_POINT('Ctrl Pts',(-53.1870621995371,-4.24009445412503,
4.34532464343756));
#34422=CARTESIAN_POINT('Ctrl Pts',(-52.9441663261533,-4.23725223817857,
4.66946739029586));
#34423=CARTESIAN_POINT('Ctrl Pts',(-52.6940654070999,-4.23400446880359,
4.99008143969754));
#34424=CARTESIAN_POINT('Ctrl Pts',(-51.5993293700175,-4.21832863439708,
6.33826150780282));
#34425=CARTESIAN_POINT('Ctrl Pts',(-49.8156106685733,-4.18572164472913,
8.26773769630283));
#34426=CARTESIAN_POINT('Ctrl Pts',(-46.8568510448354,-4.11799618192084,
10.7525697593713));
#34427=CARTESIAN_POINT('Ctrl Pts',(-43.1253084596183,-4.02550335874969,
13.1625385894897));
#34428=CARTESIAN_POINT('Ctrl Pts',(-39.1077078270931,-3.92690475481451,
14.9472114885605));
#34429=CARTESIAN_POINT('Ctrl Pts',(-34.8995234161583,-3.83755718932749,
16.0860839457906));
#34430=CARTESIAN_POINT('Ctrl Pts',(-30.589864068293,-3.76285616468038,16.6976922413632));
#34431=CARTESIAN_POINT('Ctrl Pts',(-26.2171128932958,-3.71481495977278,
16.6371028524245));
#34432=CARTESIAN_POINT('Ctrl Pts',(-21.8768503613734,-3.70275434803773,
15.8851071811083));
#34433=CARTESIAN_POINT('Ctrl Pts',(-18.2225224734843,-3.71962751323487,
14.7578178297532));
#34434=CARTESIAN_POINT('Ctrl Pts',(-15.8592594973308,-3.74992063397164,
13.6787524066036));
#34435=CARTESIAN_POINT('Ctrl Pts',(-14.3361562667453,-3.77604797989279,
12.8582381071574));
#34436=CARTESIAN_POINT('Ctrl Pts',(-13.974817866806,-3.78276245762616,12.6538069497816));
#34437=CARTESIAN_POINT('Ctrl Pts',(-13.6191764391839,-3.78989370687861,
12.4428410361005));
#34438=CARTESIAN_POINT('Ctrl Pts',(-53.1177874295843,-3.80075287541765,
4.05749922158663));
#34439=CARTESIAN_POINT('Ctrl Pts',(-52.8767867368435,-3.79905339336963,
4.38285827146066));
#34440=CARTESIAN_POINT('Ctrl Pts',(-52.6285750022794,-3.79695621683146,
4.7047423894142));
#34441=CARTESIAN_POINT('Ctrl Pts',(-51.541843702939,-3.78620663871065,6.05855883565579));
#34442=CARTESIAN_POINT('Ctrl Pts',(-49.7699443207133,-3.76109400159902,
7.99752044121646));
#34443=CARTESIAN_POINT('Ctrl Pts',(-46.8274357987597,-3.70440674399875,
10.4990527223183));
#34444=CARTESIAN_POINT('Ctrl Pts',(-43.1129011207827,-3.62448835210827,
12.9312507195699));
#34445=CARTESIAN_POINT('Ctrl Pts',(-39.1095812653897,-3.53802316526296,
14.7414040548252));
#34446=CARTESIAN_POINT('Ctrl Pts',(-34.9125240042515,-3.46032715355504,
15.9087253564222));
#34447=CARTESIAN_POINT('Ctrl Pts',(-30.6112411258892,-3.39690914788247,
16.5509976263655));
#34448=CARTESIAN_POINT('Ctrl Pts',(-26.2431498662277,-3.35971861494906,
16.5236373449463));
#34449=CARTESIAN_POINT('Ctrl Pts',(-21.9034199271629,-3.35817927654809,
15.8071251099738));
#34450=CARTESIAN_POINT('Ctrl Pts',(-18.2465365368635,-3.38391914529348,
14.7116415712368));
#34451=CARTESIAN_POINT('Ctrl Pts',(-15.879443166288,-3.42007079724739,13.6546163643265));
#34452=CARTESIAN_POINT('Ctrl Pts',(-14.3530780248134,-3.45006162272336,
12.8488621843749));
#34453=CARTESIAN_POINT('Ctrl Pts',(-13.990857400756,-3.45770043113048,12.6479516105235));
#34454=CARTESIAN_POINT('Ctrl Pts',(-13.6342398281543,-3.46574819271174,
12.4404689854205));
#34455=CARTESIAN_POINT('Ctrl Pts',(-52.8689004777194,-2.2653457359543,3.02246760313475));
#34456=CARTESIAN_POINT('Ctrl Pts',(-52.6346047659193,-2.26761569662348,
3.35218985314796));
#34457=CARTESIAN_POINT('Ctrl Pts',(-52.3930760318627,-2.26951335386862,
3.67862619991285));
#34458=CARTESIAN_POINT('Ctrl Pts',(-51.3346585498217,-2.27586002752392,
5.05262899676798));
#34459=CARTESIAN_POINT('Ctrl Pts',(-49.6045518529517,-2.27671432942662,
7.02547485602001));
#34460=CARTESIAN_POINT('Ctrl Pts',(-46.7194808240327,-2.25814179129592,
9.58643472149431));
#34461=CARTESIAN_POINT('Ctrl Pts',(-43.0650395670317,-2.2214798205824,12.0975139363354));
#34462=CARTESIAN_POINT('Ctrl Pts',(-39.1121771246984,-2.17652897108851,
13.9978620983042));
#34463=CARTESIAN_POINT('Ctrl Pts',(-34.9544569047753,-2.13845241575724,
15.2657254601391));
#34464=CARTESIAN_POINT('Ctrl Pts',(-30.6828258526428,-2.11316923258448,
16.0162881999903));
#34465=CARTESIAN_POINT('Ctrl Pts',(-26.3312963999019,-2.11235831802136,
16.1062368873549));
#34466=CARTESIAN_POINT('Ctrl Pts',(-21.9935755581312,-2.14581153060268,
15.5150394164916));
#34467=CARTESIAN_POINT('Ctrl Pts',(-18.327773585856,-2.20085463389179,14.5319934262389));
#34468=CARTESIAN_POINT('Ctrl Pts',(-15.9472027453685,-2.25628908058851,
13.5529671676988));
#34469=CARTESIAN_POINT('Ctrl Pts',(-14.4093368232033,-2.29898278275007,
12.799490048317));
#34470=CARTESIAN_POINT('Ctrl Pts',(-14.0440004582171,-2.30966173471912,
12.6110582357232));
#34471=CARTESIAN_POINT('Ctrl Pts',(-13.6839307875775,-2.32072459453129,
12.4159313107788));
#34472=CARTESIAN_POINT('Ctrl Pts',(-52.4024685456813,0.42091842584111,1.07848752259329));
#34473=CARTESIAN_POINT('Ctrl Pts',(-52.1802375771876,0.412015546281074,
1.41623609520554));
#34474=CARTESIAN_POINT('Ctrl Pts',(-51.9507383304312,0.403442573942463,
1.75103341927263));
#34475=CARTESIAN_POINT('Ctrl Pts',(-50.9433065549328,0.368526239150617,
3.16205940115231));
#34476=CARTESIAN_POINT('Ctrl Pts',(-49.288458491273,0.324281374370589,5.1968918518957));
#34477=CARTESIAN_POINT('Ctrl Pts',(-46.5068266086684,0.279215865745994,
7.86614365370726));
#34478=CARTESIAN_POINT('Ctrl Pts',(-42.9606237061091,0.243759038204317,
10.5205566320174));
#34479=CARTESIAN_POINT('Ctrl Pts',(-39.0986741979798,0.21967725703067,12.5843645499658));
#34480=CARTESIAN_POINT('Ctrl Pts',(-35.011880788994,0.192114722189047,14.0340846219934));
#34481=CARTESIAN_POINT('Ctrl Pts',(-30.7937738910368,0.154437491851918,
14.980275523655));
#34482=CARTESIAN_POINT('Ctrl Pts',(-26.4722529890479,0.0954817696064694,
15.2818750597512));
#34483=CARTESIAN_POINT('Ctrl Pts',(-22.1384049721548,0.0048363712043943,
14.9165437766969));
#34484=CARTESIAN_POINT('Ctrl Pts',(-18.4568160996774,-0.0979118428630517,
14.1360163938409));
#34485=CARTESIAN_POINT('Ctrl Pts',(-16.0521989825758,-0.184631554593919,
13.2973974695823));
#34486=CARTESIAN_POINT('Ctrl Pts',(-14.4937852736123,-0.247909792323189,
12.6380015081389));
#34487=CARTESIAN_POINT('Ctrl Pts',(-14.1228765604169,-0.263520166061751,
12.4720559824965));
#34488=CARTESIAN_POINT('Ctrl Pts',(-13.75662704767,-0.279478515480188,12.2992216174618));
#34489=CARTESIAN_POINT('Ctrl Pts',(-51.6812106838394,3.93922736422659,-1.9401699282817));
#34490=CARTESIAN_POINT('Ctrl Pts',(-51.4760538436571,3.92273017306588,-1.59057825251053));
#34491=CARTESIAN_POINT('Ctrl Pts',(-51.263584894514,3.90651491483579,-1.24347554024485));
#34492=CARTESIAN_POINT('Ctrl Pts',(-50.3283655357373,3.83888692720806,0.221910991507739));
#34493=CARTESIAN_POINT('Ctrl Pts',(-48.7801103103006,3.74496038387833,2.34729155538723));
#34494=CARTESIAN_POINT('Ctrl Pts',(-46.1450033475284,3.6271896762232,5.17349042592491));
#34495=CARTESIAN_POINT('Ctrl Pts',(-42.7521630054787,3.50969140214063,8.03442807426281));
#34496=CARTESIAN_POINT('Ctrl Pts',(-39.0191042094579,3.40771510315772,10.3324686633491));
#34497=CARTESIAN_POINT('Ctrl Pts',(-35.0329941213862,3.30695483103527,12.0417080640687));
#34498=CARTESIAN_POINT('Ctrl Pts',(-30.891020829036,3.1998573133211,13.2663261001275));
#34499=CARTESIAN_POINT('Ctrl Pts',(-26.6124740089013,3.07607789704229,13.8683245393028));
#34500=CARTESIAN_POINT('Ctrl Pts',(-22.2847669139082,2.92448144596071,13.8228473589188));
#34501=CARTESIAN_POINT('Ctrl Pts',(-18.5815246338201,2.77158317941627,13.3286701208219));
#34502=CARTESIAN_POINT('Ctrl Pts',(-16.1434293986355,2.65236568914073,12.6883132843688));
#34503=CARTESIAN_POINT('Ctrl Pts',(-14.5563351006402,2.56779645721963,12.1616854590491));
#34504=CARTESIAN_POINT('Ctrl Pts',(-14.1776469180455,2.54707902977605,12.0275353341212));
#34505=CARTESIAN_POINT('Ctrl Pts',(-13.8027662533503,2.52604544176493,11.8862838166198));
#34506=CARTESIAN_POINT('Ctrl Pts',(-50.7849974013264,7.64857049485316,-5.70122737713707));
#34507=CARTESIAN_POINT('Ctrl Pts',(-50.5995059831301,7.62538079009264,-5.33758143700541));
#34508=CARTESIAN_POINT('Ctrl Pts',(-50.4066643269634,7.6024320797305,-4.97591736065702));
#34509=CARTESIAN_POINT('Ctrl Pts',(-49.5547312908686,7.50598047950645,-3.44637468117887));
#34510=CARTESIAN_POINT('Ctrl Pts',(-48.1294152598895,7.36825978906471,-1.21450705382876));
#34511=CARTESIAN_POINT('Ctrl Pts',(-45.6633104617947,7.18657585481396,1.79524361104216));
#34512=CARTESIAN_POINT('Ctrl Pts',(-42.4473772579401,6.99739878870591,4.89670142836206));
#34513=CARTESIAN_POINT('Ctrl Pts',(-38.8630354862451,6.82819742189185,7.46642848002267));
#34514=CARTESIAN_POINT('Ctrl Pts',(-34.993164758737,6.66543158101024,9.47573998110103));
#34515=CARTESIAN_POINT('Ctrl Pts',(-30.9391726596963,6.50060855796851,11.0216245495761));
#34516=CARTESIAN_POINT('Ctrl Pts',(-26.7104480931522,6.32441606849526,11.9694786820947));
#34517=CARTESIAN_POINT('Ctrl Pts',(-22.3901917930574,6.12505774886043,12.2915705314655));
#34518=CARTESIAN_POINT('Ctrl Pts',(-18.662378603183,5.93384517916791,12.1260283153189));
#34519=CARTESIAN_POINT('Ctrl Pts',(-16.1860069271246,5.79035915091665,11.7129412555412));
#34520=CARTESIAN_POINT('Ctrl Pts',(-14.5660799894216,5.69001969995687,11.3384237535995));
#34521=CARTESIAN_POINT('Ctrl Pts',(-14.1785181216796,5.66551509710643,11.2407915689695));
#34522=CARTESIAN_POINT('Ctrl Pts',(-13.7938169458334,5.64071489355821,11.1359032947783));
#34523=CARTESIAN_POINT('Ctrl Pts',(-49.9421179311135,10.6050661536892,-9.24468742082597));
#34524=CARTESIAN_POINT('Ctrl Pts',(-49.7739435279274,10.5777689837161,-8.86839695461952));
#34525=CARTESIAN_POINT('Ctrl Pts',(-49.5983941291953,10.5506896266998,-8.49366788478655));
#34526=CARTESIAN_POINT('Ctrl Pts',(-48.8198852019977,10.4365567481294,-6.90671046826663));
#34527=CARTESIAN_POINT('Ctrl Pts',(-47.5029498445623,10.2719415070743,-4.57979182054436));
#34528=CARTESIAN_POINT('Ctrl Pts',(-45.1858329874651,10.0511774947007,-1.40687928349953));
#34529=CARTESIAN_POINT('Ctrl Pts',(-42.1258585913662,9.81863871620139,1.90769663539571));
#34530=CARTESIAN_POINT('Ctrl Pts',(-38.6726313940744,9.60967367489776,4.71739998166952));
#34531=CARTESIAN_POINT('Ctrl Pts',(-34.9052599503476,9.41153176383594,6.99109418128465));
#34532=CARTESIAN_POINT('Ctrl Pts',(-30.9288736511082,9.21500541081661,8.81955439844158));
#34533=CARTESIAN_POINT('Ctrl Pts',(-26.7441444079205,9.01175979868378,10.07105129362));
#34534=CARTESIAN_POINT('Ctrl Pts',(-22.4305703275812,8.78956564702969,10.7153281176886));
#34535=CARTESIAN_POINT('Ctrl Pts',(-18.6812269030208,8.58124477590158,10.8375076202336));
#34536=CARTESIAN_POINT('Ctrl Pts',(-16.1712252072741,8.42762540105217,10.6231810669046));
#34537=CARTESIAN_POINT('Ctrl Pts',(-14.5224388077575,8.32086564673385,10.3816244231577));
#34538=CARTESIAN_POINT('Ctrl Pts',(-14.1271306078084,8.29482075310626,10.3159831567471));
#34539=CARTESIAN_POINT('Ctrl Pts',(-13.7339007596026,8.26849188852043,10.2430203848967));
#34540=CARTESIAN_POINT('Ctrl Pts',(-48.9190413835945,13.6252616883324,-13.5486550301516));
#34541=CARTESIAN_POINT('Ctrl Pts',(-48.7707426344082,13.5952855444977,-13.157707499603));
#34542=CARTESIAN_POINT('Ctrl Pts',(-48.6150473980909,13.5655149131873,-12.7678728818138));
#34543=CARTESIAN_POINT('Ctrl Pts',(-47.9208800025026,13.4398628522405,-11.1146965665455));
#34544=CARTESIAN_POINT('Ctrl Pts',(-46.728437940084,13.2576618204372,-8.67830331115292));
#34545=CARTESIAN_POINT('Ctrl Pts',(-44.5824461493721,13.0115743729063,-5.31790493889871));
#34546=CARTESIAN_POINT('Ctrl Pts',(-41.7015829857729,12.751644575675,-1.75889877066355));
#34547=CARTESIAN_POINT('Ctrl Pts',(-38.3989009034041,12.5189796899122,1.32550695910777));
#34548=CARTESIAN_POINT('Ctrl Pts',(-34.7491709788807,12.301865256328,3.90134067434971));
#34549=CARTESIAN_POINT('Ctrl Pts',(-30.8618018689639,12.0904144587841,6.05235254691278));
#34550=CARTESIAN_POINT('Ctrl Pts',(-26.7274417568102,11.8774764455751,7.64998503667857));
#34551=CARTESIAN_POINT('Ctrl Pts',(-22.4213311430581,11.6504923923572,8.66107165744092));
#34552=CARTESIAN_POINT('Ctrl Pts',(-18.6470419033825,11.4410171343385,9.1105101988073));
#34553=CARTESIAN_POINT('Ctrl Pts',(-16.09824451068,11.2882220371981,9.12204563341117));
#34554=CARTESIAN_POINT('Ctrl Pts',(-14.4161911759617,11.1823584691134,9.03150892265254));
#34555=CARTESIAN_POINT('Ctrl Pts',(-14.0120429911226,11.1565388193505,9.00226487804507));
#34556=CARTESIAN_POINT('Ctrl Pts',(-13.6091566427535,11.1304479812224,8.96568686170588));
#34557=CARTESIAN_POINT('Ctrl Pts',(-47.9760265763764,15.9398275064074,-17.5159409401114));
#34558=CARTESIAN_POINT('Ctrl Pts',(-47.845173721344,15.9092719019138,-17.1120993990557));
#34559=CARTESIAN_POINT('Ctrl Pts',(-47.7069077842713,15.8789225535602,-16.7090082004271));
#34560=CARTESIAN_POINT('Ctrl Pts',(-47.0867986772895,15.7507918597713,-14.9978536657822));
#34561=CARTESIAN_POINT('Ctrl Pts',(-46.0036684189674,15.5646999212503,-12.4656708226873));
#34562=CARTESIAN_POINT('Ctrl Pts',(-44.0079170280876,15.3133344724918,-8.94141691639378));
#34563=CARTESIAN_POINT('Ctrl Pts',(-41.28427599618,15.0487502016962,-5.16901063122818));
#34564=CARTESIAN_POINT('Ctrl Pts',(-38.1136889032606,14.8142492774957,-1.84505503058845));
#34565=CARTESIAN_POINT('Ctrl Pts',(-34.5671043809285,14.5991383033468,0.993962480657613));
#34566=CARTESIAN_POINT('Ctrl Pts',(-30.7576929966717,14.3930646018661,3.42570304001716));
#34567=CARTESIAN_POINT('Ctrl Pts',(-26.6672790166255,14.1899609567462,5.32428496179455));
#34568=CARTESIAN_POINT('Ctrl Pts',(-22.3673509929844,13.977122935371,6.65396667590596));
#34569=CARTESIAN_POINT('Ctrl Pts',(-18.5707723340629,13.7824369346935,7.38741364551115));
#34570=CARTESIAN_POINT('Ctrl Pts',(-15.9876039554074,13.6409944051188,7.5947963714473));
#34571=CARTESIAN_POINT('Ctrl Pts',(-14.276121320492,13.5429643472183,7.63515342013838));
#34572=CARTESIAN_POINT('Ctrl Pts',(-13.8642441857383,13.5190447294408,7.63748833309744));
#34573=CARTESIAN_POINT('Ctrl Pts',(-13.4529946868638,13.4948677704672,7.63251220583618));
#34574=CARTESIAN_POINT('Ctrl Pts',(-46.8518840273662,18.188947172369,-22.2413015794463));
#34575=CARTESIAN_POINT('Ctrl Pts',(-46.7409936449756,18.1597316481657,-21.8228367447842));
#34576=CARTESIAN_POINT('Ctrl Pts',(-46.6226695035064,18.1307342364494,-21.4047437320774));
#34577=CARTESIAN_POINT('Ctrl Pts',(-46.0872954411095,18.0083786966032,-19.6281175320506));
#34578=CARTESIAN_POINT('Ctrl Pts',(-45.129232033727,17.830846834045,-16.9877153100835));
#34579=CARTESIAN_POINT('Ctrl Pts',(-43.3053469438411,17.5925027676131,-13.2782512104459));
#34580=CARTESIAN_POINT('Ctrl Pts',(-40.7615054946399,17.3443426911773,-9.26458661207112));
#34581=CARTESIAN_POINT('Ctrl Pts',(-37.7418859285627,17.1289494695207,-5.66981412176888));
#34582=CARTESIAN_POINT('Ctrl Pts',(-34.3130328703258,16.9369213116231,-2.53334672084906));
#34583=CARTESIAN_POINT('Ctrl Pts',(-30.5924274640541,16.7575317657622,0.215568117021719));
#34584=CARTESIAN_POINT('Ctrl Pts',(-26.5517507933222,16.5859876106103,2.45399400638956));
#34585=CARTESIAN_POINT('Ctrl Pts',(-22.2581672791192,16.4095763329362,4.14320050884528));
#34586=CARTESIAN_POINT('Ctrl Pts',(-18.4353192402588,16.2491906636996,5.19694543642052));
#34587=CARTESIAN_POINT('Ctrl Pts',(-15.8122098215815,16.1323920433636,5.62504820870853));
#34588=CARTESIAN_POINT('Ctrl Pts',(-14.0666127972462,16.0510402241362,5.81286568186864));
#34589=CARTESIAN_POINT('Ctrl Pts',(-13.6458884937628,16.0311583490605,5.85078659563688));
#34590=CARTESIAN_POINT('Ctrl Pts',(-13.2251660207337,16.01103806515,5.8814349310918));
#34591=CARTESIAN_POINT('Ctrl Pts',(-45.8324093010083,19.7983627848149,-26.5208862143558));
#34592=CARTESIAN_POINT('Ctrl Pts',(-45.7389874917903,19.7720645135703,-26.0898395604211));
#34593=CARTESIAN_POINT('Ctrl Pts',(-45.6381086468713,19.7460021313493,-25.6588639245312));
#34594=CARTESIAN_POINT('Ctrl Pts',(-45.1768456950506,19.6361820466171,-23.8261216909706));
#34595=CARTESIAN_POINT('Ctrl Pts',(-44.3281644612076,19.4774394485581,-21.0928503619399));
#34596=CARTESIAN_POINT('Ctrl Pts',(-42.6545622359201,19.2670183310104,-17.2241812601364));
#34597=CARTESIAN_POINT('Ctrl Pts',(-40.2678831350707,19.0520629838802,-13.0029153733495));
#34598=CARTESIAN_POINT('Ctrl Pts',(-37.3801185452477,18.8717166252608,-9.17492625949768));
#34599=CARTESIAN_POINT('Ctrl Pts',(-34.0539261447635,18.7178122962125,-5.78223641699785));
#34600=CARTESIAN_POINT('Ctrl Pts',(-30.4105634338668,18.5794411422907,-2.76010396718932));
#34601=CARTESIAN_POINT('Ctrl Pts',(-26.4127865038372,18.4529446490623,-0.228985441518097));
#34602=CARTESIAN_POINT('Ctrl Pts',(-22.1239414086001,18.3257380682571,1.76972639038569));
#34603=CARTESIAN_POINT('Ctrl Pts',(-18.2772624864382,18.2102139945187,3.09907703011229));
#34604=CARTESIAN_POINT('Ctrl Pts',(-15.6185315114537,18.1249152482566,3.71699064283981));
#34605=CARTESIAN_POINT('Ctrl Pts',(-13.8426013038607,18.064727637235,4.03157365432944));
#34606=CARTESIAN_POINT('Ctrl Pts',(-13.4141050388812,18.0499634327475,4.10007468068017));
#34607=CARTESIAN_POINT('Ctrl Pts',(-12.98514701221,18.0349776243875,4.16132700560662));
#34608=CARTESIAN_POINT('Ctrl Pts',(-45.0842283862103,20.6836496418694,-29.6550287755562));
#34609=CARTESIAN_POINT('Ctrl Pts',(-45.003258058161,20.6606519170286,-29.2152696874927));
#34610=CARTESIAN_POINT('Ctrl Pts',(-44.9148096467711,20.6379063239872,-28.7753846724798));
#34611=CARTESIAN_POINT('Ctrl Pts',(-44.5063377455988,20.5422448076096,-26.9038829192087));
#34612=CARTESIAN_POINT('Ctrl Pts',(-43.7355687870834,20.4047755971079,-24.1063107670654));
#34613=CARTESIAN_POINT('Ctrl Pts',(-42.1689863802376,20.225761668211,-20.1270266003951));
#34614=CARTESIAN_POINT('Ctrl Pts',(-39.8941747111083,20.0475517349526,-15.7611783203895));
#34615=CARTESIAN_POINT('Ctrl Pts',(-37.1001683740488,19.9048724048602,-11.7704442775268));
#34616=CARTESIAN_POINT('Ctrl Pts',(-33.8468226781346,19.790507905872,-8.19875157949892));
#34617=CARTESIAN_POINT('Ctrl Pts',(-30.2580901286986,19.6935273080542,-4.98563776740868));
#34618=CARTESIAN_POINT('Ctrl Pts',(-26.2903187546283,19.6110850660289,-2.24985464000988));
#34619=CARTESIAN_POINT('Ctrl Pts',(-22.004099523508,19.530779076001,-0.0347369010676612));
#34620=CARTESIAN_POINT('Ctrl Pts',(-18.1396517532032,19.4573327991495,1.48727002286964));
#34621=CARTESIAN_POINT('Ctrl Pts',(-15.4549058300219,19.4012238336331,2.23781143845789));
#34622=CARTESIAN_POINT('Ctrl Pts',(-13.6569059350236,19.3605693891818,2.64094405458518));
#34623=CARTESIAN_POINT('Ctrl Pts',(-13.2228097538454,19.3505226070412,2.73078956348044));
#34624=CARTESIAN_POINT('Ctrl Pts',(-12.7879686848707,19.3402634731691,2.81338796599552));
#34625=CARTESIAN_POINT('Ctrl Pts',(-44.662892732026,21.117312799858,-31.4181748325572));
#34626=CARTESIAN_POINT('Ctrl Pts',(-44.5888652243124,21.0964267127388,-30.9736279625641));
#34627=CARTESIAN_POINT('Ctrl Pts',(-44.5073458457706,21.0758020890032,-30.5288506865157));
#34628=CARTESIAN_POINT('Ctrl Pts',(-44.1282930941642,20.9891913310095,-28.6360818457722));
#34629=CARTESIAN_POINT('Ctrl Pts',(-43.4009419459597,20.8653273744228,-25.8031807347521));
#34630=CARTESIAN_POINT('Ctrl Pts',(-41.89399142233,20.7063681300896,-21.7630023216518));
#34631=CARTESIAN_POINT('Ctrl Pts',(-39.6814995550379,20.5515335415639,-17.3174532750829));
#34632=CARTESIAN_POINT('Ctrl Pts',(-36.9397000222138,20.4326519806542,-13.2369023278833));
#34633=CARTESIAN_POINT('Ctrl Pts',(-33.7268776305302,20.3430531321453,-9.56634965008858));
#34634=CARTESIAN_POINT('Ctrl Pts',(-30.1684879882071,20.2718184169426,-6.2477203062325));
#34635=CARTESIAN_POINT('Ctrl Pts',(-26.2172948692171,20.2165549432469,-3.39882871550882));
#34636=CARTESIAN_POINT('Ctrl Pts',(-21.9323446710577,20.164982094833,-1.06410354139334));
#34637=CARTESIAN_POINT('Ctrl Pts',(-18.0577887965766,20.117197691553,0.564381352586137));
#34638=CARTESIAN_POINT('Ctrl Pts',(-15.3583788882933,20.0788282397779,1.3882155360768));
#34639=CARTESIAN_POINT('Ctrl Pts',(-13.5479598507639,20.0500302875854,1.84027756187001));
#34640=CARTESIAN_POINT('Ctrl Pts',(-13.1107276962677,20.0428451797642,1.9419101019128));
#34641=CARTESIAN_POINT('Ctrl Pts',(-12.6726064287586,20.0354515632684,2.03628977646432));
#34642=CARTESIAN_POINT('Ctrl Pts',(-44.5430178615257,21.2334813897109,-31.9196050263226));
#34643=CARTESIAN_POINT('Ctrl Pts',(-44.4709595266528,21.2132228077857,-31.4737036812526));
#34644=CARTESIAN_POINT('Ctrl Pts',(-44.3914050023503,21.1932283095702,-31.0275427813411));
#34645=CARTESIAN_POINT('Ctrl Pts',(-44.0206929537339,21.1093059289188,-29.1287610721839));
#34646=CARTESIAN_POINT('Ctrl Pts',(-43.3056498664664,20.9894835119608,-26.2858714770087));
#34647=CARTESIAN_POINT('Ctrl Pts',(-41.8155996100812,20.8364792943525,-22.2284811708669));
#34648=CARTESIAN_POINT('Ctrl Pts',(-39.6207640549177,20.6885792302246,-17.7604142055847));
#34649=CARTESIAN_POINT('Ctrl Pts',(-36.893748873692,20.5767478260626,-13.65450541157));
#34650=CARTESIAN_POINT('Ctrl Pts',(-33.6923948010559,20.4944756050622,-9.95606573502258));
#34651=CARTESIAN_POINT('Ctrl Pts',(-30.1425849867683,20.4308554028779,-6.60769833039274));
#34652=CARTESIAN_POINT('Ctrl Pts',(-26.1960663524986,20.3836340081555,-3.72696185433125));
#34653=CARTESIAN_POINT('Ctrl Pts',(-21.9114441822608,20.340580727313,-1.35859572870376));
#34654=CARTESIAN_POINT('Ctrl Pts',(-18.0339852147836,20.3004356869138,0.29981387071413));
#34655=CARTESIAN_POINT('Ctrl Pts',(-15.3303820039488,20.2673681898868,1.1442388647251));
#34656=CARTESIAN_POINT('Ctrl Pts',(-13.5164122338016,20.2421246596599,1.61004653123375));
#34657=CARTESIAN_POINT('Ctrl Pts',(-13.0782862790771,20.2357981340653,1.71498902850875));
#34658=CARTESIAN_POINT('Ctrl Pts',(-12.6392326905351,20.2292648564311,1.81267574713249));
#34659=CARTESIAN_POINT('Ctrl Pts',(-44.4227536970802,21.3428689572265,-32.4224779048909));
#34660=CARTESIAN_POINT('Ctrl Pts',(-44.3526640269045,21.323266505305,-31.9752258099344));
#34661=CARTESIAN_POINT('Ctrl Pts',(-44.2750736219715,21.303930781031,-31.527685218234));
#34662=CARTESIAN_POINT('Ctrl Pts',(-43.9126982425839,21.2228186866547,-29.622908370639));
#34663=CARTESIAN_POINT('Ctrl Pts',(-43.2099559547992,21.1072213437662,-26.7700597812476));
#34664=CARTESIAN_POINT('Ctrl Pts',(-41.7367921725809,20.9604400919523,-22.695512686503));
#34665=CARTESIAN_POINT('Ctrl Pts',(-39.559593085345,20.819779963638,-18.2050092760581));
#34666=CARTESIAN_POINT('Ctrl Pts',(-36.8473391964997,20.7152993064879,-14.0738520907221));
#34667=CARTESIAN_POINT('Ctrl Pts',(-33.6574284865114,20.6406553883908,-10.3476693174035));
#34668=CARTESIAN_POINT('Ctrl Pts',(-30.116172752319,20.5849601975755,-6.9697435065069));
#34669=CARTESIAN_POINT('Ctrl Pts',(-26.1743020658466,20.5461109852346,-4.05738761544544));
#34670=CARTESIAN_POINT('Ctrl Pts',(-21.8899779235893,20.5119420676311,-1.65565290050457));
#34671=CARTESIAN_POINT('Ctrl Pts',(-18.0095823216269,20.4797911688045,0.0324145407608299));
#34672=CARTESIAN_POINT('Ctrl Pts',(-15.3017542572766,20.4522911786996,0.897238235717693));
#34673=CARTESIAN_POINT('Ctrl Pts',(-13.4842075697677,20.4307901345004,1.37666218058237));
#34674=CARTESIAN_POINT('Ctrl Pts',(-13.045183204915,20.4253683033402,1.48488253420603));
#34675=CARTESIAN_POINT('Ctrl Pts',(-12.6051943113167,20.4197421663948,1.58584330107463));
#34676=CARTESIAN_POINT('',(-41.8448486400327,20.5529756002067,-21.125185596459));
#34677=CARTESIAN_POINT('Ctrl Pts',(-45.5574402514582,-3.27137127985419,
11.0356091047656));
#34678=CARTESIAN_POINT('Ctrl Pts',(-46.5282583031688,1.76302065360852,7.02785488001061));
#34679=CARTESIAN_POINT('Ctrl Pts',(-47.208951015116,6.26298702224666,1.80001364845749));
#34680=CARTESIAN_POINT('Ctrl Pts',(-46.4493663072616,12.5188402724798,-6.92582206775948));
#34681=CARTESIAN_POINT('Ctrl Pts',(-45.9228610941799,14.4577038717082,-9.88449847911477));
#34682=CARTESIAN_POINT('Ctrl Pts',(-44.3011001623703,17.848637426394,-15.5857057966297));
#34683=CARTESIAN_POINT('Ctrl Pts',(-43.226555471649,19.3555632898771,-18.3882954426068));
#34684=CARTESIAN_POINT('Ctrl Pts',(-41.8448486400325,20.5529756002057,-21.1251855964593));
#34685=CARTESIAN_POINT('Ctrl Pts',(-20.6391955918159,19.9464420456703,-0.223416847360507));
#34686=CARTESIAN_POINT('Ctrl Pts',(-25.3016667625211,20.0189549105364,-2.24188131992115));
#34687=CARTESIAN_POINT('Ctrl Pts',(-29.5639710976893,20.0954766247834,-5.1557195977613));
#34688=CARTESIAN_POINT('Ctrl Pts',(-36.794002124349,20.2752040736289,-12.2855823812624));
#34689=CARTESIAN_POINT('Ctrl Pts',(-39.7632550653996,20.3824974081049,-16.5004134660379));
#34690=CARTESIAN_POINT('Ctrl Pts',(-41.8448486400326,20.5529756002056,-21.1251855964591));
#34691=CARTESIAN_POINT('Ctrl Pts',(-44.6192557971265,20.9435908393615,-30.0463497312518));
#34692=CARTESIAN_POINT('Ctrl Pts',(-44.5900546737109,20.9358615047579,-29.8937793939917));
#34693=CARTESIAN_POINT('Ctrl Pts',(-44.5608535502954,20.9281321701544,-29.7412090567315));
#34694=CARTESIAN_POINT('Ctrl Pts',(-44.5316524268797,20.9204028355509,-29.5886387194714));
#34695=CARTESIAN_POINT('Ctrl Pts',(-41.6115400853208,20.1474693751975,-14.3316049934558));
#34696=CARTESIAN_POINT('Ctrl Pts',(-29.138210899356,20.0812550388979,-1.52559743671482));
#34697=CARTESIAN_POINT('Ctrl Pts',(-14.0127168543002,19.8399463130827,1.960201331136));
#34698=CARTESIAN_POINT('Ctrl Pts',(-44.6192837493325,20.9469886892296,-30.0462588269131));
#34699=CARTESIAN_POINT('Ctrl Pts',(-44.5900898599601,20.9392720585054,-29.8936849146578));
#34700=CARTESIAN_POINT('Ctrl Pts',(-44.5608959705877,20.9315554277811,-29.7411110024025));
#34701=CARTESIAN_POINT('Ctrl Pts',(-44.5317020812152,20.9238387970569,-29.5885370901472));
#34702=CARTESIAN_POINT('Ctrl Pts',(-41.6123131439728,20.1521757246323,-14.331145864618));
#34703=CARTESIAN_POINT('Ctrl Pts',(-29.1385639877428,20.0873688943554,-1.52532137413304));
#34704=CARTESIAN_POINT('Ctrl Pts',(-14.0131984274678,19.8474084919615,1.96069388785016));
#34705=CARTESIAN_POINT('Ctrl Pts',(-44.6193117015385,20.9503865390978,-30.0461679225743));
#34706=CARTESIAN_POINT('Ctrl Pts',(-44.5901250462092,20.9426826122528,-29.8935904353239));
#34707=CARTESIAN_POINT('Ctrl Pts',(-44.56093839088,20.9349786854078,-29.7410129480734));
#34708=CARTESIAN_POINT('Ctrl Pts',(-44.5317517355507,20.9272747585629,-29.588435460823));
#34709=CARTESIAN_POINT('Ctrl Pts',(-41.6130862026247,20.1568820740671,-14.3306867357802));
#34710=CARTESIAN_POINT('Ctrl Pts',(-29.1389170761296,20.093482749813,-1.52504531155125));
#34711=CARTESIAN_POINT('Ctrl Pts',(-14.0136800006353,19.8548706708402,1.96118644456431));
#34712=CARTESIAN_POINT('Ctrl Pts',(-44.6193396537445,20.9537843889659,-30.0460770182355));
#34713=CARTESIAN_POINT('Ctrl Pts',(-44.5901602324584,20.9460931660003,-29.8934959559899));
#34714=CARTESIAN_POINT('Ctrl Pts',(-44.5609808111723,20.9384019430346,-29.7409148937444));
#34715=CARTESIAN_POINT('Ctrl Pts',(-44.5318013898862,20.9307107200689,-29.5883338314988));
#34716=CARTESIAN_POINT('Ctrl Pts',(-41.6138592612767,20.1615884235019,-14.3302276069424));
#34717=CARTESIAN_POINT('Ctrl Pts',(-29.1392701645165,20.0995966052706,-1.52476924896946));
#34718=CARTESIAN_POINT('Ctrl Pts',(-14.0141615738029,19.862332849719,1.96167900127847));
#34719=CARTESIAN_POINT('Ctrl Pts',(-44.6194245372235,20.9641027630587,-30.0458009657286));
#34720=CARTESIAN_POINT('Ctrl Pts',(-44.590267083819,20.9564501184246,-29.8932090471655));
#34721=CARTESIAN_POINT('Ctrl Pts',(-44.5611096304145,20.9487974737906,-29.7406171286024));
#34722=CARTESIAN_POINT('Ctrl Pts',(-44.53195217701,20.9411448291565,-29.5880252100392));
#34723=CARTESIAN_POINT('Ctrl Pts',(-41.61620683656,20.1758803657488,-14.3288333537267));
#34724=CARTESIAN_POINT('Ctrl Pts',(-29.1403424008437,20.1181627721728,-1.52393091970171));
#34725=CARTESIAN_POINT('Ctrl Pts',(-14.0156239845298,19.8849935193208,1.96317476614031));
#34726=CARTESIAN_POINT('Ctrl Pts',(-44.6195943039941,20.9847395112521,-30.0452488605024));
#34727=CARTESIAN_POINT('Ctrl Pts',(-44.5904807864153,20.9771640232786,-29.892635229375));
#34728=CARTESIAN_POINT('Ctrl Pts',(-44.5613672688365,20.9695885353052,-29.7400215982477));
#34729=CARTESIAN_POINT('Ctrl Pts',(-44.5322537512578,20.9620130473318,-29.5874079671203));
#34730=CARTESIAN_POINT('Ctrl Pts',(-41.6209019933817,20.2044642499886,-14.326044854383));
#34731=CARTESIAN_POINT('Ctrl Pts',(-29.142486871632,20.1552951062578,-1.52225425630454));
#34732=CARTESIAN_POINT('Ctrl Pts',(-14.0185488059837,19.9303148585245,1.96616629586402));
#34733=CARTESIAN_POINT('Ctrl Pts',(-44.6198489420188,21.0156946339229,-30.0444206880632));
#34734=CARTESIAN_POINT('Ctrl Pts',(-44.5908013322223,21.0082348808134,-29.891774492956));
#34735=CARTESIAN_POINT('Ctrl Pts',(-44.5617537224258,21.000775127704,-29.7391282978488));
#34736=CARTESIAN_POINT('Ctrl Pts',(-44.5327061126293,20.9933153745945,-29.5864821027416));
#34737=CARTESIAN_POINT('Ctrl Pts',(-41.6279451329777,20.2473400636495,-14.3218625920227));
#34738=CARTESIAN_POINT('Ctrl Pts',(-29.1457034681185,20.2109936225946,-1.51973895748648));
#34739=CARTESIAN_POINT('Ctrl Pts',(-14.0229360381646,19.9982968673298,1.97065359044955));
#34740=CARTESIAN_POINT('Ctrl Pts',(-44.6201035640659,21.0466497571015,-30.0435924964379));
#34741=CARTESIAN_POINT('Ctrl Pts',(-44.5911218673776,21.0393057386868,-29.8909137437463));
#34742=CARTESIAN_POINT('Ctrl Pts',(-44.5621401706893,21.0319617202721,-29.7382349910547));
#34743=CARTESIAN_POINT('Ctrl Pts',(-44.5331584740009,21.0246177018574,-29.5855562383631));
#34744=CARTESIAN_POINT('Ctrl Pts',(-41.6349888051667,20.2902158603888,-14.317680969202));
#34745=CARTESIAN_POINT('Ctrl Pts',(-29.1489199175254,20.2666921589687,-1.51722325780471));
#34746=CARTESIAN_POINT('Ctrl Pts',(-14.0273232703454,20.0662788761352,1.97514088503509));
#34747=CARTESIAN_POINT('Ctrl Pts',(-44.6202733040188,21.0672865061488,-30.0430403590245));
#34748=CARTESIAN_POINT('Ctrl Pts',(-44.5913355520954,21.0600196441101,-29.8903399044977));
#34749=CARTESIAN_POINT('Ctrl Pts',(-44.562397800172,21.0527527820714,-29.7376394499708));
#34750=CARTESIAN_POINT('Ctrl Pts',(-44.5334600482486,21.0454859200326,-29.584938995444));
#34751=CARTESIAN_POINT('Ctrl Pts',(-41.6396848559067,20.3187997161584,-14.3148935427609));
#34752=CARTESIAN_POINT('Ctrl Pts',(-29.151064141164,20.3038245267329,-1.5155459213784));
#34753=CARTESIAN_POINT('Ctrl Pts',(-14.0302480917993,20.1116002153389,1.97813241475879));
#34754=CARTESIAN_POINT('Ctrl Pts',(-44.6203581739018,21.0776048806767,-30.0427642902148));
#34755=CARTESIAN_POINT('Ctrl Pts',(-44.591442394392,21.0703765968246,-29.8900529848047));
#34756=CARTESIAN_POINT('Ctrl Pts',(-44.5625266148822,21.0631483129724,-29.7373416793946));
#34757=CARTESIAN_POINT('Ctrl Pts',(-44.5336108353724,21.0559200291202,-29.5846303739845));
#34758=CARTESIAN_POINT('Ctrl Pts',(-41.6420328843933,20.3330916439037,-14.3134998329725));
#34759=CARTESIAN_POINT('Ctrl Pts',(-29.1521362519135,20.3223907107576,-1.51470725069692));
#34760=CARTESIAN_POINT('Ctrl Pts',(-14.0317105025263,20.1342608849406,1.97962817962064));
#34761=CARTESIAN_POINT('Ctrl Pts',(-44.6203663519816,21.0785991614118,-30.0427376881664));
#34762=CARTESIAN_POINT('Ctrl Pts',(-44.5914526897381,21.0713745949617,-29.8900253371629));
#34763=CARTESIAN_POINT('Ctrl Pts',(-44.5625390274948,21.0641500285117,-29.7373129861594));
#34764=CARTESIAN_POINT('Ctrl Pts',(-44.5336253652514,21.0569254620617,-29.5846006351559));
#34765=CARTESIAN_POINT('Ctrl Pts',(-41.6422591409111,20.3344688170607,-14.3133655348048));
#34766=CARTESIAN_POINT('Ctrl Pts',(-29.1522395607303,20.3241797521467,-1.51462643621404));
#34767=CARTESIAN_POINT('Ctrl Pts',(-14.0318514207308,20.1364444718193,1.97977231183664));
#34768=CARTESIAN_POINT('Ctrl Pts',(-44.6203745300613,21.0795934421468,-30.042711086118));
#34769=CARTESIAN_POINT('Ctrl Pts',(-44.5914629850843,21.0723725930989,-29.8899976895211));
#34770=CARTESIAN_POINT('Ctrl Pts',(-44.5625514401073,21.0651517440511,-29.7372842929242));
#34771=CARTESIAN_POINT('Ctrl Pts',(-44.5336398951302,21.0579308950032,-29.5845708963273));
#34772=CARTESIAN_POINT('Ctrl Pts',(-41.6424853974288,20.3358459902176,-14.3132312366371));
#34773=CARTESIAN_POINT('Ctrl Pts',(-29.1523428695472,20.3259687935359,-1.51454562173116));
#34774=CARTESIAN_POINT('Ctrl Pts',(-14.0319923389354,20.1386280586979,1.97991644405265));
#34775=CARTESIAN_POINT('Ctrl Pts',(-44.620382708141,21.0805877228818,-30.0426844840695));
#34776=CARTESIAN_POINT('Ctrl Pts',(-44.5914732804304,21.0733705912361,-29.8899700418792));
#34777=CARTESIAN_POINT('Ctrl Pts',(-44.5625638527198,21.0661534595904,-29.7372555996889));
#34778=CARTESIAN_POINT('Ctrl Pts',(-44.5336544250092,21.0589363279447,-29.5845411574986));
#34779=CARTESIAN_POINT('Ctrl Pts',(-41.6427116539466,20.3372231633746,-14.3130969384694));
#34780=CARTESIAN_POINT('Ctrl Pts',(-29.152446178364,20.327757834925,-1.51446480724828));
#34781=CARTESIAN_POINT('Ctrl Pts',(-14.03213325714,20.1408116455766,1.98006057626865));
#34782=CARTESIAN_POINT('',(-41.8448486400327,20.5529756002067,-21.125185596459));
#34783=CARTESIAN_POINT('Ctrl Pts',(-2.30431969428901,21.2883239772394,-54.9614594276758));
#34784=CARTESIAN_POINT('Ctrl Pts',(-2.60925515681931,21.2711623310641,-54.6300210443754));
#34785=CARTESIAN_POINT('Ctrl Pts',(-2.90976919678355,21.2542807820542,-54.2925838115906));
#34786=CARTESIAN_POINT('Ctrl Pts',(-4.17259771949928,21.1834525291307,-52.8271650732017));
#34787=CARTESIAN_POINT('Ctrl Pts',(-5.96614078384086,21.0834264338425,-50.5049177591858));
#34788=CARTESIAN_POINT('Ctrl Pts',(-8.23551887565116,20.9598507183575,-46.8200324861014));
#34789=CARTESIAN_POINT('Ctrl Pts',(-10.3917998591798,20.8461335954997,-42.3247528309648));
#34790=CARTESIAN_POINT('Ctrl Pts',(-11.9336389677477,20.7684839093916,-37.6328489259993));
#34791=CARTESIAN_POINT('Ctrl Pts',(-12.8608056432646,20.7206230093664,-32.8175597616776));
#34792=CARTESIAN_POINT('Ctrl Pts',(-13.2962652334972,20.6916936542703,-27.9427190446355));
#34793=CARTESIAN_POINT('Ctrl Pts',(-13.1172637173845,20.6796111419738,-23.042397384734));
#34794=CARTESIAN_POINT('Ctrl Pts',(-12.3245180251463,20.6722203558656,-18.190077858897));
#34795=CARTESIAN_POINT('Ctrl Pts',(-11.2247049129228,20.6630225594897,-14.0974459439554));
#34796=CARTESIAN_POINT('Ctrl Pts',(-10.2117545439491,20.6508204531822,-11.4357140304342));
#34797=CARTESIAN_POINT('Ctrl Pts',(-9.45356552143072,20.6394053700742,-9.71398247664349));
#34798=CARTESIAN_POINT('Ctrl Pts',(-9.2653103465393,20.6364191357732,-9.30449670135436));
#34799=CARTESIAN_POINT('Ctrl Pts',(-9.0708504506859,20.6332209087108,-8.89876866574359));
#34800=CARTESIAN_POINT('Ctrl Pts',(-2.78786144780353,21.2398788304839,-54.734986648491));
#34801=CARTESIAN_POINT('Ctrl Pts',(-3.09054674124275,21.2217224127637,-54.4028694868473));
#34802=CARTESIAN_POINT('Ctrl Pts',(-3.38879132187344,21.2038412173392,-54.0647741544324));
#34803=CARTESIAN_POINT('Ctrl Pts',(-4.64185221060926,21.1287309618461,-52.5966368693792));
#34804=CARTESIAN_POINT('Ctrl Pts',(-6.42010193270706,21.0222253289507,-50.2710574808013));
#34805=CARTESIAN_POINT('Ctrl Pts',(-8.6657758353777,20.8890564489947,-46.5837358359478));
#34806=CARTESIAN_POINT('Ctrl Pts',(-10.7937946739521,20.7641817659416,-42.0886817979723));
#34807=CARTESIAN_POINT('Ctrl Pts',(-12.3069696347546,20.6752847595175,-37.4009341484086));
#34808=CARTESIAN_POINT('Ctrl Pts',(-13.2056001710523,20.6159219251614,-32.593875126352));
#34809=CARTESIAN_POINT('Ctrl Pts',(-13.6129162346445,20.5752144761384,-27.7305920467752));
#34810=CARTESIAN_POINT('Ctrl Pts',(-13.4066122237822,20.5509334123338,-22.8460826300547));
#34811=CARTESIAN_POINT('Ctrl Pts',(-12.5879285743064,20.5308579865904,-18.0139735024298));
#34812=CARTESIAN_POINT('Ctrl Pts',(-11.4670654551122,20.510426256151,-13.9417473429775));
#34813=CARTESIAN_POINT('Ctrl Pts',(-10.441017302005,20.4905046142392,-11.2957311335189));
#34814=CARTESIAN_POINT('Ctrl Pts',(-9.67457087624675,20.4739374093561,-9.58505126521439));
#34815=CARTESIAN_POINT('Ctrl Pts',(-9.48435985345334,20.469713411733,-9.17824321596247));
#34816=CARTESIAN_POINT('Ctrl Pts',(-9.2879705742477,20.4652767483487,-8.7752182278677));
#34817=CARTESIAN_POINT('Ctrl Pts',(-3.27157466622819,21.1822016013635,-54.5083686162039));
#34818=CARTESIAN_POINT('Ctrl Pts',(-3.57199026498769,21.1630886105529,-54.1755741433477));
#34819=CARTESIAN_POINT('Ctrl Pts',(-3.867945357497,21.1442460408093,-53.8368225496259));
#34820=CARTESIAN_POINT('Ctrl Pts',(-5.11115096322305,21.0650173413637,-52.3659763157366));
#34821=CARTESIAN_POINT('Ctrl Pts',(-6.87397448879546,20.9522796229575,-50.0370826487369));
#34822=CARTESIAN_POINT('Ctrl Pts',(-9.09574496106366,20.8098799445818,-46.3473629383914));
#34823=CARTESIAN_POINT('Ctrl Pts',(-11.1952649174008,20.6742608619688,-41.8525956339481));
#34824=CARTESIAN_POINT('Ctrl Pts',(-12.6795277371662,20.5745198093833,-37.1690907037834));
#34825=CARTESIAN_POINT('Ctrl Pts',(-13.549357274074,20.5040526001987,-32.3703795244388));
#34826=CARTESIAN_POINT('Ctrl Pts',(-13.928244644041,20.4519664047462,-27.5188030016408));
#34827=CARTESIAN_POINT('Ctrl Pts',(-13.6943252090186,20.4158956934967,-22.6502962432811));
#34828=CARTESIAN_POINT('Ctrl Pts',(-12.84935865861,20.3835681705302,-17.8386311771449));
#34829=CARTESIAN_POINT('Ctrl Pts',(-11.7071209683214,20.3523071857454,-13.7870404729825));
#34830=CARTESIAN_POINT('Ctrl Pts',(-10.6677427713326,20.3249607749065,-11.1569060982881));
#34831=CARTESIAN_POINT('Ctrl Pts',(-9.89288025107589,20.3034475984546,-9.45738932777788));
#34832=CARTESIAN_POINT('Ctrl Pts',(-9.70067558073745,20.2980359714688,-9.05328776689231));
#34833=CARTESIAN_POINT('Ctrl Pts',(-9.502319413209,20.29241155197,-8.65299653157533));
#34834=CARTESIAN_POINT('Ctrl Pts',(-5.00075672518562,20.942701117012,-53.6979980175762));
#34835=CARTESIAN_POINT('Ctrl Pts',(-5.29299497875376,20.9203083949833,-53.3627895497372));
#34836=CARTESIAN_POINT('Ctrl Pts',(-5.58069899267371,20.898168919688,-53.0217006865309));
#34837=CARTESIAN_POINT('Ctrl Pts',(-6.78837683302675,20.8048139743737,-51.5412148799487));
#34838=CARTESIAN_POINT('Ctrl Pts',(-8.49560417926637,20.6706999592586,-49.2005507523738));
#34839=CARTESIAN_POINT('Ctrl Pts',(-10.6312465418532,20.496623371127,-45.5024117366326));
#34840=CARTESIAN_POINT('Ctrl Pts',(-12.6280792027309,20.3241023157428,-41.0089019403645));
#34841=CARTESIAN_POINT('Ctrl Pts',(-14.0081323264445,20.1870685788371,-36.3408814186532));
#34842=CARTESIAN_POINT('Ctrl Pts',(-14.7740833823745,20.0783595881962,-31.5724358370727));
#34843=CARTESIAN_POINT('Ctrl Pts',(-15.050345615672,19.9870599496472,-26.7632388302389));
#34844=CARTESIAN_POINT('Ctrl Pts',(-14.716602165243,19.9103458023656,-21.9526114892868));
#34845=CARTESIAN_POINT('Ctrl Pts',(-13.7764534706996,19.8358125374395,-17.2148494062985));
#34846=CARTESIAN_POINT('Ctrl Pts',(-12.5566475355216,19.767331746443,-13.2378259159173));
#34847=CARTESIAN_POINT('Ctrl Pts',(-11.4687854770212,19.7145309927478,-10.6650386217668));
#34848=CARTESIAN_POINT('Ctrl Pts',(-10.6632684791928,19.6760973304852,-9.00580897579432));
#34849=CARTESIAN_POINT('Ctrl Pts',(-10.4638019355425,19.6666248028076,-8.61148427775603));
#34850=CARTESIAN_POINT('Ctrl Pts',(-10.2582811126764,19.6569408091057,-8.22107717923549));
#34851=CARTESIAN_POINT('Ctrl Pts',(-7.46361100628468,20.4780024533914,-52.5428514904373));
#34852=CARTESIAN_POINT('Ctrl Pts',(-7.74396251989346,20.4514551579611,-52.2042338877599));
#34853=CARTESIAN_POINT('Ctrl Pts',(-8.01966600566118,20.4251375618498,-51.8598495527096));
#34854=CARTESIAN_POINT('Ctrl Pts',(-9.17564362561465,20.3138746691076,-50.3657973352887));
#34855=CARTESIAN_POINT('Ctrl Pts',(-10.8019893466219,20.1526659052326,-48.0086692011363));
#34856=CARTESIAN_POINT('Ctrl Pts',(-12.8123729854089,19.938389785095,-44.2991483331433));
#34857=CARTESIAN_POINT('Ctrl Pts',(-14.6598833650052,19.7189203495023,-39.8083335665313));
#34858=CARTESIAN_POINT('Ctrl Pts',(-15.8883904533384,19.5342279169114,-35.1635209475294));
#34859=CARTESIAN_POINT('Ctrl Pts',(-16.5032185242019,19.3763677050182,-30.4395979969074));
#34860=CARTESIAN_POINT('Ctrl Pts',(-16.6301079290243,19.2344308170631,-25.6923932190953));
#34861=CARTESIAN_POINT('Ctrl Pts',(-16.150942601219,19.1049298841923,-20.9661119486891));
#34862=CARTESIAN_POINT('Ctrl Pts',(-15.071952261372,18.9752993129734,-16.3358067118265));
#34863=CARTESIAN_POINT('Ctrl Pts',(-13.7388416841064,18.8580619466085,-12.4670750288679));
#34864=CARTESIAN_POINT('Ctrl Pts',(-12.5800312173463,18.7718242877839,-9.97749611367835));
#34865=CARTESIAN_POINT('Ctrl Pts',(-11.7296051602899,18.7111415689428,-8.37669984088804));
#34866=CARTESIAN_POINT('Ctrl Pts',(-11.5195014970783,18.6963263828107,-7.99657495662887));
#34867=CARTESIAN_POINT('Ctrl Pts',(-11.3034879690696,18.6812985797984,-7.62054189991676));
#34868=CARTESIAN_POINT('Ctrl Pts',(-11.0569415256315,19.4355555088431,-50.8552329684943));
#34869=CARTESIAN_POINT('Ctrl Pts',(-11.3192343320996,19.4044605226273,-50.5116606355265));
#34870=CARTESIAN_POINT('Ctrl Pts',(-11.5766912052793,19.3735658358572,-50.1625007339047));
#34871=CARTESIAN_POINT('Ctrl Pts',(-12.653995917516,19.2426748194849,-48.6488552478595));
#34872=CARTESIAN_POINT('Ctrl Pts',(-14.1573023261151,19.0517849995255,-46.2681979540424));
#34873=CARTESIAN_POINT('Ctrl Pts',(-15.9771942148807,18.7933185397158,-42.5433868704522));
#34874=CARTESIAN_POINT('Ctrl Pts',(-17.597612542223,18.5218580841843,-38.0587382248537));
#34875=CARTESIAN_POINT('Ctrl Pts',(-18.5955579184473,18.2836948825759,-33.4509227879516));
#34876=CARTESIAN_POINT('Ctrl Pts',(-18.9802606649373,18.0697821020849,-28.7960392710661));
#34877=CARTESIAN_POINT('Ctrl Pts',(-18.8794585829925,17.8693333343866,-24.1441381552406));
#34878=CARTESIAN_POINT('Ctrl Pts',(-18.1782482378414,17.6778661310593,-19.5467704498198));
#34879=CARTESIAN_POINT('Ctrl Pts',(-16.8867429791504,17.4826662284719,-15.0801299557059));
#34880=CARTESIAN_POINT('Ctrl Pts',(-15.3797696484439,17.3068805329357,-11.3760221291961));
#34881=CARTESIAN_POINT('Ctrl Pts',(-14.1117405005934,17.1802068447994,-9.0127555471549));
#34882=CARTESIAN_POINT('Ctrl Pts',(-13.1920422418364,17.0925519552341,-7.50061046136997));
#34883=CARTESIAN_POINT('Ctrl Pts',(-12.965539839746,17.0712544126695,-7.14207420900537));
#34884=CARTESIAN_POINT('Ctrl Pts',(-12.733360180583,17.0497370990139,-6.78793828427621));
#34885=CARTESIAN_POINT('Ctrl Pts',(-15.1119097686709,17.8320672383652,-48.9488137829308));
#34886=CARTESIAN_POINT('Ctrl Pts',(-15.3529931425318,17.7976045693245,-48.5995837467735));
#34887=CARTESIAN_POINT('Ctrl Pts',(-15.5889976518167,17.7633163796081,-48.2449887280201));
#34888=CARTESIAN_POINT('Ctrl Pts',(-16.5737137552487,17.6178640028275,-46.7091305060896));
#34889=CARTESIAN_POINT('Ctrl Pts',(-17.9322327728079,17.4049846203341,-44.3020244766142));
#34890=CARTESIAN_POINT('Ctrl Pts',(-19.5279513167919,17.1135517229592,-40.5609220746071));
#34891=CARTESIAN_POINT('Ctrl Pts',(-20.8810506766434,16.8027253827761,-36.0853303795502));
#34892=CARTESIAN_POINT('Ctrl Pts',(-21.6074270786827,16.523022337621,-31.5226206762998));
#34893=CARTESIAN_POINT('Ctrl Pts',(-21.7208002337218,16.2641978724915,-26.950312603897));
#34894=CARTESIAN_POINT('Ctrl Pts',(-21.3512579632507,16.0157341831644,-22.4117014626838));
#34895=CARTESIAN_POINT('Ctrl Pts',(-20.3875400600326,15.7719994721116,-17.9669301842299));
#34896=CARTESIAN_POINT('Ctrl Pts',(-18.8442287628299,15.5202180684676,-13.6935287962594));
#34897=CARTESIAN_POINT('Ctrl Pts',(-17.1307828365004,15.2931736272884,-10.1835212283731));
#34898=CARTESIAN_POINT('Ctrl Pts',(-15.7326823378276,15.130708702949,-7.96902663040391));
#34899=CARTESIAN_POINT('Ctrl Pts',(-14.7303426130687,15.0190926843839,-6.56125019998718));
#34900=CARTESIAN_POINT('Ctrl Pts',(-14.4843031082476,14.9920326361705,-6.22819169107344));
#34901=CARTESIAN_POINT('Ctrl Pts',(-14.232891211722,14.9647422323135,-5.8999558309418));
#34902=CARTESIAN_POINT('Ctrl Pts',(-18.970908270454,15.7638142683891,-47.1328184999909));
#34903=CARTESIAN_POINT('Ctrl Pts',(-19.1907412698361,15.7283726072843,-46.7780154330218));
#34904=CARTESIAN_POINT('Ctrl Pts',(-19.4052286980466,15.6930928161318,-46.4180868298392));
#34905=CARTESIAN_POINT('Ctrl Pts',(-20.2969793577773,15.543379415412,-44.8605288213155));
#34906=CARTESIAN_POINT('Ctrl Pts',(-21.510103862618,15.3241289383934,-42.4277782313556));
#34907=CARTESIAN_POINT('Ctrl Pts',(-22.8806049730129,15.0227233638938,-38.6716539324935));
#34908=CARTESIAN_POINT('Ctrl Pts',(-23.9649653230345,14.6988957424381,-34.2066804509099));
#34909=CARTESIAN_POINT('Ctrl Pts',(-24.4180458113406,14.4035050799014,-29.6907449133417));
#34910=CARTESIAN_POINT('Ctrl Pts',(-24.2579799735948,14.1252237593235,-25.2027953528283));
#34911=CARTESIAN_POINT('Ctrl Pts',(-23.6172443794943,13.8539516979883,-20.7793517379232));
#34912=CARTESIAN_POINT('Ctrl Pts',(-22.3880897501917,13.5829362127958,-16.4891755568032));
#34913=CARTESIAN_POINT('Ctrl Pts',(-20.5895002890963,13.2994842764397,-12.4111363639204));
#34914=CARTESIAN_POINT('Ctrl Pts',(-18.6662036034684,13.0425486753816,-9.09713537144141));
#34915=CARTESIAN_POINT('Ctrl Pts',(-17.1354921955775,12.8585920936854,-7.03274207893589));
#34916=CARTESIAN_POINT('Ctrl Pts',(-16.048739648028,12.7324540777387,-5.73022824514736));
#34917=CARTESIAN_POINT('Ctrl Pts',(-15.7827885451181,12.7018988467546,-5.42292608178293));
#34918=CARTESIAN_POINT('Ctrl Pts',(-15.5118211192701,12.6711030837425,-5.12093005973719));
#34919=CARTESIAN_POINT('Ctrl Pts',(-22.5969658936558,13.2592937677246,-45.4258711593088));
#34920=CARTESIAN_POINT('Ctrl Pts',(-22.7957177855766,13.2252177231213,-45.0654769225982));
#34921=CARTESIAN_POINT('Ctrl Pts',(-22.9888377624845,13.191306123502,-44.7002131505109));
#34922=CARTESIAN_POINT('Ctrl Pts',(-23.7881792480622,13.0474600457288,-43.1210272437177));
#34923=CARTESIAN_POINT('Ctrl Pts',(-24.8567080894127,12.8372075593629,-40.6627647663409));
#34924=CARTESIAN_POINT('Ctrl Pts',(-26.0029935116187,12.5484949329477,-36.8918909076659));
#34925=CARTESIAN_POINT('Ctrl Pts',(-26.8195147395495,12.2377054846042,-32.4379437041746));
#34926=CARTESIAN_POINT('Ctrl Pts',(-26.9998173751933,11.9522310106351,-27.9693078951154));
#34927=CARTESIAN_POINT('Ctrl Pts',(-26.5663869056578,11.6797819251771,-23.5663639192412));
#34928=CARTESIAN_POINT('Ctrl Pts',(-25.6541474279455,11.4108111467242,-19.2588329729169));
#34929=CARTESIAN_POINT('Ctrl Pts',(-24.1587280567503,11.1374939458242,-15.12412018789));
#34930=CARTESIAN_POINT('Ctrl Pts',(-22.1034644686606,10.8473681096278,-11.2424340363213));
#34931=CARTESIAN_POINT('Ctrl Pts',(-19.9687094955924,10.5820480444149,-8.12537223739529));
#34932=CARTESIAN_POINT('Ctrl Pts',(-18.3040278835727,10.3910369789073,-6.21175695472705));
#34933=CARTESIAN_POINT('Ctrl Pts',(-17.1318696035033,10.2599216927486,-5.01496871371572));
#34934=CARTESIAN_POINT('Ctrl Pts',(-16.845831430263,10.2281653805015,-4.73358189890223));
#34935=CARTESIAN_POINT('Ctrl Pts',(-16.5551956536855,10.1961599190035,-4.45802969804284));
#34936=CARTESIAN_POINT('Ctrl Pts',(-26.0167061432083,10.420684636249,-43.8161837189555));
#34937=CARTESIAN_POINT('Ctrl Pts',(-26.1946291832305,10.3898269637342,-43.4501190170891));
#34938=CARTESIAN_POINT('Ctrl Pts',(-26.3666176764586,10.3591499865554,-43.079458719461));
#34939=CARTESIAN_POINT('Ctrl Pts',(-27.0744900734894,10.2291883131935,-41.4784672756312));
#34940=CARTESIAN_POINT('Ctrl Pts',(-27.999808981558,10.0401067219452,-38.9944407782196));
#34941=CARTESIAN_POINT('Ctrl Pts',(-28.9237686887517,9.78206378055234,-35.20850249419));
#34942=CARTESIAN_POINT('Ctrl Pts',(-29.474407698267,9.50499638561923,-30.7652910285251));
#34943=CARTESIAN_POINT('Ctrl Pts',(-29.3835473154896,9.24981780003299,-26.343762915146));
#34944=CARTESIAN_POINT('Ctrl Pts',(-28.6779829078192,9.00337535985762,-22.0257324189637));
#34945=CARTESIAN_POINT('Ctrl Pts',(-27.4951432333356,8.75677479408939,-17.8341016659244));
#34946=CARTESIAN_POINT('Ctrl Pts',(-25.73393053778,8.50116890088297,-13.8549385098536));
#34947=CARTESIAN_POINT('Ctrl Pts',(-23.4220006890394,8.22444592813344,-10.1697877782279));
#34948=CARTESIAN_POINT('Ctrl Pts',(-21.0754636537987,7.96804930448713,-7.24988582865412));
#34949=CARTESIAN_POINT('Ctrl Pts',(-19.2763679910782,7.78162503245108,-5.48723735239392));
#34950=CARTESIAN_POINT('Ctrl Pts',(-18.0184348821575,7.65323614745839,-4.39631216064967));
#34951=CARTESIAN_POINT('Ctrl Pts',(-17.7122933135742,7.62212996336316,-4.14090141603417));
#34952=CARTESIAN_POINT('Ctrl Pts',(-17.4020440680749,7.59076668565169,-3.89187867255944));
#34953=CARTESIAN_POINT('Ctrl Pts',(-29.153478657498,7.18298363715391,-42.3405988972462));
#34954=CARTESIAN_POINT('Ctrl Pts',(-29.3110150080358,7.15763661423686,-41.968710532368));
#34955=CARTESIAN_POINT('Ctrl Pts',(-29.4623028504942,7.13250342173354,-41.5925157737493));
#34956=CARTESIAN_POINT('Ctrl Pts',(-30.0804996917727,7.02634360727853,-39.9692026543914));
#34957=CARTESIAN_POINT('Ctrl Pts',(-30.8652738685615,6.87350147707393,-37.4586487692798));
#34958=CARTESIAN_POINT('Ctrl Pts',(-31.570631702725,6.66841421880391,-33.6565856487172));
#34959=CARTESIAN_POINT('Ctrl Pts',(-31.8593828840731,6.45075222930465,-29.2229740367431));
#34960=CARTESIAN_POINT('Ctrl Pts',(-31.5008821225295,6.25122984378583,-24.8475460187101));
#34961=CARTESIAN_POINT('Ctrl Pts',(-30.5261914416043,6.05595707526583,-20.6135492497893));
#34962=CARTESIAN_POINT('Ctrl Pts',(-29.0753280478855,5.8568061689083,-16.5370395810716));
#34963=CARTESIAN_POINT('Ctrl Pts',(-27.0503371471076,5.64398234710963,-12.7127701150548));
#34964=CARTESIAN_POINT('Ctrl Pts',(-24.4831672830312,5.40587468584602,-9.22361623976366));
#34965=CARTESIAN_POINT('Ctrl Pts',(-21.9256568997423,5.18017895256177,-6.50048971464225));
#34966=CARTESIAN_POINT('Ctrl Pts',(-19.9924050455866,5.01301666232781,-4.88860082735946));
#34967=CARTESIAN_POINT('Ctrl Pts',(-18.6487730514648,4.89707445701614,-3.90341761267217));
#34968=CARTESIAN_POINT('Ctrl Pts',(-18.3226214021972,4.86894780999335,-3.6739618069591));
#34969=CARTESIAN_POINT('Ctrl Pts',(-17.9929253405265,4.84055053954568,-3.45145291255317));
#34970=CARTESIAN_POINT('Ctrl Pts',(-31.9690930439721,3.57357815210241,-41.0180792529404));
#34971=CARTESIAN_POINT('Ctrl Pts',(-32.1068917240552,3.55599962931061,-40.6401207805861));
#34972=CARTESIAN_POINT('Ctrl Pts',(-32.2381219635969,3.53868515668548,-40.2581553674421));
#34973=CARTESIAN_POINT('Ctrl Pts',(-32.7693658218617,3.46609807861293,-38.6115622659731));
#34974=CARTESIAN_POINT('Ctrl Pts',(-33.4176633186792,3.36435917107101,-36.0730433066292));
#34975=CARTESIAN_POINT('Ctrl Pts',(-33.9101935588516,3.23426720235262,-32.2527904354527));
#34976=CARTESIAN_POINT('Ctrl Pts',(-33.9433875335791,3.10147907156715,-27.8264773869434));
#34977=CARTESIAN_POINT('Ctrl Pts',(-33.3230442294874,2.98285053627008,-23.4949825382079));
#34978=CARTESIAN_POINT('Ctrl Pts',(-32.0844634781661,2.86388130857434,-19.342983262472));
#34979=CARTESIAN_POINT('Ctrl Pts',(-30.3703524340721,2.73730530568202,-15.3796595222941));
#34980=CARTESIAN_POINT('Ctrl Pts',(-28.0857727571174,2.59247375589619,-11.7084699295552));
#34981=CARTESIAN_POINT('Ctrl Pts',(-25.2669562806955,2.41842603756845,-8.41361075233248));
#34982=CARTESIAN_POINT('Ctrl Pts',(-22.5011430936133,2.24547053120763,-5.88587199558128));
#34983=CARTESIAN_POINT('Ctrl Pts',(-20.4352434834371,2.11246131963295,-4.423861375631));
#34984=CARTESIAN_POINT('Ctrl Pts',(-19.0068166510242,2.01884144332686,-3.54385338001933));
#34985=CARTESIAN_POINT('Ctrl Pts',(-18.6609406970972,1.99605339732081,-3.34020224802802));
#34986=CARTESIAN_POINT('Ctrl Pts',(-18.3121499863602,1.9729679754383,-3.14404091243222));
#34987=CARTESIAN_POINT('Ctrl Pts',(-34.1445283674067,0.237308438758995,
-39.9981929654655));
#34988=CARTESIAN_POINT('Ctrl Pts',(-34.2659507766525,0.227921876287717,
-39.6148155006927));
#34989=CARTESIAN_POINT('Ctrl Pts',(-34.3805279861517,0.218854274805993,
-39.2276946514564));
#34990=CARTESIAN_POINT('Ctrl Pts',(-34.8395344608935,0.181679983795775,
-37.5602873097401));
#34991=CARTESIAN_POINT('Ctrl Pts',(-35.3742864588916,0.133848323063104,
-34.996502923227));
#34992=CARTESIAN_POINT('Ctrl Pts',(-35.689296702141,0.0830496793456984,
-31.158781314165));
#34993=CARTESIAN_POINT('Ctrl Pts',(-35.508860093127,0.0403924264632703,
-26.7366100715681));
#34994=CARTESIAN_POINT('Ctrl Pts',(-34.6691074999777,0.00837005963384143,
-22.4407523838643));
#34995=CARTESIAN_POINT('Ctrl Pts',(-33.2089581147195,-0.0279539839125438,
-18.3571071296996));
#34996=CARTESIAN_POINT('Ctrl Pts',(-31.2735021578734,-0.0750512999789021,
-14.4889393778444));
#34997=CARTESIAN_POINT('Ctrl Pts',(-28.77030238607,-0.14423024726241,-10.9471823477048));
#34998=CARTESIAN_POINT('Ctrl Pts',(-25.7392642180907,-0.245792879606331,
-7.81715607344157));
#34999=CARTESIAN_POINT('Ctrl Pts',(-22.7976079423453,-0.358291148292244,
-5.45547658199914));
#35000=CARTESIAN_POINT('Ctrl Pts',(-20.6196310618627,-0.451704594358635,
-4.12101639283359));
#35001=CARTESIAN_POINT('Ctrl Pts',(-19.1195316867098,-0.519340602547392,
-3.33056337659497));
#35002=CARTESIAN_POINT('Ctrl Pts',(-18.7570395705057,-0.535923052101836,
-3.14886314137711));
#35003=CARTESIAN_POINT('Ctrl Pts',(-18.3922183482205,-0.552841667182328,
-2.97509251221366));
#35004=CARTESIAN_POINT('Ctrl Pts',(-35.4242625444563,-2.14030259993981,
-39.3999067907448));
#35005=CARTESIAN_POINT('Ctrl Pts',(-35.5351906676675,-2.14321532053782,
-39.0127533168375));
#35006=CARTESIAN_POINT('Ctrl Pts',(-35.6390899705067,-2.14576465810466,
-38.6220306854052));
#35007=CARTESIAN_POINT('Ctrl Pts',(-36.0517533718566,-2.15494826818845,
-36.9400382714986));
#35008=CARTESIAN_POINT('Ctrl Pts',(-36.513530409794,-2.16016260296573,-34.3583397184339));
#35009=CARTESIAN_POINT('Ctrl Pts',(-36.7140964838328,-2.1481556077715,-30.5074117705083));
#35010=CARTESIAN_POINT('Ctrl Pts',(-36.3955751956867,-2.11918777525101,
-26.0862334557496));
#35011=CARTESIAN_POINT('Ctrl Pts',(-35.4136079539949,-2.08197924289826,
-21.812429632092));
#35012=CARTESIAN_POINT('Ctrl Pts',(-33.8095227208381,-2.05170003121316,
-17.7727099144858));
#35013=CARTESIAN_POINT('Ctrl Pts',(-31.7300551335314,-2.03426137368081,
-13.9663813266482));
#35014=CARTESIAN_POINT('Ctrl Pts',(-29.0843808269317,-2.04135770257883,
-10.5093678461129));
#35015=CARTESIAN_POINT('Ctrl Pts',(-25.9148616326331,-2.08278583441843,
-7.48773188556975));
#35016=CARTESIAN_POINT('Ctrl Pts',(-22.8583671131416,-2.14471303148954,
-5.23550264905522));
#35017=CARTESIAN_POINT('Ctrl Pts',(-20.6071497187297,-2.20477046252904,
-3.98525510992991));
#35018=CARTESIAN_POINT('Ctrl Pts',(-19.0602046224515,-2.25046208753918,
-3.25396976945851));
#35019=CARTESIAN_POINT('Ctrl Pts',(-18.6868772548584,-2.26180965939547,
-3.08675753401129));
#35020=CARTESIAN_POINT('Ctrl Pts',(-18.3116275119647,-2.27353152926925,
-2.92775054349675));
#35021=CARTESIAN_POINT('Ctrl Pts',(-36.2458754281875,-3.83428286431684,
-39.0165372468892));
#35022=CARTESIAN_POINT('Ctrl Pts',(-36.3497179357597,-3.83237339034492,
-38.6267050482277));
#35023=CARTESIAN_POINT('Ctrl Pts',(-36.4464049450996,-3.83006698099443,
-38.2334239905326));
#35024=CARTESIAN_POINT('Ctrl Pts',(-36.827755913052,-3.81839846831683,-36.5410559830271));
#35025=CARTESIAN_POINT('Ctrl Pts',(-37.2401729585333,-3.79185933798401,
-33.9465304329049));
#35026=CARTESIAN_POINT('Ctrl Pts',(-37.3631874453177,-3.73301479320489,
-30.0858254407128));
#35027=CARTESIAN_POINT('Ctrl Pts',(-36.9509520321193,-3.65055513724086,
-25.6645975154325));
#35028=CARTESIAN_POINT('Ctrl Pts',(-35.8723140298153,-3.56151400652134,
-21.4053271089361));
#35029=CARTESIAN_POINT('Ctrl Pts',(-34.170266900352,-3.48120332570528,-17.3952827734835));
#35030=CARTESIAN_POINT('Ctrl Pts',(-31.9927051724745,-3.41513875248544,
-13.6310298223079));
#35031=CARTESIAN_POINT('Ctrl Pts',(-29.2499014363018,-3.37526128513496,
-10.2319449785824));
#35032=CARTESIAN_POINT('Ctrl Pts',(-25.9859204297108,-3.37099617994084,
-7.28460114094662));
#35033=CARTESIAN_POINT('Ctrl Pts',(-22.8510661243058,-3.39437469848804,
-5.10749779158423));
#35034=CARTESIAN_POINT('Ctrl Pts',(-20.5498647319002,-3.42893690611626,
-3.91511396280375));
#35035=CARTESIAN_POINT('Ctrl Pts',(-18.9709493935299,-3.45783930783476,
-3.22450080356909));
#35036=CARTESIAN_POINT('Ctrl Pts',(-18.5902381355287,-3.46518513130081,
-3.06723973368515));
#35037=CARTESIAN_POINT('Ctrl Pts',(-18.2078921549279,-3.47293757911652,
-2.91836533081347));
#35038=CARTESIAN_POINT('Ctrl Pts',(-36.4655794448433,-4.30636894546118,
-38.9141058712393));
#35039=CARTESIAN_POINT('Ctrl Pts',(-36.5674940832915,-4.3031084050989,-38.5235258839868));
#35040=CARTESIAN_POINT('Ctrl Pts',(-36.6622180197793,-4.29944065268701,
-38.1295298100554));
#35041=CARTESIAN_POINT('Ctrl Pts',(-37.0350431681583,-4.28192251284736,
-36.4342583416843));
#35042=CARTESIAN_POINT('Ctrl Pts',(-37.4340027033603,-4.24645759656194,
-33.8361337960593));
#35043=CARTESIAN_POINT('Ctrl Pts',(-37.5358283873113,-4.17439213330946,
-29.9726517814578));
#35044=CARTESIAN_POINT('Ctrl Pts',(-37.0979456046996,-4.07676875425951,
-25.5513313272549));
#35045=CARTESIAN_POINT('Ctrl Pts',(-35.9928116326167,-3.97294922980807,
-21.296010801273));
#35046=CARTESIAN_POINT('Ctrl Pts',(-34.2638927997542,-3.87828739688684,
-17.2941090731212));
#35047=CARTESIAN_POINT('Ctrl Pts',(-32.0594214767088,-3.79820251809058,
-13.5414254218137));
#35048=CARTESIAN_POINT('Ctrl Pts',(-29.2899822669843,-3.74469501429227,
-10.1582784319748));
#35049=CARTESIAN_POINT('Ctrl Pts',(-26.0001245878037,-3.72710099262819,
-7.23136065579539));
#35050=CARTESIAN_POINT('Ctrl Pts',(-22.843837540975,-3.7392015362719,-5.07488539244714));
#35051=CARTESIAN_POINT('Ctrl Pts',(-20.5289842613135,-3.76629674044718,
-3.89837054749424));
#35052=CARTESIAN_POINT('Ctrl Pts',(-18.9413452630501,-3.79028538091932,
-3.21890267223375));
#35053=CARTESIAN_POINT('Ctrl Pts',(-18.558620753541,-3.79646095010219,-3.06436626748395));
#35054=CARTESIAN_POINT('Ctrl Pts',(-18.1743414502133,-3.80305340259771,
-2.9182640862329));
#35055=CARTESIAN_POINT('Ctrl Pts',(-36.6775857957588,-4.78145508078572,
-38.8153455871797));
#35056=CARTESIAN_POINT('Ctrl Pts',(-36.7776062638762,-4.77682808742727,
-38.4240131371284));
#35057=CARTESIAN_POINT('Ctrl Pts',(-36.8704007885924,-4.7717826224726,-38.0292964530863));
#35058=CARTESIAN_POINT('Ctrl Pts',(-37.234843496037,-4.74834091216943,-36.3310936653698));
#35059=CARTESIAN_POINT('Ctrl Pts',(-37.6205540771554,-4.70381966688121,
-33.729326641453));
#35060=CARTESIAN_POINT('Ctrl Pts',(-37.7014739516717,-4.61828583278682,
-29.8630026526442));
#35061=CARTESIAN_POINT('Ctrl Pts',(-37.2382435623926,-4.50515190400754,
-25.4415155647569));
#35062=CARTESIAN_POINT('Ctrl Pts',(-36.10688371564,-4.38613315046716,-21.190074076811));
#35063=CARTESIAN_POINT('Ctrl Pts',(-34.3513451208948,-4.27662792828432,
-17.1962429261849));
#35064=CARTESIAN_POINT('Ctrl Pts',(-32.1202148359084,-4.18197237106197,
-13.4550487006667));
#35065=CARTESIAN_POINT('Ctrl Pts',(-29.3243976191462,-4.11421750462538,
-10.0877374299455));
#35066=CARTESIAN_POINT('Ctrl Pts',(-26.0089405061619,-4.08262421860679,
-7.18109960770556));
#35067=CARTESIAN_POINT('Ctrl Pts',(-22.8314832033504,-4.0828488851085,-5.04507681792322));
#35068=CARTESIAN_POINT('Ctrl Pts',(-20.5031646226372,-4.10207414795096,
-3.88427613292033));
#35069=CARTESIAN_POINT('Ctrl Pts',(-18.9069293129407,-4.12088738197538,
-3.2158356955667));
#35070=CARTESIAN_POINT('Ctrl Pts',(-18.5222216096196,-4.12583098108427,
-3.0639936442264));
#35071=CARTESIAN_POINT('Ctrl Pts',(-18.1360384644055,-4.13120272145022,
-2.92063144712372));
#35072=CARTESIAN_POINT('',(-9.59372125972938,20.7105311502984,-45.8827377044908));
#35073=CARTESIAN_POINT('Ctrl Pts',(-9.5937212597294,20.7105311502984,-45.8827377044908));
#35074=CARTESIAN_POINT('Ctrl Pts',(-11.9656966255223,20.5483438544848,-41.273662205894));
#35075=CARTESIAN_POINT('Ctrl Pts',(-13.4213771307776,20.4520245495079,-36.2040060452052));
#35076=CARTESIAN_POINT('Ctrl Pts',(-14.4263273756746,20.3052748660675,-25.8880364474773));
#35077=CARTESIAN_POINT('Ctrl Pts',(-13.978485237413,20.248474007324,-20.6405355948745));
#35078=CARTESIAN_POINT('Ctrl Pts',(-12.5441843191278,20.1925493450898,-15.6634703684439));
#35079=CARTESIAN_POINT('',(-37.032580314656,-3.27137091447505,-28.7376553268898));
#35080=CARTESIAN_POINT('Ctrl Pts',(-9.59372125972839,20.7105311502992,-45.8827377044852));
#35081=CARTESIAN_POINT('Ctrl Pts',(-12.689974521814,19.9641940681955,-45.2353349371288));
#35082=CARTESIAN_POINT('Ctrl Pts',(-15.6237739429307,18.7336189223951,-44.2899044956698));
#35083=CARTESIAN_POINT('Ctrl Pts',(-21.3095375661309,15.6437709263415,-41.8792648939248));
#35084=CARTESIAN_POINT('Ctrl Pts',(-24.0969041079348,13.6706054953475,-40.3166248003805));
#35085=CARTESIAN_POINT('Ctrl Pts',(-28.9050095453594,9.45712578015132,-37.0129844875419));
#35086=CARTESIAN_POINT('Ctrl Pts',(-31.0016800075678,7.182688558081,-35.2467154850527));
#35087=CARTESIAN_POINT('Ctrl Pts',(-34.5055399597611,2.26699026933606,-31.8194310502729));
#35088=CARTESIAN_POINT('Ctrl Pts',(-35.9295603487439,-0.36522399219569,
-30.1590544146936));
#35089=CARTESIAN_POINT('Ctrl Pts',(-37.0325806584272,-3.27137053313469,
-28.7376548139838));
#35090=CARTESIAN_POINT('Ctrl Pts',(-37.0325798368516,-3.27137100135122,
-28.7376553603834));
#35091=CARTESIAN_POINT('Ctrl Pts',(-36.9761954831548,-3.25992112204953,
-27.9630010274032));
#35092=CARTESIAN_POINT('Ctrl Pts',(-36.8905408508367,-3.24789096533568,
-27.1935900368743));
#35093=CARTESIAN_POINT('Ctrl Pts',(-36.7763506206657,-3.23555894384663,
-26.4309495822826));
#35094=CARTESIAN_POINT('Ctrl Pts',(-36.4966946574327,-3.20535738156791,
-24.5632157962139));
#35095=CARTESIAN_POINT('Ctrl Pts',(-36.0458884752206,-3.17334534347451,
-22.7360903115206));
#35096=CARTESIAN_POINT('Ctrl Pts',(-35.4348689964149,-3.14345008158506,
-20.9719738284514));
#35097=CARTESIAN_POINT('Ctrl Pts',(-35.0275226565476,-3.12351990598109,
-19.7958961134128));
#35098=CARTESIAN_POINT('Ctrl Pts',(-34.5489703998561,-3.10453051989494,
-18.6478224019152));
#35099=CARTESIAN_POINT('Ctrl Pts',(-34.0024927143669,-3.08752071373526,
-17.5343714336233));
#35100=CARTESIAN_POINT('Ctrl Pts',(-33.4560150291637,-3.07051090758448,
-16.4209204659143));
#35101=CARTESIAN_POINT('Ctrl Pts',(-32.8416119152349,-3.0554806813514,-15.342092241367));
#35102=CARTESIAN_POINT('Ctrl Pts',(-32.162579197906,-3.04339100491456,-14.3044960466025));
#35103=CARTESIAN_POINT('Ctrl Pts',(-31.1440301231784,-3.02525649028182,
-12.74810175639));
#35104=CARTESIAN_POINT('Ctrl Pts',(-29.9800644412201,-3.01373821257335,
-11.284479532925));
#35105=CARTESIAN_POINT('Ctrl Pts',(-28.6818918835157,-3.01128625574909,
-9.93585464417003));
#35106=CARTESIAN_POINT('Ctrl Pts',(-27.8164435137448,-3.00965161787008,
-9.03677138711117));
#35107=CARTESIAN_POINT('Ctrl Pts',(-26.891347643875,-3.01204645592803,-8.18879805630125));
#35108=CARTESIAN_POINT('Ctrl Pts',(-25.9099387717161,-3.01891855380822,
-7.39849523212083));
#35109=CARTESIAN_POINT('Ctrl Pts',(-24.9285300172334,-3.02579065086441,
-6.60819250270197));
#35110=CARTESIAN_POINT('Ctrl Pts',(-23.8908082739512,-3.03714000665748,
-5.87556026604573));
#35111=CARTESIAN_POINT('Ctrl Pts',(-22.8001058140645,-3.05321938564873,
-5.20714428357849));
#35112=CARTESIAN_POINT('Ctrl Pts',(-22.3506640922016,-3.05984515577954,
-4.93171258599896));
#35113=CARTESIAN_POINT('Ctrl Pts',(-21.8922263256852,-3.06727406915266,
-4.66718473035009));
#35114=CARTESIAN_POINT('Ctrl Pts',(-21.4250255310232,-3.07550335254719,
-4.41401723611861));
#35115=CARTESIAN_POINT('Ctrl Pts',(-36.8218388167228,-4.68328060676847,
-38.751295439731));
#35116=CARTESIAN_POINT('Ctrl Pts',(-36.9217087088858,-4.67927906663786,
-38.3585621385122));
#35117=CARTESIAN_POINT('Ctrl Pts',(-37.014288976107,-4.67486342687383,-37.962433466881));
#35118=CARTESIAN_POINT('Ctrl Pts',(-37.3764699113101,-4.65418501649615,
-36.2631808787972));
#35119=CARTESIAN_POINT('Ctrl Pts',(-37.7581985948115,-4.61395560865182,
-33.6622303832942));
#35120=CARTESIAN_POINT('Ctrl Pts',(-37.8331190147459,-4.53496565777432,
-29.7973573317513));
#35121=CARTESIAN_POINT('Ctrl Pts',(-37.3628812674897,-4.42959393838223,
-25.3778345391439));
#35122=CARTESIAN_POINT('Ctrl Pts',(-36.2245349411945,-4.31850354734918,
-21.1287082650676));
#35123=CARTESIAN_POINT('Ctrl Pts',(-34.4620735486552,-4.2170896233612,-17.1375634223537));
#35124=CARTESIAN_POINT('Ctrl Pts',(-32.224084021324,-4.13063759391767,-13.3993703876313));
#35125=CARTESIAN_POINT('Ctrl Pts',(-29.421520970621,-4.07121155600733,-10.0354694255977));
#35126=CARTESIAN_POINT('Ctrl Pts',(-26.0994749828814,-4.04803120464602,
-7.13267369659695));
#35127=CARTESIAN_POINT('Ctrl Pts',(-22.9164994170118,-4.055480889925,-5.00025025831193));
#35128=CARTESIAN_POINT('Ctrl Pts',(-20.5846089679859,-4.07952578289679,
-3.84205015737256));
#35129=CARTESIAN_POINT('Ctrl Pts',(-18.9840129497197,-4.10152925776619,
-3.17453027868918));
#35130=CARTESIAN_POINT('Ctrl Pts',(-18.5967019960699,-4.1072571624472,-3.02235727198848));
#35131=CARTESIAN_POINT('Ctrl Pts',(-18.2079217603241,-4.11341014061892,
-2.87876106338383));
#35132=CARTESIAN_POINT('Ctrl Pts',(-36.5588964654534,-4.24009445412503,
-38.8740584245357));
#35133=CARTESIAN_POINT('Ctrl Pts',(-36.6608783697925,-4.23725223817857,
-38.4820550867501));
#35134=CARTESIAN_POINT('Ctrl Pts',(-36.755609154871,-4.23400446880359,-38.0866187243054));
#35135=CARTESIAN_POINT('Ctrl Pts',(-37.1271020213035,-4.21832863439708,
-36.3901431019892));
#35136=CARTESIAN_POINT('Ctrl Pts',(-37.52349683041,-4.18572164472913,-33.7925669388741));
#35137=CARTESIAN_POINT('Ctrl Pts',(-37.6214603144111,-4.11799618192084,
-29.9300480653258));
#35138=CARTESIAN_POINT('Ctrl Pts',(-37.1790710704798,-4.02550335874969,
-25.5100196056566));
#35139=CARTESIAN_POINT('Ctrl Pts',(-36.0694515065602,-3.92690475481451,
-21.2562075949406));
#35140=CARTESIAN_POINT('Ctrl Pts',(-34.3360977835797,-3.83755718932749,
-17.2560411757399));
#35141=CARTESIAN_POINT('Ctrl Pts',(-32.1272437511178,-3.76285616468038,
-13.5052822838444));
#35142=CARTESIAN_POINT('Ctrl Pts',(-29.3535072956654,-3.71481495977278,
-10.1243046163367));
#35143=CARTESIAN_POINT('Ctrl Pts',(-26.0594639791076,-3.70275434803773,
-7.19981235881089));
#35144=CARTESIAN_POINT('Ctrl Pts',(-22.8996775036204,-3.71962751323487,
-5.04559718311213));
#35145=CARTESIAN_POINT('Ctrl Pts',(-20.5825598194173,-3.74992063397164,
-3.87071007387643));
#35146=CARTESIAN_POINT('Ctrl Pts',(-18.9914165768469,-3.77604797989279,
-3.19148231513987));
#35147=CARTESIAN_POINT('Ctrl Pts',(-18.606295054631,-3.78276245762616,-3.03643732004868));
#35148=CARTESIAN_POINT('Ctrl Pts',(-18.2196164583466,-3.78989370687861,
-2.88992075118384));
#35149=CARTESIAN_POINT('Ctrl Pts',(-36.290673376604,-3.80075287541765,-38.9993534436856));
#35150=CARTESIAN_POINT('Ctrl Pts',(-36.3947878507366,-3.79905339336963,
-38.6080734652654));
#35151=CARTESIAN_POINT('Ctrl Pts',(-36.4916895026568,-3.79695621683146,
-38.2133222519409));
#35152=CARTESIAN_POINT('Ctrl Pts',(-36.872579939312,-3.78620663871065,-36.5195907613128));
#35153=CARTESIAN_POINT('Ctrl Pts',(-37.2837599710986,-3.76109400159902,
-33.9253412532604));
#35154=CARTESIAN_POINT('Ctrl Pts',(-37.4049126075535,-3.70440674399875,
-30.0651155870792));
#35155=CARTESIAN_POINT('Ctrl Pts',(-36.9905070830313,-3.62448835210827,
-25.6445247857299));
#35156=CARTESIAN_POINT('Ctrl Pts',(-35.9097128452123,-3.53802316526296,
-21.3859911440621));
#35157=CARTESIAN_POINT('Ctrl Pts',(-34.2055389888196,-3.46032715355504,
-17.376786716545));
#35158=CARTESIAN_POINT('Ctrl Pts',(-32.025881660209,-3.39690914788247,-13.6134581369143));
#35159=CARTESIAN_POINT('Ctrl Pts',(-29.2810301768391,-3.35971861494906,
-10.2154057282584));
#35160=CARTESIAN_POINT('Ctrl Pts',(-26.0150609941361,-3.35817927654809,
-7.26920630790089));
#35161=CARTESIAN_POINT('Ctrl Pts',(-22.8785479745878,-3.38391914529348,
-5.09316256015692));
#35162=CARTESIAN_POINT('Ctrl Pts',(-20.5762738134618,-3.42007079724739,
-3.90153887791587));
#35163=CARTESIAN_POINT('Ctrl Pts',(-18.9946367288233,-3.45006162272336,
-3.21055807057412));
#35164=CARTESIAN_POINT('Ctrl Pts',(-18.6117176519029,-3.45770043113048,
-3.05262827696875));
#35165=CARTESIAN_POINT('Ctrl Pts',(-18.2271537838515,-3.46574819271174,
-2.903176732322));
#35166=CARTESIAN_POINT('Ctrl Pts',(-35.326274595645,-2.2653457359543,-39.4500974478482));
#35167=CARTESIAN_POINT('Ctrl Pts',(-35.4379808442489,-2.26761569662348,
-39.0613392238265));
#35168=CARTESIAN_POINT('Ctrl Pts',(-35.5426083546314,-2.26951335386862,
-38.6689747224565));
#35169=CARTESIAN_POINT('Ctrl Pts',(-35.9569344920503,-2.27586002752392,
-36.9847938818377));
#35170=CARTESIAN_POINT('Ctrl Pts',(-36.4206636132443,-2.27671432942662,
-34.4020927243131));
#35171=CARTESIAN_POINT('Ctrl Pts',(-36.6240902972401,-2.25814179129592,
-30.5497210056551));
#35172=CARTESIAN_POINT('Ctrl Pts',(-36.3088242271421,-2.2214798205824,-26.1269314979888));
#35173=CARTESIAN_POINT('Ctrl Pts',(-35.3300068268744,-2.17652897108851,
-21.8516114957386));
#35174=CARTESIAN_POINT('Ctrl Pts',(-33.7289661625207,-2.13845241575724,
-17.8104750562544));
#35175=CARTESIAN_POINT('Ctrl Pts',(-31.6524613437962,-2.11316923258448,
-14.0028112042569));
#35176=CARTESIAN_POINT('Ctrl Pts',(-29.0096518231127,-2.11235831802136,
-10.5445663919547));
#35177=CARTESIAN_POINT('Ctrl Pts',(-25.8429103198821,-2.14581153060268,
-7.52180526966867));
#35178=CARTESIAN_POINT('Ctrl Pts',(-22.7887438706414,-2.20085463389179,
-5.26868502893114));
#35179=CARTESIAN_POINT('Ctrl Pts',(-20.5390486779056,-2.25628908058851,
-4.01789268754426));
#35180=CARTESIAN_POINT('Ctrl Pts',(-18.9911128255576,-2.29898278275007,
-3.28532599364926));
#35181=CARTESIAN_POINT('Ctrl Pts',(-18.6160074043562,-2.30966173471912,
-3.11717983531058));
#35182=CARTESIAN_POINT('Ctrl Pts',(-18.2389512637551,-2.32072459453129,
-2.95732567869355));
#35183=CARTESIAN_POINT('Ctrl Pts',(-33.5155942144999,0.42091842584111,-40.2974780341865));
#35184=CARTESIAN_POINT('Ctrl Pts',(-33.6410979392138,0.412015546281074,
-39.9131480760228));
#35185=CARTESIAN_POINT('Ctrl Pts',(-33.7597625875287,0.403442573942463,
-39.5249756224605));
#35186=CARTESIAN_POINT('Ctrl Pts',(-34.2348236846508,0.368526239150617,
-37.8575734340774));
#35187=CARTESIAN_POINT('Ctrl Pts',(-34.793938864872,0.324281374370589,-35.2950638376772));
#35188=CARTESIAN_POINT('Ctrl Pts',(-35.1465248468338,0.279215865745994,
-31.4560451821976));
#35189=CARTESIAN_POINT('Ctrl Pts',(-35.0108071356808,0.243759038204317,
-27.0285126878594));
#35190=CARTESIAN_POINT('Ctrl Pts',(-34.2164710060877,0.21967725703067,-22.7223557888659));
#35191=CARTESIAN_POINT('Ctrl Pts',(-32.8018337863586,0.192114722189047,
-18.6232863589188));
#35192=CARTESIAN_POINT('Ctrl Pts',(-30.9116489876761,0.154437491851918,
-14.7354972118828));
#35193=CARTESIAN_POINT('Ctrl Pts',(-28.4530247891845,0.0954817696064694,
-11.1687518835629));
#35194=CARTESIAN_POINT('Ctrl Pts',(-25.4652872492237,0.0048363712043943,
-8.00819339300858));
#35195=CARTESIAN_POINT('Ctrl Pts',(-22.5596132517522,-0.0979118428630517,
-5.61646217028398));
#35196=CARTESIAN_POINT('Ctrl Pts',(-20.4047003250856,-0.184631554593919,
-4.25932715177338));
#35197=CARTESIAN_POINT('Ctrl Pts',(-18.9175087484012,-0.247909792323189,
-3.45203690874275));
#35198=CARTESIAN_POINT('Ctrl Pts',(-18.5565095119815,-0.263520166061751,
-3.26551414254701));
#35199=CARTESIAN_POINT('Ctrl Pts',(-18.1930293280116,-0.279478515480188,
-3.08692920705276));
#35200=CARTESIAN_POINT('Ctrl Pts',(-30.7058158632503,3.93922736422659,-41.6156780667464));
#35201=CARTESIAN_POINT('Ctrl Pts',(-30.8512244437417,3.92273017306588,-41.2373131455902));
#35202=CARTESIAN_POINT('Ctrl Pts',(-30.9901280488388,3.90651491483579,-40.8547832308081));
#35203=CARTESIAN_POINT('Ctrl Pts',(-31.5527136406494,3.83888692720806,-39.209945734774));
#35204=CARTESIAN_POINT('Ctrl Pts',(-32.2490817339818,3.74496038387833,-36.6743179499844));
#35205=CARTESIAN_POINT('Ctrl Pts',(-32.8157306685883,3.6271896762232,-32.8520021930134));
#35206=CARTESIAN_POINT('Ctrl Pts',(-32.9371004388341,3.50969140214063,-28.415607351119));
#35207=CARTESIAN_POINT('Ctrl Pts',(-32.4062568303131,3.40771510315772,-24.064179586933));
#35208=CARTESIAN_POINT('Ctrl Pts',(-31.2572950158716,3.30695483103527,-19.8820198922113));
#35209=CARTESIAN_POINT('Ctrl Pts',(-29.6322618431089,3.1998573133211,-15.8801579160552));
#35210=CARTESIAN_POINT('Ctrl Pts',(-27.4352928661237,3.07607789704229,-12.1597154252998));
#35211=CARTESIAN_POINT('Ctrl Pts',(-24.7014561356057,2.92448144596071,-8.8045323297206));
#35212=CARTESIAN_POINT('Ctrl Pts',(-22.0061590174955,2.77158317941627,-6.21733539620513));
#35213=CARTESIAN_POINT('Ctrl Pts',(-19.9853803676448,2.65236568914073,-4.71041174116156));
#35214=CARTESIAN_POINT('Ctrl Pts',(-18.584109044878,2.56779645721963,-3.79791853180525));
#35215=CARTESIAN_POINT('Ctrl Pts',(-18.2431180339001,2.54707902977605,-3.58548942342471));
#35216=CARTESIAN_POINT('Ctrl Pts',(-17.8989488792197,2.52604544176493,-3.38046479825666));
#35217=CARTESIAN_POINT('Ctrl Pts',(-27.2065229004271,7.64857049485316,-43.2599712710379));
#35218=CARTESIAN_POINT('Ctrl Pts',(-27.375180737316,7.62538079009264,-42.8882187054049));
#35219=CARTESIAN_POINT('Ctrl Pts',(-27.5377062922894,7.6024320797305,-42.5119551641807));
#35220=CARTESIAN_POINT('Ctrl Pts',(-28.2023793530123,7.50598047950645,-40.8922328334449));
#35221=CARTESIAN_POINT('Ctrl Pts',(-29.0586537190346,7.36825978906471,-38.3863291832077));
#35222=CARTESIAN_POINT('Ctrl Pts',(-29.8741803512828,7.18657585481396,-34.5817019673071));
#35223=CARTESIAN_POINT('Ctrl Pts',(-30.2938961583478,6.99739878870591,-30.1336568230252));
#35224=CARTESIAN_POINT('Ctrl Pts',(-30.0681891276577,6.82819742189185,-25.729106971718));
#35225=CARTESIAN_POINT('Ctrl Pts',(-29.226307184173,6.66543158101024,-21.4507349741909));
#35226=CARTESIAN_POINT('Ctrl Pts',(-27.9073056775005,6.50060855796851,-17.3173530581892));
#35227=CARTESIAN_POINT('Ctrl Pts',(-26.0118012369813,6.32441606849526,-13.420225676104));
#35228=CARTESIAN_POINT('Ctrl Pts',(-23.5699870405407,6.12505774886043,-9.84169230501458));
#35229=CARTESIAN_POINT('Ctrl Pts',(-21.1163074171586,5.93384517916791,-7.0303844759557));
#35230=CARTESIAN_POINT('Ctrl Pts',(-19.24935046319,5.79035915091665,-5.35183470637228));
#35231=CARTESIAN_POINT('Ctrl Pts',(-17.9465329640227,5.69001969995687,-4.3188326702563));
#35232=CARTESIAN_POINT('Ctrl Pts',(-17.6285601762503,5.66551509710643,-4.07669727210146));
#35233=CARTESIAN_POINT('Ctrl Pts',(-17.3066979614427,5.64071489355821,-3.84132255077521));
#35234=CARTESIAN_POINT('Ctrl Pts',(-23.9106075275297,10.6050661536892,-44.8102927658334));
#35235=CARTESIAN_POINT('Ctrl Pts',(-24.0999482352423,10.5777689837161,-44.4441954546609));
#35236=CARTESIAN_POINT('Ctrl Pts',(-24.2834699596018,10.5506896266998,-44.0733056545029));
#35237=CARTESIAN_POINT('Ctrl Pts',(-25.0388108524095,10.4365567481294,-42.4751911006532));
#35238=CARTESIAN_POINT('Ctrl Pts',(-26.0369733432726,10.2719415070743,-39.9947595312251));
#35239=CARTESIAN_POINT('Ctrl Pts',(-27.0729575257367,10.0511774947007,-36.204886014752));
#35240=CARTESIAN_POINT('Ctrl Pts',(-27.7565345002429,9.81863871620139,-31.7458974134181));
#35241=CARTESIAN_POINT('Ctrl Pts',(-27.8001970917429,9.60967367489776,-27.2942342918104));
#35242=CARTESIAN_POINT('Ctrl Pts',(-27.2289251235294,9.41153176383594,-22.9311595449484));
#35243=CARTESIAN_POINT('Ctrl Pts',(-26.1792365799165,9.21500541081661,-18.6822692512467));
#35244=CARTESIAN_POINT('Ctrl Pts',(-24.5485602461104,9.01175979868378,-14.6302206321163));
#35245=CARTESIAN_POINT('Ctrl Pts',(-22.3628067019381,8.78956564702969,-10.8560325847683));
#35246=CARTESIAN_POINT('Ctrl Pts',(-20.1206530946606,8.58124477590158,-7.84850018302945));
#35247=CARTESIAN_POINT('Ctrl Pts',(-18.3881253877929,8.42762540105217,-6.0197322565147));
#35248=CARTESIAN_POINT('Ctrl Pts',(-17.1712672933703,8.32086564673385,-4.88126724545499));
#35249=CARTESIAN_POINT('Ctrl Pts',(-16.873476253482,8.29482075310626,-4.61312950964513));
#35250=CARTESIAN_POINT('Ctrl Pts',(-16.5712568612584,8.26849188852043,-4.35118157863571));
#35251=CARTESIAN_POINT('Ctrl Pts',(-19.9077523571373,13.6252616883324,-46.6938992239532));
#35252=CARTESIAN_POINT('Ctrl Pts',(-20.1209446867673,13.5952855444977,-46.3342027946698));
#35253=CARTESIAN_POINT('Ctrl Pts',(-20.328655271869,13.5655149131873,-45.9694174486435));
#35254=CARTESIAN_POINT('Ctrl Pts',(-21.1883542692841,13.4398628522405,-44.3959569514256));
#35255=CARTESIAN_POINT('Ctrl Pts',(-22.3497277547974,13.2576618204372,-41.944601857953));
#35256=CARTESIAN_POINT('Ctrl Pts',(-23.6389889994787,13.0115743729063,-38.1716237995733));
#35257=CARTESIAN_POINT('Ctrl Pts',(-24.6253432650482,12.751644575675,-33.700270230942));
#35258=CARTESIAN_POINT('Ctrl Pts',(-24.9776401721497,12.5189796899122,-29.195033885056));
#35259=CARTESIAN_POINT('Ctrl Pts',(-24.7159386768495,12.301865256328,-24.7355540748207));
#35260=CARTESIAN_POINT('Ctrl Pts',(-23.973932481888,12.0904144587841,-20.3551525544938));
#35261=CARTESIAN_POINT('Ctrl Pts',(-22.6452804926613,11.8774764455751,-16.1266720944649));
#35262=CARTESIAN_POINT('Ctrl Pts',(-20.7509637909255,11.6504923923572,-12.1296170528026));
#35263=CARTESIAN_POINT('Ctrl Pts',(-18.7491181417974,11.4410171343385,-8.89853855417975));
#35264=CARTESIAN_POINT('Ctrl Pts',(-17.1689877263805,11.2882220371981,-6.89861628429694));
#35265=CARTESIAN_POINT('Ctrl Pts',(-16.0494601752109,11.1823584691134,-5.63998274787565));
#35266=CARTESIAN_POINT('Ctrl Pts',(-15.7746139887752,11.1565388193505,-5.34224033696405));
#35267=CARTESIAN_POINT('Ctrl Pts',(-15.4948206145188,11.1304479812224,-5.05005712611216));
#35268=CARTESIAN_POINT('Ctrl Pts',(-16.2180432174767,15.9398275064074,-48.4301828651543));
#35269=CARTESIAN_POINT('Ctrl Pts',(-16.4521938275456,15.9092719019138,-48.076086901104));
#35270=CARTESIAN_POINT('Ctrl Pts',(-16.6811358152299,15.8789225535602,-47.7166629869837));
#35271=CARTESIAN_POINT('Ctrl Pts',(-17.6323385975404,15.7507918597713,-46.1649547628248));
#35272=CARTESIAN_POINT('Ctrl Pts',(-18.936758193489,15.5646999212503,-43.7393392481435));
#35273=CARTESIAN_POINT('Ctrl Pts',(-20.4478002103812,15.3133344724918,-39.9816616098395));
#35274=CARTESIAN_POINT('Ctrl Pts',(-21.6990238014656,15.0487502016962,-35.5001764568839));
#35275=CARTESIAN_POINT('Ctrl Pts',(-22.3209682180315,14.8142492774957,-30.9488592309027));
#35276=CARTESIAN_POINT('Ctrl Pts',(-22.3293422064976,14.5991383033468,-26.4059293305493));
#35277=CARTESIAN_POINT('Ctrl Pts',(-21.8554243838307,14.3930646018661,-21.9114461411382));
#35278=CARTESIAN_POINT('Ctrl Pts',(-20.7894641003817,14.1899609567462,-17.5296852489892));
#35279=CARTESIAN_POINT('Ctrl Pts',(-19.1480898546693,13.977122935371,-13.3388231592936));
#35280=CARTESIAN_POINT('Ctrl Pts',(-17.3543937104353,13.7824369346935,-9.91324173232946));
#35281=CARTESIAN_POINT('Ctrl Pts',(-15.9059529139166,13.6409944051188,-7.76433835467781));
#35282=CARTESIAN_POINT('Ctrl Pts',(-14.8704133561947,13.5429643472183,-6.40108514071164));
#35283=CARTESIAN_POINT('Ctrl Pts',(-14.6154376715172,13.5190447294408,-6.07761083543428));
#35284=CARTESIAN_POINT('Ctrl Pts',(-14.3551373099958,13.4948677704672,-5.75918559466514));
#35285=CARTESIAN_POINT('Ctrl Pts',(-11.822716088486,18.188947172369,-50.4975069982862));
#35286=CARTESIAN_POINT('Ctrl Pts',(-12.0807460479859,18.1597316481657,-50.149900849382));
#35287=CARTESIAN_POINT('Ctrl Pts',(-12.3338504324003,18.1307342364494,-49.7967145807944));
#35288=CARTESIAN_POINT('Ctrl Pts',(-13.3890724600746,18.0083786966032,-48.2704339664839));
#35289=CARTESIAN_POINT('Ctrl Pts',(-14.85607927955,17.830846834045,-45.87512597419));
#35290=CARTESIAN_POINT('Ctrl Pts',(-16.6190813424255,17.5925027676131,-42.1363421540281));
#35291=CARTESIAN_POINT('Ctrl Pts',(-18.1710314843799,17.3443426911773,-37.6450078774674));
#35292=CARTESIAN_POINT('Ctrl Pts',(-19.098835784666,17.1289494695207,-33.042870247926));
#35293=CARTESIAN_POINT('Ctrl Pts',(-19.4131698285569,16.9369213116231,-28.4065295399037));
#35294=CARTESIAN_POINT('Ctrl Pts',(-19.2425984638769,16.7575317657622,-23.7837227318492));
#35295=CARTESIAN_POINT('Ctrl Pts',(-18.4733495985464,16.5859876106103,-19.2289587859595));
#35296=CARTESIAN_POINT('Ctrl Pts',(-17.1170188880216,16.4095763329362,-14.8188969944352));
#35297=CARTESIAN_POINT('Ctrl Pts',(-15.5573630806058,16.2491906636996,-11.1730748288595));
#35298=CARTESIAN_POINT('Ctrl Pts',(-14.2565853340076,16.1323920433636,-8.85532759071016));
#35299=CARTESIAN_POINT('Ctrl Pts',(-13.3150650046537,16.0510402241362,-7.37346260225604));
#35300=CARTESIAN_POINT('Ctrl Pts',(-13.0823954562657,16.0311583490605,-7.02088379334164));
#35301=CARTESIAN_POINT('Ctrl Pts',(-12.8440411184632,16.01103806515,-6.67284079394564));
#35302=CARTESIAN_POINT('Ctrl Pts',(-7.8411699938905,19.7983627848149,-52.3687269376966));
#35303=CARTESIAN_POINT('Ctrl Pts',(-8.11992829303053,19.7720645135703,-52.0269336332472));
#35304=CARTESIAN_POINT('Ctrl Pts',(-8.39398168231564,19.7460021313493,-51.6793544625476));
#35305=CARTESIAN_POINT('Ctrl Pts',(-9.53928451332661,19.6361820466171,-50.1760284730572));
#35306=CARTESIAN_POINT('Ctrl Pts',(-11.14709799416,19.4774394485581,-47.8083359664954));
#35307=CARTESIAN_POINT('Ctrl Pts',(-13.1282713733665,19.2670183310104,-44.0877853258967));
#35308=CARTESIAN_POINT('Ctrl Pts',(-14.9405198598359,19.0520629838802,-39.5898882349583));
#35309=CARTESIAN_POINT('Ctrl Pts',(-16.1328704916667,18.8717166252608,-34.9454307905654));
#35310=CARTESIAN_POINT('Ctrl Pts',(-16.7115351800607,18.7178122962125,-30.2296013374526));
#35311=CARTESIAN_POINT('Ctrl Pts',(-16.8027339787928,18.5794411422907,-25.4968369057016));
#35312=CARTESIAN_POINT('Ctrl Pts',(-16.289068982041,18.4529446490623,-20.7931224538683));
#35313=CARTESIAN_POINT('Ctrl Pts',(-15.1776736379726,18.3257380682571,-16.1937918909369));
#35314=CARTESIAN_POINT('Ctrl Pts',(-13.818636740357,18.2102139945187,-12.3575006396806));
#35315=CARTESIAN_POINT('Ctrl Pts',(-12.6440494074441,18.1249152482566,-9.89355822405953));
#35316=CARTESIAN_POINT('Ctrl Pts',(-11.7827259364293,18.064727637235,-8.30894077759558));
#35317=CARTESIAN_POINT('Ctrl Pts',(-11.5691191440624,18.0499634327475,-7.93121921616813));
#35318=CARTESIAN_POINT('Ctrl Pts',(-11.3495571850093,18.0349776243875,-7.5576561263274));
#35319=CARTESIAN_POINT('Ctrl Pts',(-4.92431549867914,20.6836496418694,-53.7378814684056));
#35320=CARTESIAN_POINT('Ctrl Pts',(-5.21764882463673,20.6606519170286,-53.4003910101086));
#35321=CARTESIAN_POINT('Ctrl Pts',(-5.50641809554749,20.6379063239872,-53.0569754366587));
#35322=CARTESIAN_POINT('Ctrl Pts',(-6.71493902102225,20.5422448076096,-51.5707569872934));
#35323=CARTESIAN_POINT('Ctrl Pts',(-8.42160241882005,20.4047755971079,-49.2238878429916));
#35324=CARTESIAN_POINT('Ctrl Pts',(-10.5559839035698,20.225761668211,-45.5180413008222));
#35325=CARTESIAN_POINT('Ctrl Pts',(-12.5510196597057,20.0475517349526,-41.0174600421653));
#35326=CARTESIAN_POINT('Ctrl Pts',(-13.9290667150874,19.9048724048602,-36.3448359479815));
#35327=CARTESIAN_POINT('Ctrl Pts',(-14.6931006487833,19.790507905872,-31.5743538869703));
#35328=CARTESIAN_POINT('Ctrl Pts',(-14.9676760376565,19.6935273080542,-26.7652261036137));
#35329=CARTESIAN_POINT('Ctrl Pts',(-14.6327324280219,19.6110850660289,-21.9573646480998));
#35330=CARTESIAN_POINT('Ctrl Pts',(-13.6921672345661,19.530779076001,-17.2251601923033));
#35331=CARTESIAN_POINT('Ctrl Pts',(-12.4726763896338,19.4573327991495,-13.2548574676923));
#35332=CARTESIAN_POINT('Ctrl Pts',(-11.3855615935515,19.4012238336331,-10.6878836640295));
#35333=CARTESIAN_POINT('Ctrl Pts',(-10.579708766175,19.3605693891818,-9.03080166569367));
#35334=CARTESIAN_POINT('Ctrl Pts',(-10.3792982715972,19.3505226070412,-8.63539384629041));
#35335=CARTESIAN_POINT('Ctrl Pts',(-10.17275733115,19.3402634731691,-8.24392214707791));
#35336=CARTESIAN_POINT('Ctrl Pts',(-3.28313391958304,21.117312799858,-54.5077715750056));
#35337=CARTESIAN_POINT('Ctrl Pts',(-3.58453926185978,21.0964267127388,-54.1727240990175));
#35338=CARTESIAN_POINT('Ctrl Pts',(-3.88145363778616,21.0758020890032,-53.8316755867277));
#35339=CARTESIAN_POINT('Ctrl Pts',(-5.12494438152081,20.9891913310095,-52.3551981425261));
#35340=CARTESIAN_POINT('Ctrl Pts',(-6.88629963355924,20.8653273744228,-50.0202471636553));
#35341=CARTESIAN_POINT('Ctrl Pts',(-9.10547002832004,20.7063681300896,-46.323055763502));
#35342=CARTESIAN_POINT('Ctrl Pts',(-11.2016741138313,20.5515335415639,-41.8215054727501));
#35343=CARTESIAN_POINT('Ctrl Pts',(-12.6824932627098,20.4326519806542,-37.1336983778281));
#35344=CARTESIAN_POINT('Ctrl Pts',(-13.549084907869,20.3430531321453,-32.3332605226414));
#35345=CARTESIAN_POINT('Ctrl Pts',(-13.9250741545097,20.2718184169426,-27.4820679213417));
#35346=CARTESIAN_POINT('Ctrl Pts',(-13.6888986754112,20.2165549432469,-22.6166458941869));
#35347=CARTESIAN_POINT('Ctrl Pts',(-12.8426375694204,20.164982094833,-17.8108595922544));
#35348=CARTESIAN_POINT('Ctrl Pts',(-11.7000922537864,20.117197691553,-13.7662661051264));
#35349=CARTESIAN_POINT('Ctrl Pts',(-10.6611372059216,20.0788282397779,-11.1421302429153));
#35350=CARTESIAN_POINT('Ctrl Pts',(-9.88579572272463,20.0500302875854,-9.44483158002572));
#35351=CARTESIAN_POINT('Ctrl Pts',(-9.69264545280016,20.0428451797642,-9.03962286423958));
#35352=CARTESIAN_POINT('Ctrl Pts',(-9.49327031140026,20.0354515632684,-8.63824109957652));
#35353=CARTESIAN_POINT('Ctrl Pts',(-2.8163592485811,21.2334813897109,-54.7266862394484));
#35354=CARTESIAN_POINT('Ctrl Pts',(-3.12005132129948,21.2132228077857,-54.3923338233844));
#35355=CARTESIAN_POINT('Ctrl Pts',(-3.41927252450223,21.1932283095702,-54.051958820629));
#35356=CARTESIAN_POINT('Ctrl Pts',(-4.67266466131728,21.1093059289188,-52.578253438475));
#35357=CARTESIAN_POINT('Ctrl Pts',(-6.44950317520521,20.9894835119608,-50.2466975711262));
#35358=CARTESIAN_POINT('Ctrl Pts',(-8.69266751409434,20.8364792943525,-46.5519878921847));
#35359=CARTESIAN_POINT('Ctrl Pts',(-10.8174853479259,20.6885792302246,-42.0502021694425));
#35360=CARTESIAN_POINT('Ctrl Pts',(-12.3273479522208,20.5767478260626,-37.3581435871616));
#35361=CARTESIAN_POINT('Ctrl Pts',(-13.2228929109269,20.4944756050622,-32.5492847655305));
#35362=CARTESIAN_POINT('Ctrl Pts',(-13.6274817449899,20.4308554028779,-27.6862587662835));
#35363=CARTESIAN_POINT('Ctrl Pts',(-13.4191180933562,20.3836340081555,-22.8046364371979));
#35364=CARTESIAN_POINT('Ctrl Pts',(-12.5993630644216,20.340580727313,-17.9781318076291));
#35365=CARTESIAN_POINT('Ctrl Pts',(-11.4784037767259,20.3004356869138,-13.9126108423358));
#35366=CARTESIAN_POINT('Ctrl Pts',(-10.4529327913986,20.2673681898868,-11.272358363803));
#35367=CARTESIAN_POINT('Ctrl Pts',(-9.68612423728318,20.2421246596599,-9.56371335956087));
#35368=CARTESIAN_POINT('Ctrl Pts',(-9.49500452080127,20.2357981340653,-9.15574211803836));
#35369=CARTESIAN_POINT('Ctrl Pts',(-9.29763363791485,20.2292648564311,-8.75156952718668));
#35370=CARTESIAN_POINT('Ctrl Pts',(-2.34821392037626,21.3428689572265,-54.9461960408909));
#35371=CARTESIAN_POINT('Ctrl Pts',(-2.65418949424281,21.323266505305,-54.6125406100865));
#35372=CARTESIAN_POINT('Ctrl Pts',(-2.95571399231871,21.303930781031,-54.2728409939294));
#35373=CARTESIAN_POINT('Ctrl Pts',(-4.21899114535187,21.2228186866547,-52.8019155745608));
#35374=CARTESIAN_POINT('Ctrl Pts',(-6.0112853374839,21.1072213437662,-50.4737675281765));
#35375=CARTESIAN_POINT('Ctrl Pts',(-8.27839193827317,20.9604400919523,-46.7815631436401));
#35376=CARTESIAN_POINT('Ctrl Pts',(-10.4317474491813,20.819779963638,-42.2795772720142));
#35377=CARTESIAN_POINT('Ctrl Pts',(-11.9705535559543,20.7152993064879,-37.5833174183362));
#35378=CARTESIAN_POINT('Ctrl Pts',(-12.8949237610472,20.6406553883908,-32.7661078399796));
#35379=CARTESIAN_POINT('Ctrl Pts',(-13.3279556694048,20.5849601975755,-27.8913403249881));
#35380=CARTESIAN_POINT('Ctrl Pts',(-13.1472110199265,20.5461109852346,-22.9936375250261));
#35381=CARTESIAN_POINT('Ctrl Pts',(-12.353730422049,20.5119420676311,-18.1465609279757));
#35382=CARTESIAN_POINT('Ctrl Pts',(-11.2541276071585,20.4797911688045,-14.0602526474523));
#35383=CARTESIAN_POINT('Ctrl Pts',(-10.2419708153508,20.4522911786996,-11.4039786634214));
#35384=CARTESIAN_POINT('Ctrl Pts',(-9.48357772483115,20.4307901345004,-9.68404750188143));
#35385=CARTESIAN_POINT('Ctrl Pts',(-9.29446059008481,20.4253683033402,-9.27333014503118));
#35386=CARTESIAN_POINT('Ctrl Pts',(-9.09906630802712,20.4197421663948,-8.86638496754931));
#35387=CARTESIAN_POINT('',(-9.57349520052307,20.5529756002067,-45.8869621655533));
#35388=CARTESIAN_POINT('Ctrl Pts',(-37.0325800073215,-3.27137127985419,
-28.7376556530266));
#35389=CARTESIAN_POINT('Ctrl Pts',(-34.5044867351128,1.76302065361439,-31.995465657097));
#35390=CARTESIAN_POINT('Ctrl Pts',(-30.8416008390371,6.26298702225072,-35.7871583427932));
#35391=CARTESIAN_POINT('Ctrl Pts',(-23.5458744462642,12.5188402724799,-40.6337606863442));
#35392=CARTESIAN_POINT('Ctrl Pts',(-20.9044174504492,14.4577038717082,-42.0668269045533));
#35393=CARTESIAN_POINT('Ctrl Pts',(-15.4358826795028,17.848637426394,-44.3535277717808));
#35394=CARTESIAN_POINT('Ctrl Pts',(-12.5747622055328,19.3555632898771,-45.2608009663176));
#35395=CARTESIAN_POINT('Ctrl Pts',(-9.57349520052268,20.5529756002057,-45.8869621655533));
#35396=CARTESIAN_POINT('Ctrl Pts',(-12.693647630517,19.9464420456703,-16.2756753502908));
#35397=CARTESIAN_POINT('Ctrl Pts',(-14.0225517860209,20.0189549105364,-21.1794341117034));
#35398=CARTESIAN_POINT('Ctrl Pts',(-14.4019245709807,20.0954766247834,-26.3285862792967));
#35399=CARTESIAN_POINT('Ctrl Pts',(-13.3354239934069,20.2752040736289,-36.426648889325));
#35400=CARTESIAN_POINT('Ctrl Pts',(-11.8914352859286,20.3824974081049,-41.3760085159638));
#35401=CARTESIAN_POINT('Ctrl Pts',(-9.57349520052296,20.5529756002056,-45.8869621655532));
#35402=CARTESIAN_POINT('Ctrl Pts',(-4.32846278832924,20.9435908393615,-53.6183358849051));
#35403=CARTESIAN_POINT('Ctrl Pts',(-4.42954047863754,20.9358615047579,-53.5003794779475));
#35404=CARTESIAN_POINT('Ctrl Pts',(-4.53061816894586,20.9281321701544,-53.3824230709899));
#35405=CARTESIAN_POINT('Ctrl Pts',(-4.63169585925417,20.9204028355509,-53.2644666640323));
#35406=CARTESIAN_POINT('Ctrl Pts',(-14.7394648900858,20.1474693751975,-41.4688259682726));
#35407=CARTESIAN_POINT('Ctrl Pts',(-16.9746112199935,20.0812550388979,-23.7323694053441));
#35408=CARTESIAN_POINT('Ctrl Pts',(-10.2693271530803,19.8399463130827,-9.7334219899501));
#35409=CARTESIAN_POINT('Ctrl Pts',(-4.32855128811855,20.9469886892296,-53.6183010608916));
#35410=CARTESIAN_POINT('Ctrl Pts',(-4.42963628382275,20.9392720585054,-53.5003480807636));
#35411=CARTESIAN_POINT('Ctrl Pts',(-4.53072127952695,20.9315554277811,-53.3823951006357));
#35412=CARTESIAN_POINT('Ctrl Pts',(-4.63180627523115,20.9238387970569,-53.2644421205078));
#35413=CARTESIAN_POINT('Ctrl Pts',(-14.7403058456515,20.1521757246323,-41.4691441077164));
#35414=CARTESIAN_POINT('Ctrl Pts',(-16.9750472014194,20.0873688943554,-23.7324733387566));
#35415=CARTESIAN_POINT('Ctrl Pts',(-10.2700125053852,19.8474084919615,-9.73349139492549));
#35416=CARTESIAN_POINT('Ctrl Pts',(-4.32863978790787,20.9503865390978,-53.618266236878));
#35417=CARTESIAN_POINT('Ctrl Pts',(-4.42973208900795,20.9426826122528,-53.5003166835798));
#35418=CARTESIAN_POINT('Ctrl Pts',(-4.53082439010804,20.9349786854078,-53.3823671302816));
#35419=CARTESIAN_POINT('Ctrl Pts',(-4.63191669120813,20.9272747585629,-53.2644175769833));
#35420=CARTESIAN_POINT('Ctrl Pts',(-14.7411468012171,20.1568820740671,-41.4694622471602));
#35421=CARTESIAN_POINT('Ctrl Pts',(-16.9754831828453,20.093482749813,-23.7325772721691));
#35422=CARTESIAN_POINT('Ctrl Pts',(-10.27069785769,19.8548706708402,-9.73356079990087));
#35423=CARTESIAN_POINT('Ctrl Pts',(-4.32872828769718,20.9537843889659,-53.6182314128645));
#35424=CARTESIAN_POINT('Ctrl Pts',(-4.42982789419316,20.9460931660003,-53.500285286396));
#35425=CARTESIAN_POINT('Ctrl Pts',(-4.53092750068913,20.9384019430346,-53.3823391599274));
#35426=CARTESIAN_POINT('Ctrl Pts',(-4.63202710718511,20.9307107200689,-53.2643930334589));
#35427=CARTESIAN_POINT('Ctrl Pts',(-14.7419877567828,20.1615884235019,-41.469780386604));
#35428=CARTESIAN_POINT('Ctrl Pts',(-16.9759191642713,20.0995966052706,-23.7326812055816));
#35429=CARTESIAN_POINT('Ctrl Pts',(-10.2713832099948,19.862332849719,-9.73363020487625));
#35430=CARTESIAN_POINT('Ctrl Pts',(-4.3289970382214,20.9641027630587,-53.6181256615179));
#35431=CARTESIAN_POINT('Ctrl Pts',(-4.43011882927837,20.9564501184246,-53.5001899414275));
#35432=CARTESIAN_POINT('Ctrl Pts',(-4.53124062033534,20.9487974737906,-53.3822542213371));
#35433=CARTESIAN_POINT('Ctrl Pts',(-4.63236241139232,20.9411448291565,-53.2643185012467));
#35434=CARTESIAN_POINT('Ctrl Pts',(-14.7445415170896,20.1758803657488,-41.4707464922068));
#35435=CARTESIAN_POINT('Ctrl Pts',(-16.9772431249007,20.1181627721728,-23.7329968239499));
#35436=CARTESIAN_POINT('Ctrl Pts',(-10.2734644442286,19.8849935193208,-9.73384096948556));
#35437=CARTESIAN_POINT('Ctrl Pts',(-4.32953453931903,20.9847395112521,-53.6179141585457));
#35438=CARTESIAN_POINT('Ctrl Pts',(-4.43070069948158,20.9771640232786,-53.4999992513047));
#35439=CARTESIAN_POINT('Ctrl Pts',(-4.53186685964413,20.9695885353052,-53.3820843440637));
#35440=CARTESIAN_POINT('Ctrl Pts',(-4.63303301980668,20.9620130473318,-53.2641694368227));
#35441=CARTESIAN_POINT('Ctrl Pts',(-14.7496490360618,20.2044642499886,-41.4726787127218));
#35442=CARTESIAN_POINT('Ctrl Pts',(-16.979891048797,20.1552951062578,-23.7336280561961));
#35443=CARTESIAN_POINT('Ctrl Pts',(-10.2776269126961,19.9303148585245,-9.7342624987041));
#35444=CARTESIAN_POINT('Ctrl Pts',(-4.33034079481653,21.0156946339229,-53.6175968855001));
#35445=CARTESIAN_POINT('Ctrl Pts',(-4.43157350735379,21.0082348808134,-53.4997132037288));
#35446=CARTESIAN_POINT('Ctrl Pts',(-4.53280621989104,21.000775127704,-53.3818295219576));
#35447=CARTESIAN_POINT('Ctrl Pts',(-4.63403893242831,20.9933153745945,-53.2639458401864));
#35448=CARTESIAN_POINT('Ctrl Pts',(-14.7573101861541,20.2473400636495,-41.475577663063));
#35449=CARTESIAN_POINT('Ctrl Pts',(-16.9838631037067,20.2109936225946,-23.7345746294339));
#35450=CARTESIAN_POINT('Ctrl Pts',(-10.2838706153973,19.9982968673298,-9.73489479253199));
#35451=CARTESIAN_POINT('Ctrl Pts',(-4.33114705535237,21.0466497571015,-53.6172795880003));
#35452=CARTESIAN_POINT('Ctrl Pts',(-4.43244631858488,21.0393057386868,-53.4994271398503));
#35453=CARTESIAN_POINT('Ctrl Pts',(-4.53374558181739,21.0319617202721,-53.3815746917003));
#35454=CARTESIAN_POINT('Ctrl Pts',(-4.6350448450499,21.0246177018574,-53.2637222435503));
#35455=CARTESIAN_POINT('Ctrl Pts',(-14.7649711683006,20.2902158603888,-41.4784774285487));
#35456=CARTESIAN_POINT('Ctrl Pts',(-16.9878353803218,20.2666921589687,-23.735520837746));
#35457=CARTESIAN_POINT('Ctrl Pts',(-10.2901143180985,20.0662788761352,-9.73552708635984));
#35458=CARTESIAN_POINT('Ctrl Pts',(-4.33168456489443,21.0672865061488,-53.6170680439928));
#35459=CARTESIAN_POINT('Ctrl Pts',(-4.43302819441772,21.0600196441101,-53.4992364223706));
#35460=CARTESIAN_POINT('Ctrl Pts',(-4.534371823941,21.0527527820714,-53.3814048007483));
#35461=CARTESIAN_POINT('Ctrl Pts',(-4.63571545346429,21.0454859200326,-53.2635731791261));
#35462=CARTESIAN_POINT('Ctrl Pts',(-14.7700784057928,20.3187997161584,-41.480411016901));
#35463=CARTESIAN_POINT('Ctrl Pts',(-16.9904836763181,20.3038245267329,-23.7361514571359));
#35464=CARTESIAN_POINT('Ctrl Pts',(-10.294276786566,20.1116002153389,-9.73594861557842));
#35465=CARTESIAN_POINT('Ctrl Pts',(-4.33195331968768,21.0776048806767,-53.6169622718518));
#35466=CARTESIAN_POINT('Ctrl Pts',(-4.43331913234895,21.0703765968246,-53.4991410635392));
#35467=CARTESIAN_POINT('Ctrl Pts',(-4.53468494501022,21.0631483129724,-53.3813198552266));
#35468=CARTESIAN_POINT('Ctrl Pts',(-4.63605075767149,21.0559200291202,-53.263498646914));
#35469=CARTESIAN_POINT('Ctrl Pts',(-14.7726320237987,20.3330916439037,-41.4813778156538));
#35470=CARTESIAN_POINT('Ctrl Pts',(-16.9918078255791,20.3223907107576,-23.7364667644556));
#35471=CARTESIAN_POINT('Ctrl Pts',(-10.2963580207998,20.1342608849406,-9.73615938018771));
#35472=CARTESIAN_POINT('Ctrl Pts',(-4.33197921695597,21.0785991614118,-53.6169520796261));
#35473=CARTESIAN_POINT('Ctrl Pts',(-4.43334716718907,21.0713745949617,-53.4991318747422));
#35474=CARTESIAN_POINT('Ctrl Pts',(-4.53471511742217,21.0641500285117,-53.3813116698583));
#35475=CARTESIAN_POINT('Ctrl Pts',(-4.63608306765527,21.0569254620617,-53.2634914649744));
#35476=CARTESIAN_POINT('Ctrl Pts',(-14.7728780909656,20.3344688170607,-41.4814709765845));
#35477=CARTESIAN_POINT('Ctrl Pts',(-16.9919354208798,20.3241797521467,-23.7364971475351));
#35478=CARTESIAN_POINT('Ctrl Pts',(-10.2965585689673,20.1364444718193,-9.73617968950969));
#35479=CARTESIAN_POINT('Ctrl Pts',(-4.33200511422425,21.0795934421468,-53.6169418874004));
#35480=CARTESIAN_POINT('Ctrl Pts',(-4.43337520202918,21.0723725930989,-53.4991226859452));
#35481=CARTESIAN_POINT('Ctrl Pts',(-4.53474528983412,21.0651517440511,-53.38130348449));
#35482=CARTESIAN_POINT('Ctrl Pts',(-4.63611537763905,21.0579308950032,-53.2634842830348));
#35483=CARTESIAN_POINT('Ctrl Pts',(-14.7731241581326,20.3358459902176,-41.4815641375152));
#35484=CARTESIAN_POINT('Ctrl Pts',(-16.9920630161805,20.3259687935359,-23.7365275306146));
#35485=CARTESIAN_POINT('Ctrl Pts',(-10.2967591171349,20.1386280586979,-9.73619999883167));
#35486=CARTESIAN_POINT('Ctrl Pts',(-4.33203101149253,21.0805877228818,-53.6169316951747));
#35487=CARTESIAN_POINT('Ctrl Pts',(-4.43340323686929,21.0733705912361,-53.4991134971482));
#35488=CARTESIAN_POINT('Ctrl Pts',(-4.53477546224606,21.0661534595904,-53.3812952991217));
#35489=CARTESIAN_POINT('Ctrl Pts',(-4.63614768762283,21.0589363279447,-53.2634771010952));
#35490=CARTESIAN_POINT('Ctrl Pts',(-14.7733702252996,20.3372231633746,-41.4816572984459));
#35491=CARTESIAN_POINT('Ctrl Pts',(-16.9921906114812,20.327757834925,-23.7365579136941));
#35492=CARTESIAN_POINT('Ctrl Pts',(-10.2969596653024,20.1408116455766,-9.73622030815366));
#35493=CARTESIAN_POINT('',(-9.57349520052307,20.5529756002067,-45.8869621655533));
#35494=CARTESIAN_POINT('Ctrl Pts',(41.5338854879026,21.2883239772394,-36.0695034689956));
#35495=CARTESIAN_POINT('Ctrl Pts',(41.0846323742273,21.2711623310641,-36.1012631617903));
#35496=CARTESIAN_POINT('Ctrl Pts',(40.6334458830462,21.2542807820542,-36.1258258257493));
#35497=CARTESIAN_POINT('Ctrl Pts',(38.7003746729656,21.1834525291307,-36.1994712829289));
#35498=CARTESIAN_POINT('Ctrl Pts',(35.7665128029796,21.0834264338425,-36.1538221981106));
#35499=CARTESIAN_POINT('Ctrl Pts',(31.4706193903941,20.9598507183575,-35.6306050471236));
#35500=CARTESIAN_POINT('Ctrl Pts',(26.6116490303384,20.8461335954997,-34.5136923836127));
#35501=CARTESIAN_POINT('Ctrl Pts',(21.9820498844225,20.7684839093916,-32.7937965035444));
#35502=CARTESIAN_POINT('Ctrl Pts',(17.6392262517605,20.7206230093664,-30.5164009130032));
#35503=CARTESIAN_POINT('Ctrl Pts',(13.5564176935285,20.6916936542703,-27.8174434572283));
#35504=CARTESIAN_POINT('Ctrl Pts',(9.83679756541101,20.6796111419738,-24.6221938557458));
#35505=CARTESIAN_POINT('Ctrl Pts',(6.53737025169527,20.6722203558656,-20.9770285762437));
#35506=CARTESIAN_POINT('Ctrl Pts',(4.02334403386231,20.6630225594897,-17.5654457985485));
#35507=CARTESIAN_POINT('Ctrl Pts',(2.57388245082573,20.6508204531822,-15.113926606545));
#35508=CARTESIAN_POINT('Ctrl Pts',(1.70050164113498,20.6394053700742,-13.4476684937515));
#35509=CARTESIAN_POINT('Ctrl Pts',(1.49772795208305,20.6364191357732,-13.0451744663849));
#35510=CARTESIAN_POINT('Ctrl Pts',(1.30176076245774,20.6332209087108,-12.6401723051977));
#35511=CARTESIAN_POINT('Ctrl Pts',(41.0553385871247,21.2398788304839,-36.3063481667607));
#35512=CARTESIAN_POINT('Ctrl Pts',(40.6069577406517,21.2217224127637,-36.3359253951444));
#35513=CARTESIAN_POINT('Ctrl Pts',(40.1566717112114,21.2038412173392,-36.3583034059402));
#35514=CARTESIAN_POINT('Ctrl Pts',(38.2275650759369,21.1287309618461,-36.4226172332441));
#35515=CARTESIAN_POINT('Ctrl Pts',(35.3006333280818,21.0222253289507,-36.362933817479));
#35516=CARTESIAN_POINT('Ctrl Pts',(31.0176144035341,20.8890564489947,-35.8196649322046));
#35517=CARTESIAN_POINT('Ctrl Pts',(26.1764415972354,20.7641817659416,-34.6807967040055));
#35518=CARTESIAN_POINT('Ctrl Pts',(21.5679637464527,20.6752847595175,-32.941081673653));
#35519=CARTESIAN_POINT('Ctrl Pts',(17.2493666899064,20.6159219251614,-30.6465070408524));
#35520=CARTESIAN_POINT('Ctrl Pts',(13.1931414583562,20.5752144761384,-27.9327521590155));
#35521=CARTESIAN_POINT('Ctrl Pts',(9.50290666680764,20.5509334123338,-24.7260153799557));
#35522=CARTESIAN_POINT('Ctrl Pts',(6.23545253050602,20.5308579865904,-21.0731719660711));
#35523=CARTESIAN_POINT('Ctrl Pts',(3.75050463941357,20.510426256151,-17.6578544106669));
#35524=CARTESIAN_POINT('Ctrl Pts',(2.32149642341642,20.4905046142392,-15.2058935398892));
#35525=CARTESIAN_POINT('Ctrl Pts',(1.461904576083,20.4739374093561,-13.5400701424733));
#35526=CARTESIAN_POINT('Ctrl Pts',(1.26244386876925,20.469713411733,-13.1377165065184));
#35527=CARTESIAN_POINT('Ctrl Pts',(1.06979295763457,20.4652767483487,-12.7328912152449));
#35528=CARTESIAN_POINT('Ctrl Pts',(40.5765712162756,21.1822016013635,-36.5432363573627));
#35529=CARTESIAN_POINT('Ctrl Pts',(40.1290759580594,21.1630886105529,-36.5706167703566));
#35530=CARTESIAN_POINT('Ctrl Pts',(39.6797043153639,21.1442460408093,-36.5907956150282));
#35531=CARTESIAN_POINT('Ctrl Pts',(37.7546244070558,21.0650173413637,-36.6457152698332));
#35532=CARTESIAN_POINT('Ctrl Pts',(34.834719528204,20.9522796229575,-36.5719047491734));
#35533=CARTESIAN_POINT('Ctrl Pts',(30.564729265643,20.8098799445818,-36.0084522400929));
#35534=CARTESIAN_POINT('Ctrl Pts',(25.7415493990861,20.6742608619688,-34.8474814639788));
#35535=CARTESIAN_POINT('Ctrl Pts',(21.1544150649873,20.5745198093833,-33.0878073038153));
#35536=CARTESIAN_POINT('Ctrl Pts',(16.8603017440869,20.5040526001987,-30.7759199377636));
#35537=CARTESIAN_POINT('Ctrl Pts',(12.8309540677332,20.4519664047462,-28.0472375270115));
#35538=CARTESIAN_POINT('Ctrl Pts',(9.17044859363215,20.4158956934967,-24.8288876342323));
#35539=CARTESIAN_POINT('Ctrl Pts',(5.93536538892685,20.3835681705302,-21.1682420847945));
#35540=CARTESIAN_POINT('Ctrl Pts',(3.4798777735314,20.3523071857454,-17.7490792127145));
#35541=CARTESIAN_POINT('Ctrl Pts',(2.07159762237086,20.3249607749065,-15.2965986559777));
#35542=CARTESIAN_POINT('Ctrl Pts',(1.22598078542615,20.3034475984546,-13.6311553685555));
#35543=CARTESIAN_POINT('Ctrl Pts',(1.02987911483698,20.2980359714688,-13.2289305040802));
#35544=CARTESIAN_POINT('Ctrl Pts',(0.840591872499916,20.29241155197,-12.8242719045711));
#35545=CARTESIAN_POINT('Ctrl Pts',(38.864870590485,20.942701117012,-37.389907526004));
#35546=CARTESIAN_POINT('Ctrl Pts',(38.4205864863258,20.9203083949833,-37.4093895318307));
#35547=CARTESIAN_POINT('Ctrl Pts',(37.974531956119,20.898168919688,-37.4216601598091));
#35548=CARTESIAN_POINT('Ctrl Pts',(36.0640667257951,20.8048139743737,-37.4427929138755));
#35549=CARTESIAN_POINT('Ctrl Pts',(33.1696229811387,20.6706999592586,-37.3181767877764));
#35550=CARTESIAN_POINT('Ctrl Pts',(28.9467502385986,20.496623371127,-36.6821372599687));
#35551=CARTESIAN_POINT('Ctrl Pts',(24.1885780130219,20.3241023157428,-35.4416663669379));
#35552=CARTESIAN_POINT('Ctrl Pts',(19.6785235596824,20.1870685788371,-33.6101721563812));
#35553=CARTESIAN_POINT('Ctrl Pts',(15.4728400094719,20.0783595881962,-31.2359396151031));
#35554=CARTESIAN_POINT('Ctrl Pts',(11.5406116990385,19.9870599496472,-28.4534448376217));
#35555=CARTESIAN_POINT('Ctrl Pts',(7.98759743124033,19.9103458023656,-25.1931366133823));
#35556=CARTESIAN_POINT('Ctrl Pts',(4.86963900159542,19.8358125374395,-21.5041524234108));
#35557=CARTESIAN_POINT('Ctrl Pts',(2.52081339113073,19.767331746443,-18.0708361527821));
#35558=CARTESIAN_POINT('Ctrl Pts',(1.18759818617417,19.7145309927478,-15.6162047066094));
#35559=CARTESIAN_POINT('Ctrl Pts',(0.392591845678522,19.6760973304852,-13.9519133948385));
#35560=CARTESIAN_POINT('Ctrl Pts',(0.208661738215443,19.6666248028076,-13.5501067434657));
#35561=CARTESIAN_POINT('Ctrl Pts',(0.0315693147396978,19.6569408091057,
-13.1460092493455));
#35562=CARTESIAN_POINT('Ctrl Pts',(36.4261761409748,20.4780024533914,-38.5952224603748));
#35563=CARTESIAN_POINT('Ctrl Pts',(35.986637929013,20.4514551579611,-38.6032854778725));
#35564=CARTESIAN_POINT('Ctrl Pts',(35.5454891020888,20.4251375618498,-38.6041190220481));
#35565=CARTESIAN_POINT('Ctrl Pts',(33.6566517848401,20.3138746691076,-38.5763723973499));
#35566=CARTESIAN_POINT('Ctrl Pts',(30.799764830004,20.1526659052326,-38.3782553300922));
#35567=CARTESIAN_POINT('Ctrl Pts',(26.6460909339275,19.938389785095,-37.6371881197587));
#35568=CARTESIAN_POINT('Ctrl Pts',(21.9831266869516,19.7189203495023,-36.2816526896943));
#35569=CARTESIAN_POINT('Ctrl Pts',(17.5857043101642,19.5342279169114,-34.3461449082959));
#35570=CARTESIAN_POINT('Ctrl Pts',(13.5090535945347,19.3763677050182,-31.8815190659229));
#35571=CARTESIAN_POINT('Ctrl Pts',(9.71842519564791,19.2344308170631,-29.0208914311038));
#35572=CARTESIAN_POINT('Ctrl Pts',(6.3220243987362,19.1049298841923,-25.6994767197043));
#35573=CARTESIAN_POINT('Ctrl Pts',(3.37464546431908,18.9752993129734,-21.9689400080561));
#35574=CARTESIAN_POINT('Ctrl Pts',(1.18113008703572,18.8580619466085,-18.5145574386863));
#35575=CARTESIAN_POINT('Ctrl Pts',(-0.0427945786360649,18.7718242877839,
-16.0563358690166));
#35576=CARTESIAN_POINT('Ctrl Pts',(-0.764115527911374,18.7111415689428,
-14.3933658531605));
#35577=CARTESIAN_POINT('Ctrl Pts',(-0.930311638349101,18.6963263828107,
-13.9920962059114));
#35578=CARTESIAN_POINT('Ctrl Pts',(-1.08962388875839,18.6812985797984,-13.5887572530535));
#35579=CARTESIAN_POINT('Ctrl Pts',(32.8663379166031,19.4355555088431,-40.352388449454));
#35580=CARTESIAN_POINT('Ctrl Pts',(32.4341853602501,19.4044605226273,-40.3432433773694));
#35581=CARTESIAN_POINT('Ctrl Pts',(32.0006794219008,19.3735658358572,-40.3268336283199));
#35582=CARTESIAN_POINT('Ctrl Pts',(30.1455752260411,19.2426748194849,-40.225361844379));
#35583=CARTESIAN_POINT('Ctrl Pts',(27.3470061899373,19.0517849995255,-39.9163785780022));
#35584=CARTESIAN_POINT('Ctrl Pts',(23.3001475854099,18.7933185397158,-39.0168456268584));
#35585=CARTESIAN_POINT('Ctrl Pts',(18.7835937846305,18.5218580841843,-37.4876069944926));
#35586=CARTESIAN_POINT('Ctrl Pts',(14.5588498457702,18.2836948825759,-35.3949061736525));
#35587=CARTESIAN_POINT('Ctrl Pts',(10.6796571258641,18.0697821020849,-32.7934064906319));
#35588=CARTESIAN_POINT('Ctrl Pts',(7.10550345028232,17.8693333343866,-29.8141833444967));
#35589=CARTESIAN_POINT('Ctrl Pts',(3.94833414086203,17.6778661310593,-26.3995431411007));
#35590=CARTESIAN_POINT('Ctrl Pts',(1.261414339538,17.4826662284719,-22.6048988734338));
#35591=CARTESIAN_POINT('Ctrl Pts',(-0.694991270314942,17.3068805329357,
-19.1172262254337));
#35592=CARTESIAN_POINT('Ctrl Pts',(-1.75206424347501,17.1802068447994,-16.6523685039809));
#35593=CARTESIAN_POINT('Ctrl Pts',(-2.36088439247878,17.0925519552341,-14.9905124109959));
#35594=CARTESIAN_POINT('Ctrl Pts',(-2.49997738438369,17.0712544126695,-14.5898820052411));
#35595=CARTESIAN_POINT('Ctrl Pts',(-2.63209034972266,17.0497370990139,-14.1875565005782));
#35596=CARTESIAN_POINT('Ctrl Pts',(28.8476080321524,17.8320672383652,-42.3340573620036));
#35597=CARTESIAN_POINT('Ctrl Pts',(28.4242559702612,17.7976045693245,-42.3048025675408));
#35598=CARTESIAN_POINT('Ctrl Pts',(27.9998760163417,17.7633163796081,-42.2682319449215));
#35599=CARTESIAN_POINT('Ctrl Pts',(26.1851332576131,17.6178640028275,-42.0805220574034));
#35600=CARTESIAN_POINT('Ctrl Pts',(23.4561592290513,17.4049846203341,-41.6418489334921));
#35601=CARTESIAN_POINT('Ctrl Pts',(19.5363333532145,17.1135517229592,-40.5568927329762));
#35602=CARTESIAN_POINT('Ctrl Pts',(15.1935312115776,16.8027253827761,-38.8243026322638));
#35603=CARTESIAN_POINT('Ctrl Pts',(11.1733728412317,16.523022337621,-36.5474036026815));
#35604=CARTESIAN_POINT('Ctrl Pts',(7.52791143671306,16.2641978724915,-33.7852548504584));
#35605=CARTESIAN_POINT('Ctrl Pts',(4.20988819682692,16.0157341831644,-30.6665573081524));
#35606=CARTESIAN_POINT('Ctrl Pts',(1.33569436348711,15.7719994721116,-27.1418227474879));
#35607=CARTESIAN_POINT('Ctrl Pts',(-1.04314652395158,15.5202180684676,-23.2707912034377));
#35608=CARTESIAN_POINT('Ctrl Pts',(-2.71906488312326,15.2931736272884,-19.7427113117026));
#35609=CARTESIAN_POINT('Ctrl Pts',(-3.5787250746749,15.130708702949,-17.2689175280809));
#35610=CARTESIAN_POINT('Ctrl Pts',(-4.0544204118661,15.0190926843839,-15.6075225274741));
#35611=CARTESIAN_POINT('Ctrl Pts',(-4.16141291752838,14.9920326361705,-15.2075025129441));
#35612=CARTESIAN_POINT('Ctrl Pts',(-4.26128529310459,14.9647422323135,-14.806289065777));
#35613=CARTESIAN_POINT('Ctrl Pts',(25.0217595366867,15.7638142683891,-44.2188893423579));
#35614=CARTESIAN_POINT('Ctrl Pts',(24.6072996956272,15.7283726072843,-44.1695456082369));
#35615=CARTESIAN_POINT('Ctrl Pts',(24.1921654581022,15.6930928161318,-44.1128268187239));
#35616=CARTESIAN_POINT('Ctrl Pts',(22.4184201291253,15.543379415412,-43.838904024895));
#35617=CARTESIAN_POINT('Ctrl Pts',(19.7600483717488,15.3241289383934,-43.2705677716271));
#35618=CARTESIAN_POINT('Ctrl Pts',(15.968898677068,15.0227233638938,-42.0001634916369));
#35619=CARTESIAN_POINT('Ctrl Pts',(11.8019542210027,14.6988957424381,-40.0640851202867));
#35620=CARTESIAN_POINT('Ctrl Pts',(7.98876258105558,14.4035050799014,-37.6026779566113));
#35621=CARTESIAN_POINT('Ctrl Pts',(4.57974174037815,14.1252237593235,-34.6793426631575));
#35622=CARTESIAN_POINT('Ctrl Pts',(1.52084636993269,13.8539516979883,-31.4204234207614));
#35623=CARTESIAN_POINT('Ctrl Pts',(-1.0669830575238,13.5829362127958,-27.7845505376458));
#35624=CARTESIAN_POINT('Ctrl Pts',(-3.13392029853443,13.2994842764397,-23.8357408245836));
#35625=CARTESIAN_POINT('Ctrl Pts',(-4.52575473794716,13.0425486753816,-20.2658011034729));
#35626=CARTESIAN_POINT('Ctrl Pts',(-5.18537945381502,12.8585920936854,-17.781914569308));
#35627=CARTESIAN_POINT('Ctrl Pts',(-5.52614664487988,12.7324540777387,-16.1201531218344));
#35628=CARTESIAN_POINT('Ctrl Pts',(-5.60058735037131,12.7018988467546,-15.7206244118355));
#35629=CARTESIAN_POINT('Ctrl Pts',(-5.66775192133469,12.6711030837425,-15.3204821076368));
#35630=CARTESIAN_POINT('Ctrl Pts',(21.4264044178079,13.2592937677246,-45.9895910901952));
#35631=CARTESIAN_POINT('Ctrl Pts',(21.0207170797347,13.2252177231213,-45.9202794452612));
#35632=CARTESIAN_POINT('Ctrl Pts',(20.6147340271746,13.191306123502,-45.8435284862164));
#35633=CARTESIAN_POINT('Ctrl Pts',(18.8816955041136,13.0474600457288,-45.4838725167592));
#35634=CARTESIAN_POINT('Ctrl Pts',(16.2935316715566,12.8372075593629,-44.7865804199157));
#35635=CARTESIAN_POINT('Ctrl Pts',(12.630646501664,12.5484949329477,-43.331681055911));
#35636=CARTESIAN_POINT('Ctrl Pts',(8.63931769810801,12.2377054846042,-41.1930723986167));
#35637=CARTESIAN_POINT('Ctrl Pts',(5.03318068432933,11.9522310106351,-38.5478898203658));
#35638=CARTESIAN_POINT('Ctrl Pts',(1.86105994601815,11.6797819251771,-35.4638295667092));
#35639=CARTESIAN_POINT('Ctrl Pts',(-0.937931348316951,11.4108111467242,
-32.0649104072594));
#35640=CARTESIAN_POINT('Ctrl Pts',(-3.23820124717178,11.1374939458242,-28.3177932082873));
#35641=CARTESIAN_POINT('Ctrl Pts',(-4.99158979822284,10.8473681096278,-24.2907317008292));
#35642=CARTESIAN_POINT('Ctrl Pts',(-6.09760889024641,10.5820480444149,-20.6782568121355));
#35643=CARTESIAN_POINT('Ctrl Pts',(-6.55582155513239,10.3910369789073,-18.1836367061482));
#35644=CARTESIAN_POINT('Ctrl Pts',(-6.76067954601502,10.2599216927486,-16.5210211970993));
#35645=CARTESIAN_POINT('Ctrl Pts',(-6.80233473263,10.2281653805015,-16.1219457386587));
#35646=CARTESIAN_POINT('Ctrl Pts',(-6.83656167557387,10.1961599190035,-15.7229135514833));
#35647=CARTESIAN_POINT('Ctrl Pts',(18.0357269294045,10.420684636249,-47.659627975918));
#35648=CARTESIAN_POINT('Ctrl Pts',(17.6385928198955,10.3898269637342,-47.5704962016297));
#35649=CARTESIAN_POINT('Ctrl Pts',(17.2415658583442,10.3591499865554,-47.4738593047325));
#35650=CARTESIAN_POINT('Ctrl Pts',(15.5485091238301,10.2291883131935,-47.0290943922104));
#35651=CARTESIAN_POINT('Ctrl Pts',(13.029492102221,10.0401067219452,-46.2037726571784));
#35652=CARTESIAN_POINT('Ctrl Pts',(9.493446906322,9.78206378055234,-44.5656595342354));
#35653=CARTESIAN_POINT('Ctrl Pts',(5.67628649226391,9.50499638561923,-42.2258694110056));
#35654=CARTESIAN_POINT('Ctrl Pts',(2.27604713466135,9.24981780003299,-39.3980542159176));
#35655=CARTESIAN_POINT('Ctrl Pts',(-0.660012836774006,9.00337535985762,
-36.1541737706072));
#35656=CARTESIAN_POINT('Ctrl Pts',(-3.19967324810691,8.75677479408939,-32.6159534467063));
#35657=CARTESIAN_POINT('Ctrl Pts',(-5.21261012281686,8.50116890088297,-28.7580142662565));
#35658=CARTESIAN_POINT('Ctrl Pts',(-6.65231229913932,8.22444592813344,-24.6528208257726));
#35659=CARTESIAN_POINT('Ctrl Pts',(-7.47214165787956,7.96804930448713,-20.9976952088575));
#35660=CARTESIAN_POINT('Ctrl Pts',(-7.72851793086956,7.78162503245108,-18.4921122305609));
#35661=CARTESIAN_POINT('Ctrl Pts',(-7.79712912596018,7.65323614745839,-16.8284397915245));
#35662=CARTESIAN_POINT('Ctrl Pts',(-7.80594114112445,7.62212996336316,-16.429842680561));
#35663=CARTESIAN_POINT('Ctrl Pts',(-7.80719772122039,7.59076668565169,-16.0320169120303));
#35664=CARTESIAN_POINT('Ctrl Pts',(14.9263225873298,7.18298363715391,-49.1920433928168));
#35665=CARTESIAN_POINT('Ctrl Pts',(14.5373462477221,7.15763661423686,-49.083341668369));
#35666=CARTESIAN_POINT('Ctrl Pts',(14.1488989149765,7.13250342173354,-48.9670696710061));
#35667=CARTESIAN_POINT('Ctrl Pts',(12.4943021862807,7.02634360727853,-48.4382762487368));
#35668=CARTESIAN_POINT('Ctrl Pts',(10.0421734244781,6.87350147707393,-47.4865326623943));
#35669=CARTESIAN_POINT('Ctrl Pts',(6.62981736222956,6.66841421880391,-45.6674560418548));
#35670=CARTESIAN_POINT('Ctrl Pts',(2.98344680610714,6.45075222930465,-43.1288991805643));
#35671=CARTESIAN_POINT('Ctrl Pts',(-0.21387899888273,6.25122984378583,-40.1205772506902));
#35672=CARTESIAN_POINT('Ctrl Pts',(-2.91644126996934,6.05595707526583,-36.7186795841497));
#35673=CARTESIAN_POINT('Ctrl Pts',(-5.1989863376844,5.8568061689083,-33.042686700556));
#35674=CARTESIAN_POINT('Ctrl Pts',(-6.92635942816575,5.64398234710963,-29.0750920509953));
#35675=CARTESIAN_POINT('Ctrl Pts',(-8.05368554515301,5.40587468584602,-24.8925459720573));
#35676=CARTESIAN_POINT('Ctrl Pts',(-8.58812995110823,5.18017895256177,-21.195162220079));
#35677=CARTESIAN_POINT('Ctrl Pts',(-8.6429926139357,5.01301666232781,-18.6786887740101));
#35678=CARTESIAN_POINT('Ctrl Pts',(-8.57549902139121,4.89707445701614,-17.0139432928344));
#35679=CARTESIAN_POINT('Ctrl Pts',(-8.55154256695504,4.86894780999335,-16.6158843105388));
#35680=CARTESIAN_POINT('Ctrl Pts',(-8.51994489356607,4.84055053954568,-16.219385523394));
#35681=CARTESIAN_POINT('Ctrl Pts',(12.1368282372958,3.57357815210241,-50.5688018516697));
#35682=CARTESIAN_POINT('Ctrl Pts',(11.7554123328022,3.55599962931061,-50.4408839449622));
#35683=CARTESIAN_POINT('Ctrl Pts',(11.3749590315426,3.53868515668548,-50.3053323379297));
#35684=CARTESIAN_POINT('Ctrl Pts',(9.75637557807125,3.46609807861293,-49.694041504612));
#35685=CARTESIAN_POINT('Ctrl Pts',(7.36747465897793,3.36435917107101,-48.6181602146532));
#35686=CARTESIAN_POINT('Ctrl Pts',(4.07359311144879,3.23426720235262,-46.6213471567875));
#35687=CARTESIAN_POINT('Ctrl Pts',(0.592266114139445,3.10147907156715,-43.8875382056778));
#35688=CARTESIAN_POINT('Ctrl Pts',(-2.40745520099751,2.98285053627008,-40.7018914156105));
#35689=CARTESIAN_POINT('Ctrl Pts',(-4.881376482725,2.86388130857434,-37.1448007849025));
#35690=CARTESIAN_POINT('Ctrl Pts',(-6.91129700276302,2.73730530568202,-33.3335628727181));
#35691=CARTESIAN_POINT('Ctrl Pts',(-8.35713647436029,2.59247375589619,-29.2584572853056));
#35692=CARTESIAN_POINT('Ctrl Pts',(-9.17565778305131,2.41842603756845,-25.0003067251804));
#35693=CARTESIAN_POINT('Ctrl Pts',(-9.42746720654185,2.24547053120763,-21.2618875642968));
#35694=CARTESIAN_POINT('Ctrl Pts',(-9.28244579831276,2.11246131963295,-18.7351534976944));
#35695=CARTESIAN_POINT('Ctrl Pts',(-9.07985419139475,2.01884144332686,-17.0696884188939));
#35696=CARTESIAN_POINT('Ctrl Pts',(-9.02342492784415,1.99605339732081,-16.6722973051515));
#35697=CARTESIAN_POINT('Ctrl Pts',(-8.95932258452836,1.9729679754383,-16.277297154442));
#35698=CARTESIAN_POINT('Ctrl Pts',(9.98308729044565,0.237308438758995,-51.6337369763077));
#35699=CARTESIAN_POINT('Ctrl Pts',(9.60764508493566,0.227921876287717,-51.4896368989849));
#35700=CARTESIAN_POINT('Ctrl Pts',(9.23354409583478,0.218854274805993,-51.337851066959));
#35701=CARTESIAN_POINT('Ctrl Pts',(7.64372668599397,0.181679983795775,-50.6571053064643));
#35702=CARTESIAN_POINT('Ctrl Pts',(5.30586692108267,0.133848323063104,-49.4766978346564));
#35703=CARTESIAN_POINT('Ctrl Pts',(2.10900967202317,0.0830496793456984,
-47.3302024745056));
#35704=CARTESIAN_POINT('Ctrl Pts',(-1.23588264070169,0.0403924264632703,
-44.4319527811565));
#35705=CARTESIAN_POINT('Ctrl Pts',(-4.07094224723787,0.00837005963384143,
-41.0969843078284));
#35706=CARTESIAN_POINT('Ctrl Pts',(-6.35327641927623,-0.0279539839125438,
-37.4092823789468));
#35707=CARTESIAN_POINT('Ctrl Pts',(-8.17079469610385,-0.0750512999789021,
-33.4843188337937));
#35708=CARTESIAN_POINT('Ctrl Pts',(-9.37913231578503,-0.14423024726241,
-29.3189890563375));
#35709=CARTESIAN_POINT('Ctrl Pts',(-9.93646401117645,-0.245792879606331,
-24.9976885304961));
#35710=CARTESIAN_POINT('Ctrl Pts',(-9.94880670058422,-0.358291148292244,
-21.2253259653454));
#35711=CARTESIAN_POINT('Ctrl Pts',(-9.6341833149091,-0.451704594358635,
-18.6904927531654));
#35712=CARTESIAN_POINT('Ctrl Pts',(-9.31688770623376,-0.519340602547392,
-17.0248284403669));
#35713=CARTESIAN_POINT('Ctrl Pts',(-9.23293653279146,-0.535923052101836,
-16.6281324481184));
#35714=CARTESIAN_POINT('Ctrl Pts',(-9.1413335698033,-0.552841667182328,
-16.2345595159175));
#35715=CARTESIAN_POINT('Ctrl Pts',(8.71742711504317,-2.14030259993981,-52.261248116584));
#35716=CARTESIAN_POINT('Ctrl Pts',(8.34557578703409,-2.14321532053782,-52.1065889728662));
#35717=CARTESIAN_POINT('Ctrl Pts',(7.97531637712704,-2.14576465810466,-51.9442091427789));
#35718=CARTESIAN_POINT('Ctrl Pts',(6.40299033232049,-2.15494826818845,-51.2181372647421));
#35719=CARTESIAN_POINT('Ctrl Pts',(4.09662385140589,-2.16016260296573,-49.9695063715731));
#35720=CARTESIAN_POINT('Ctrl Pts',(0.960796243239608,-2.1481556077715,-47.7253009393472));
#35721=CARTESIAN_POINT('Ctrl Pts',(-2.29722537800971,-2.11918777525101,
-44.7197113769873));
#35722=CARTESIAN_POINT('Ctrl Pts',(-5.02637319628328,-2.08197924289826,
-41.2873053734851));
#35723=CARTESIAN_POINT('Ctrl Pts',(-7.18462246766922,-2.05170003121316,
-37.5144569913459));
#35724=CARTESIAN_POINT('Ctrl Pts',(-8.86400315627726,-2.03426137368081,
-33.5154567077776));
#35725=CARTESIAN_POINT('Ctrl Pts',(-9.91725418147156,-2.04135770257883,
-29.2915725925193));
#35726=CARTESIAN_POINT('Ctrl Pts',(-10.303501409541,-2.08278583441843,-24.9295834958016));
#35727=CARTESIAN_POINT('Ctrl Pts',(-10.158671970043,-2.14471303148954,-21.1356778940573));
#35728=CARTESIAN_POINT('Ctrl Pts',(-9.73254376982651,-2.20477046252904,
-18.5960886707828));
#35729=CARTESIAN_POINT('Ctrl Pts',(-9.33978118010959,-2.25046208753918,
-16.9306893408303));
#35730=CARTESIAN_POINT('Ctrl Pts',(-9.23774716358698,-2.26180965939547,
-16.5345551280317));
#35731=CARTESIAN_POINT('Ctrl Pts',(-9.12809944685942,-2.27353152926925,
-16.1420338282393));
#35732=CARTESIAN_POINT('Ctrl Pts',(7.90542948215533,-3.83428286431684,-52.6645839345492));
#35733=CARTESIAN_POINT('Ctrl Pts',(7.53590165189136,-3.83237339034492,-52.5027148758859));
#35734=CARTESIAN_POINT('Ctrl Pts',(7.16813877523133,-3.83006698099443,-52.3331010949965));
#35735=CARTESIAN_POINT('Ctrl Pts',(5.60722374759459,-3.81839846831683,-51.5760790939397));
#35736=CARTESIAN_POINT('Ctrl Pts',(3.321604168471,-3.79185933798401,-50.2808595028402));
#35737=CARTESIAN_POINT('Ctrl Pts',(0.226485183062754,-3.73301479320489,
-47.9699259107911));
#35738=CARTESIAN_POINT('Ctrl Pts',(-2.97314542399398,-3.65055513724086,
-44.8910367634591));
#35739=CARTESIAN_POINT('Ctrl Pts',(-5.63065732580343,-3.56151400652134,
-41.3921119532622));
#35740=CARTESIAN_POINT('Ctrl Pts',(-7.70462720584958,-3.48120332570528,
-37.5611761746473));
#35741=CARTESIAN_POINT('Ctrl Pts',(-9.28995114080236,-3.41513875248544,
-33.5117165341006));
#35742=CARTESIAN_POINT('Ctrl Pts',(-10.2373525252032,-3.37526128513496,
-29.2480114872144));
#35743=CARTESIAN_POINT('Ctrl Pts',(-10.5066198560549,-3.37099617994084,
-24.8584895527468));
#35744=CARTESIAN_POINT('Ctrl Pts',(-10.25419810544,-3.39437469848804,-21.0501600279107));
#35745=CARTESIAN_POINT('Ctrl Pts',(-9.75166572177836,-3.42893690611626,
-18.5075691746829));
#35746=CARTESIAN_POINT('Ctrl Pts',(-9.30717122040251,-3.45783930783476,
-16.8425331931811));
#35747=CARTESIAN_POINT('Ctrl Pts',(-9.1927532889878,-3.46518513130081,-16.4468304726437));
#35748=CARTESIAN_POINT('Ctrl Pts',(-9.07075916440024,-3.47293757911652,
-16.0550786758666));
#35749=CARTESIAN_POINT('Ctrl Pts',(7.68836219406744,-4.30636894546118,-52.7724905334873));
#35750=CARTESIAN_POINT('Ctrl Pts',(7.31945172587889,-4.3031084050989,-52.6086479674884));
#35751=CARTESIAN_POINT('Ctrl Pts',(6.95235378291849,-4.29944065268701,-52.4370535891093));
#35752=CARTESIAN_POINT('Ctrl Pts',(5.39448449972533,-4.28192251284736,-51.6715555556563));
#35753=CARTESIAN_POINT('Ctrl Pts',(3.11444173302997,-4.24645759656194,-50.363570522352));
#35754=CARTESIAN_POINT('Ctrl Pts',(0.0303625865548424,-4.17439213330946,
-48.0343394120201));
#35755=CARTESIAN_POINT('Ctrl Pts',(-3.15334948925292,-4.07676875425951,
-44.9353406529986));
#35756=CARTESIAN_POINT('Ctrl Pts',(-5.79125328317668,-3.97294922980807,
-41.4181631696894));
#35757=CARTESIAN_POINT('Ctrl Pts',(-7.84210278345764,-3.87828739688684,
-37.5712950799821));
#35758=CARTESIAN_POINT('Ctrl Pts',(-9.40160361738414,-3.79820251809058,
-33.5080100112351));
#35759=CARTESIAN_POINT('Ctrl Pts',(-10.3199373397262,-3.74469501429227,
-29.2334176019375));
#35760=CARTESIAN_POINT('Ctrl Pts',(-10.5571010912029,-3.72710099262819,
-24.836399911188));
#35761=CARTESIAN_POINT('Ctrl Pts',(-10.2751885578156,-3.7392015362719,-21.024174995613));
#35762=CARTESIAN_POINT('Ctrl Pts',(-9.75173749052255,-3.76629674044718,
-18.4808048167157));
#35763=CARTESIAN_POINT('Ctrl Pts',(-9.29309014227641,-3.79028538091932,
-16.8158973741638));
#35764=CARTESIAN_POINT('Ctrl Pts',(-9.17528674009693,-3.79646095010219,
-16.4203194311401));
#35765=CARTESIAN_POINT('Ctrl Pts',(-9.04991979836604,-3.80305340259771,
-16.0287845536983));
#35766=CARTESIAN_POINT('Ctrl Pts',(7.478964497047,-4.78145508078572,-52.8766677431764));
#35767=CARTESIAN_POINT('Ctrl Pts',(7.11064672563727,-4.77682808742727,-52.7108751022984));
#35768=CARTESIAN_POINT('Ctrl Pts',(6.74418835556891,-4.7717826224726,-52.5373229559984));
#35769=CARTESIAN_POINT('Ctrl Pts',(5.18925364106368,-4.74834091216943,-51.7634436186052));
#35770=CARTESIAN_POINT('Ctrl Pts',(2.914623657922,-4.70381966688121,-50.4428290878201));
#35771=CARTESIAN_POINT('Ctrl Pts',(-0.158642874478715,-4.61828583278682,
-48.0954812155703));
#35772=CARTESIAN_POINT('Ctrl Pts',(-3.32668125548832,-4.50515190400754,
-44.9765610052481));
#35773=CARTESIAN_POINT('Ctrl Pts',(-5.9452007299524,-4.38613315046716,-41.4412978481233));
#35774=CARTESIAN_POINT('Ctrl Pts',(-7.97314324858038,-4.27662792828432,
-37.5786495133028));
#35775=CARTESIAN_POINT('Ctrl Pts',(-9.50703969681092,-4.18197237106197,
-33.5016851686292));
#35776=CARTESIAN_POINT('Ctrl Pts',(-10.3965461370179,-4.11421750462538,
-29.2163430123597));
#35777=CARTESIAN_POINT('Ctrl Pts',(-10.6018933961317,-4.08262421860679,
-24.8119552227925));
#35778=CARTESIAN_POINT('Ctrl Pts',(-10.2907910363082,-4.0828488851085,-20.9959306432894));
#35779=CARTESIAN_POINT('Ctrl Pts',(-9.74665866616106,-4.10207414795096,
-18.4518304865827));
#35780=CARTESIAN_POINT('Ctrl Pts',(-9.27403000727624,-4.12088738197538,
-16.7870776721948));
#35781=CARTESIAN_POINT('Ctrl Pts',(-9.15288357365941,-4.12583098108427,
-16.3916291076865));
#35782=CARTESIAN_POINT('Ctrl Pts',(-9.0241874000593,-4.13120272145022,-16.0003140988939));
#35783=CARTESIAN_POINT('Ctrl Pts',(29.890987486445,20.7105311502984,-36.1080966928895));
#35784=CARTESIAN_POINT('Ctrl Pts',(24.8085647057379,20.5483438544848,-35.0888701401329));
#35785=CARTESIAN_POINT('Ctrl Pts',(19.9373459642322,20.4520245495079,-33.0660880724366));
#35786=CARTESIAN_POINT('Ctrl Pts',(11.2454199314767,20.3052748660675,-27.4198879717431));
#35787=CARTESIAN_POINT('Ctrl Pts',(7.42198356668275,20.248474007324,-23.7979876220315));
#35788=CARTESIAN_POINT('Ctrl Pts',(4.42502927770989,20.1925493450898,-19.5734565969181));
#35789=CARTESIAN_POINT('Ctrl Pts',(-0.621425836154269,-3.27137100779394,
-46.8708764744697));
#35790=CARTESIAN_POINT('Ctrl Pts',(-1.19192002758132,-3.25992112656234,
-46.3438042435511));
#35791=CARTESIAN_POINT('Ctrl Pts',(-1.74006508034292,-3.24789096764871,
-45.7971167502074));
#35792=CARTESIAN_POINT('Ctrl Pts',(-2.26512505204463,-3.23555894384663,
-45.2323405814156));
#35793=CARTESIAN_POINT('Ctrl Pts',(-3.55101548575753,-3.2053573815679,-43.8491837768993));
#35794=CARTESIAN_POINT('Ctrl Pts',(-4.69844665488631,-3.1733453434745,-42.3575352047323));
#35795=CARTESIAN_POINT('Ctrl Pts',(-5.69672404631823,-3.14345008158505,
-40.7799123033163));
#35796=CARTESIAN_POINT('Ctrl Pts',(-6.36224234103277,-3.12351990598108,
-39.7281636490199));
#35797=CARTESIAN_POINT('Ctrl Pts',(-6.96147006117184,-3.10453051989494,
-38.6382041778315));
#35798=CARTESIAN_POINT('Ctrl Pts',(-7.49127781852105,-3.08752071373526,
-37.5167253952501));
#35799=CARTESIAN_POINT('Ctrl Pts',(-8.02108557559295,-3.07051090758448,
-36.3952466132557));
#35800=CARTESIAN_POINT('Ctrl Pts',(-8.48147336995429,-3.0554806813514,-35.2422485198971));
#35801=CARTESIAN_POINT('Ctrl Pts',(-8.86932876672715,-3.04339100491456,
-34.0644287179805));
#35802=CARTESIAN_POINT('Ctrl Pts',(-9.45111186116346,-3.02525649028182,
-32.2976990173011));
#35803=CARTESIAN_POINT('Ctrl Pts',(-9.86969706149374,-3.01373821257335,
-30.4751204725295));
#35804=CARTESIAN_POINT('Ctrl Pts',(-10.1146971067807,-3.01128625574909,
-28.6193144325686));
#35805=CARTESIAN_POINT('Ctrl Pts',(-10.2780304699219,-3.00965161787009,
-27.382110408833));
#35806=CARTESIAN_POINT('Ctrl Pts',(-10.3642148756369,-3.01204645592803,
-26.1301386094594));
#35807=CARTESIAN_POINT('Ctrl Pts',(-10.3702000810198,-3.01891855380822,
-24.8700965047755));
#35808=CARTESIAN_POINT('Ctrl Pts',(-10.376185285685,-3.02579065086441,-23.6100545511774));
#35809=CARTESIAN_POINT('Ctrl Pts',(-10.3019713092703,-3.03714000665748,
-22.3419422941696));
#35810=CARTESIAN_POINT('Ctrl Pts',(-10.1445181071464,-3.05321938564873,
-21.0724462245572));
#35811=CARTESIAN_POINT('Ctrl Pts',(-10.0796369494723,-3.05984515577954,
-20.5493296823207));
#35812=CARTESIAN_POINT('Ctrl Pts',(-10.0006218827985,-3.06727406915267,
-20.0259781834012));
#35813=CARTESIAN_POINT('Ctrl Pts',(-9.90726126923415,-3.07550335254719,
-19.5028585426849));
#35814=CARTESIAN_POINT('Ctrl Pts',(7.33894778785658,-4.68328060676847,-52.9495146826653));
#35815=CARTESIAN_POINT('Ctrl Pts',(6.96962866947374,-4.67927906663786,-52.7827309003488));
#35816=CARTESIAN_POINT('Ctrl Pts',(6.60219995041845,-4.67486342687383,-52.6081308809317));
#35817=CARTESIAN_POINT('Ctrl Pts',(5.04785466086252,-4.65418501649615,-51.831828678971));
#35818=CARTESIAN_POINT('Ctrl Pts',(2.77634573789732,-4.61395560865182,-50.5086100724079));
#35819=CARTESIAN_POINT('Ctrl Pts',(-0.292045807321255,-4.53496565777432,
-48.1574762822767));
#35820=CARTESIAN_POINT('Ctrl Pts',(-3.45417942420346,-4.42959393838223,
-45.034302216954));
#35821=CARTESIAN_POINT('Ctrl Pts',(-6.06653279283,-4.31850354734918,-41.495020322408));
#35822=CARTESIAN_POINT('Ctrl Pts',(-8.08805877753573,-4.2170896233612,-37.6286344119132));
#35823=CARTESIAN_POINT('Ctrl Pts',(-9.61533213266668,-4.13063759391767,
-33.5481785074831));
#35824=CARTESIAN_POINT('Ctrl Pts',(-10.4979663275097,-4.07121155600733,
-29.2596885385511));
#35825=CARTESIAN_POINT('Ctrl Pts',(-10.6962016209548,-4.04803120464602,
-24.8525448652187));
#35826=CARTESIAN_POINT('Ctrl Pts',(-10.3788445940736,-4.055480889925,-21.0344500928801));
#35827=CARTESIAN_POINT('Ctrl Pts',(-9.83045198196616,-4.07952578289679,
-18.4891787747176));
#35828=CARTESIAN_POINT('Ctrl Pts',(-9.35438474400941,-4.10152925776619,
-16.8215905800271));
#35829=CARTESIAN_POINT('Ctrl Pts',(-9.23187396168105,-4.1072571624472,-16.4239003651629));
#35830=CARTESIAN_POINT('Ctrl Pts',(-9.10174148617946,-4.11341014061892,
-16.030408965445));
#35831=CARTESIAN_POINT('Ctrl Pts',(7.59886962875189,-4.24009445412503,-52.8204795434402));
#35832=CARTESIAN_POINT('Ctrl Pts',(7.22880440070895,-4.23725223817857,-52.6558021234907));
#35833=CARTESIAN_POINT('Ctrl Pts',(6.86057612481852,-4.23400446880359,-52.4833150943556));
#35834=CARTESIAN_POINT('Ctrl Pts',(5.30259606036827,-4.21832863439708,-51.7160246632286));
#35835=CARTESIAN_POINT('Ctrl Pts',(3.02458111694869,-4.18572164472913,-50.4063763572215));
#35836=CARTESIAN_POINT('Ctrl Pts',(-0.0563369732475343,-4.11799618192084,
-48.0747261660015));
#35837=CARTESIAN_POINT('Ctrl Pts',(-3.2362291943784,-4.02550335874969,-44.9730096590617));
#35838=CARTESIAN_POINT('Ctrl Pts',(-5.87015686281,-3.92690475481451,-41.4532657427213));
#35839=CARTESIAN_POINT('Ctrl Pts',(-7.91688453516029,-3.83755718932749,
-37.6040122637326));
#35840=CARTESIAN_POINT('Ctrl Pts',(-9.4721479569566,-3.76285616468038,-33.5385007226496));
#35841=CARTESIAN_POINT('Ctrl Pts',(-10.3861063459171,-3.71481495977278,
-29.2619011417045));
#35842=CARTESIAN_POINT('Ctrl Pts',(-10.6187640483301,-3.70275434803773,
-24.863123274024));
#35843=CARTESIAN_POINT('Ctrl Pts',(-10.3329026491843,-3.71962751323487,
-21.0495715365539));
#35844=CARTESIAN_POINT('Ctrl Pts',(-9.80676713372355,-3.74992063397164,
-18.5054458515168));
#35845=CARTESIAN_POINT('Ctrl Pts',(-9.3457471942309,-3.77604797989279,-16.8379483906474));
#35846=CARTESIAN_POINT('Ctrl Pts',(-9.22684691101437,-3.78276245762616,
-16.4401792867344));
#35847=CARTESIAN_POINT('Ctrl Pts',(-9.10030801587574,-3.78989370687861,
-16.0465102000721));
#35848=CARTESIAN_POINT('Ctrl Pts',(7.86406357984036,-3.80075287541765,-52.6888944549166));
#35849=CARTESIAN_POINT('Ctrl Pts',(7.49323426140441,-3.79905339336963,-52.5263353523576));
#35850=CARTESIAN_POINT('Ctrl Pts',(7.12418814332937,-3.79695621683146,-52.3559727587527));
#35851=CARTESIAN_POINT('Ctrl Pts',(5.56249423822884,-3.78620663871065,-51.5977405820072));
#35852=CARTESIAN_POINT('Ctrl Pts',(3.27786174290937,-3.76109400159902,-50.3017259640724));
#35853=CARTESIAN_POINT('Ctrl Pts',(0.184278354359802,-3.70440674399875,
-47.9896355736996));
#35854=CARTESIAN_POINT('Ctrl Pts',(-3.01350108687011,-3.62448835210827,
-44.9094470052877));
#35855=CARTESIAN_POINT('Ctrl Pts',(-5.66909257188744,-3.53802316526296,
-41.4092957476385));
#35856=CARTESIAN_POINT('Ctrl Pts',(-7.74107979291541,-3.46032715355504,
-37.5772209009879));
#35857=CARTESIAN_POINT('Ctrl Pts',(-9.32437443940699,-3.39690914788247,
-33.5266991900448));
#35858=CARTESIAN_POINT('Ctrl Pts',(-10.2696918840725,-3.35971861494906,
-29.2620368626687));
#35859=CARTESIAN_POINT('Ctrl Pts',(-10.5368248659369,-3.35817927654809,
-24.8716740420261));
#35860=CARTESIAN_POINT('Ctrl Pts',(-10.2825404940654,-3.38391914529348,
-21.0627083330555));
#35861=CARTESIAN_POINT('Ctrl Pts',(-9.77874494355101,-3.42007079724739,
-18.5197526990839));
#35862=CARTESIAN_POINT('Ctrl Pts',(-9.33284089999827,-3.45006162272336,
-16.8523595458168));
#35863=CARTESIAN_POINT('Ctrl Pts',(-9.2175692452616,-3.45770043113048,-16.4545137405203));
#35864=CARTESIAN_POINT('Ctrl Pts',(-9.09464351807648,-3.46574819271174,
-16.0606680874987));
#35865=CARTESIAN_POINT('Ctrl Pts',(8.8177622376813,-2.2653457359543,-52.2159314161534));
#35866=CARTESIAN_POINT('Ctrl Pts',(8.44417111226431,-2.26761569662348,-52.0608800900341));
#35867=CARTESIAN_POINT('Ctrl Pts',(8.072174006773,-2.26951335386862,-51.8980459063678));
#35868=CARTESIAN_POINT('Ctrl Pts',(6.49710028208358,-2.27586002752392,-51.1719095459996));
#35869=CARTESIAN_POINT('Ctrl Pts',(4.18873282943485,-2.27671432942662,-49.924179739321));
#35870=CARTESIAN_POINT('Ctrl Pts',(1.04999287472117,-2.25814179129592,-47.6813106456907));
#35871=CARTESIAN_POINT('Ctrl Pts',(-2.21131802312341,-2.2214798205824,-44.6772615529364));
#35872=CARTESIAN_POINT('Ctrl Pts',(-4.94361513155905,-2.17652897108851,
-41.2463728727339));
#35873=CARTESIAN_POINT('Ctrl Pts',(-7.10487029831094,-2.13845241575724,
-37.4750215186926));
#35874=CARTESIAN_POINT('Ctrl Pts',(-8.78714219447284,-2.11316923258448,
-33.4775050972905));
#35875=CARTESIAN_POINT('Ctrl Pts',(-9.84314207841108,-2.11235831802136,
-29.2550930390527));
#35876=CARTESIAN_POINT('Ctrl Pts',(-10.2320008554077,-2.14581153060268,
-24.8945741017885));
#35877=CARTESIAN_POINT('Ctrl Pts',(-10.0893195591215,-2.20085463389179,
-21.1019331266132));
#35878=CARTESIAN_POINT('Ctrl Pts',(-9.66456637968633,-2.25628908058851,
-18.5631943298776));
#35879=CARTESIAN_POINT('Ctrl Pts',(-9.27218786611045,-2.29898278275007,
-16.896221484846));
#35880=CARTESIAN_POINT('Ctrl Pts',(-9.16977542161468,-2.30966173471912,
-16.4981148423604));
#35881=CARTESIAN_POINT('Ctrl Pts',(-9.05966377546826,-2.32072459453129,
-16.1036530445452));
#35882=CARTESIAN_POINT('Ctrl Pts',(10.6092118097825,0.42091842584111,-51.328617643362));
#35883=CARTESIAN_POINT('Ctrl Pts',(10.23048025638,0.412015546281074,-51.1871145970464));
#35884=CARTESIAN_POINT('Ctrl Pts',(9.8530086134927,0.403442573942463,-51.0378687887964));
#35885=CARTESIAN_POINT('Ctrl Pts',(8.25318533936325,0.368526239150617,-50.3696782505686));
#35886=CARTESIAN_POINT('Ctrl Pts',(5.90113204983879,0.324281374370589,-49.2091135002706));
#35887=CARTESIAN_POINT('Ctrl Pts',(2.67983263917123,0.279215865745994,-47.0911873404082));
#35888=CARTESIAN_POINT('Ctrl Pts',(-0.697133045717137,0.243759038204317,
-44.2245576034823));
#35889=CARTESIAN_POINT('Ctrl Pts',(-3.56856160174788,0.21967725703067,-40.9186756979785));
#35890=CARTESIAN_POINT('Ctrl Pts',(-5.89133125107194,0.192114722189047,
-37.2569397966404));
#35891=CARTESIAN_POINT('Ctrl Pts',(-7.75241625781529,0.154437491851918,
-33.3551369283939));
#35892=CARTESIAN_POINT('Ctrl Pts',(-9.00808293107892,0.0954817696064694,
-29.2090777884208));
#35893=CARTESIAN_POINT('Ctrl Pts',(-9.61628317437987,0.0048363712043943,
-24.9025945312891));
#35894=CARTESIAN_POINT('Ctrl Pts',(-9.67455583695819,-0.0979118428630517,
-21.1396270961213));
#35895=CARTESIAN_POINT('Ctrl Pts',(-9.39204048671938,-0.184631554593919,
-18.6086884842893));
#35896=CARTESIAN_POINT('Ctrl Pts',(-9.0959566327371,-0.247909792323189,
-16.9426180555065));
#35897=CARTESIAN_POINT('Ctrl Pts',(-9.01670666115945,-0.263520166061751,
-16.5440824447891));
#35898=CARTESIAN_POINT('Ctrl Pts',(-8.9297037981404,-0.279478515480188,
-16.1485563076619));
#35899=CARTESIAN_POINT('Ctrl Pts',(13.3916902429157,3.93922736422659,-49.9537287467088));
#35900=CARTESIAN_POINT('Ctrl Pts',(13.0052118686551,3.92273017306588,-49.8315070830361));
#35901=CARTESIAN_POINT('Ctrl Pts',(12.6195329570733,3.90651491483579,-49.7016027937567));
#35902=CARTESIAN_POINT('Ctrl Pts',(10.9827808399633,3.83888692720806,-49.115910516525));
#35903=CARTESIAN_POINT('Ctrl Pts',(8.56616880546154,3.74496038387833,-48.0794149501526));
#35904=CARTESIAN_POINT('Ctrl Pts',(5.22446217876673,3.6271896762232,-46.1392640327796));
#35905=CARTESIAN_POINT('Ctrl Pts',(1.68027620871272,3.50969140214063,-43.4681077992377));
#35906=CARTESIAN_POINT('Ctrl Pts',(-1.39083143471865,3.40771510315772,-40.3400067193343));
#35907=CARTESIAN_POINT('Ctrl Pts',(-3.94420957473155,3.30695483103527,-36.8341782812466));
#35908=CARTESIAN_POINT('Ctrl Pts',(-6.05979964528246,3.1998573133211,-33.0685560561463));
#35909=CARTESIAN_POINT('Ctrl Pts',(-7.59877096111654,3.07607789704229,-29.0312385925458));
#35910=CARTESIAN_POINT('Ctrl Pts',(-8.51743941326012,2.92448144596071,-24.801916525237));
#35911=CARTESIAN_POINT('Ctrl Pts',(-8.85970116110627,2.77158317941627,-21.0815574802459));
#35912=CARTESIAN_POINT('Ctrl Pts',(-8.77792663629936,2.65236568914073,-18.562097581594));
#35913=CARTESIAN_POINT('Ctrl Pts',(-8.61766417553023,2.56779645721963,-16.8976093356764));
#35914=CARTESIAN_POINT('Ctrl Pts',(-8.57114352238457,2.54707902977605,-16.4985644453621));
#35915=CARTESIAN_POINT('Ctrl Pts',(-8.51685227096455,2.52604544176493,-16.1016514020163));
#35916=CARTESIAN_POINT('Ctrl Pts',(16.8590239124754,7.64857049485316,-48.2430713861362));
#35917=CARTESIAN_POINT('Ctrl Pts',(16.4632196116715,7.62538079009264,-48.1431494592939));
#35918=CARTESIAN_POINT('Ctrl Pts',(16.0677119033701,7.6024320797305,-48.0356205741132));
#35919=CARTESIAN_POINT('Ctrl Pts',(14.3869451174134,7.50598047950645,-47.5454025434781));
#35920=CARTESIAN_POINT('Ctrl Pts',(11.8938724168184,7.36825978906471,-46.6524594301012));
#35921=CARTESIAN_POINT('Ctrl Pts',(8.41082254202169,7.18657585481396,-44.9179175569957));
#35922=CARTESIAN_POINT('Ctrl Pts',(4.67151228739915,6.99739878870591,-42.4727538029817));
#35923=CARTESIAN_POINT('Ctrl Pts',(1.3686225793903,6.82819742189185,-39.5500970265053));
#35924=CARTESIAN_POINT('Ctrl Pts',(-1.45143853585427,6.66543158101024,-36.2243659095515));
#35925=CARTESIAN_POINT('Ctrl Pts',(-3.86066265880184,6.50060855796851,-32.6160075343978));
#35926=CARTESIAN_POINT('Ctrl Pts',(-5.72573184926258,6.32441606849526,-28.7042233083674));
#35927=CARTESIAN_POINT('Ctrl Pts',(-7.00109565032812,6.12505774886043,-24.5639570327674));
#35928=CARTESIAN_POINT('Ctrl Pts',(-7.66922039578791,5.93384517916791,-20.8927712940131));
#35929=CARTESIAN_POINT('Ctrl Pts',(-7.81753482922903,5.79035915091665,-18.3865669077403));
#35930=CARTESIAN_POINT('Ctrl Pts',(-7.81287491810413,5.69001969995687,-16.7239169361633));
#35931=CARTESIAN_POINT('Ctrl Pts',(-7.80393120495686,5.66551509710643,-16.3243468486962));
#35932=CARTESIAN_POINT('Ctrl Pts',(-7.78727676373068,5.64071489355821,-15.9259510977805));
#35933=CARTESIAN_POINT('Ctrl Pts',(20.1260836878443,10.6050661536892,-46.632830625662));
#35934=CARTESIAN_POINT('Ctrl Pts',(19.7218052839872,10.5777689837161,-46.5526052118606));
#35935=CARTESIAN_POINT('Ctrl Pts',(19.3174080381398,10.5506896266998,-46.4648422656697));
#35936=CARTESIAN_POINT('Ctrl Pts',(17.5970044237572,10.4365567481294,-46.058983429135));
#35937=CARTESIAN_POINT('Ctrl Pts',(15.0353807990198,10.2719415070743,-45.2928545013636));
#35938=CARTESIAN_POINT('Ctrl Pts',(11.4264127966159,10.0511774947007,-43.7398720626974));
#35939=CARTESIAN_POINT('Ctrl Pts',(7.51403185573689,9.81863871620139,-41.4941801425206));
#35940=CARTESIAN_POINT('Ctrl Pts',(4.00635829739916,9.60967367489776,-38.7527503735285));
#35941=CARTESIAN_POINT('Ctrl Pts',(0.951351346209991,9.41153176383594,-35.5857793543118));
#35942=CARTESIAN_POINT('Ctrl Pts',(-1.7160947488882,9.21500541081661,-32.1159600367897));
#35943=CARTESIAN_POINT('Ctrl Pts',(-3.86740386355494,9.01175979868378,-28.314634950641));
#35944=CARTESIAN_POINT('Ctrl Pts',(-5.45538785555814,8.78956564702969,-24.2525762590724));
#35945=CARTESIAN_POINT('Ctrl Pts',(-6.40881146344196,8.58124477590158,-20.6244241991297));
#35946=CARTESIAN_POINT('Ctrl Pts',(-6.75838644584931,8.42762540105217,-18.1296613415041));
#35947=CARTESIAN_POINT('Ctrl Pts',(-6.88977562100234,8.32086564673385,-16.4684620494197));
#35948=CARTESIAN_POINT('Ctrl Pts',(-6.91374446804093,8.29482075310626,-16.0684584954673));
#35949=CARTESIAN_POINT('Ctrl Pts',(-6.9301128982961,8.26849188852043,-15.6688519964121));
#35950=CARTESIAN_POINT('Ctrl Pts',(24.0944858944396,13.6252616883324,-44.6776818510423));
#35951=CARTESIAN_POINT('Ctrl Pts',(23.6803406585357,13.5952855444977,-44.6200952707445));
#35952=CARTESIAN_POINT('Ctrl Pts',(23.2656345591204,13.5655149131873,-44.555050002304));
#35953=CARTESIAN_POINT('Ctrl Pts',(21.4994400484191,13.4398628522405,-44.2461531702864));
#35954=CARTESIAN_POINT('Ctrl Pts',(18.8587889372672,13.2576618204372,-43.6257566226496));
#35955=CARTESIAN_POINT('Ctrl Pts',(15.1051146705744,13.0115743729063,-42.2813283108309));
#35956=CARTESIAN_POINT('Ctrl Pts',(10.9942878557702,12.751644575675,-40.2646477779735));
#35957=CARTESIAN_POINT('Ctrl Pts',(7.25229871579309,12.5189796899122,-37.7311156744984));
#35958=CARTESIAN_POINT('Ctrl Pts',(3.92890521817145,12.301865256328,-34.7460690231871));
#35959=CARTESIAN_POINT('Ctrl Pts',(0.96680269920358,12.0904144587841,-31.4348095438096));
#35960=CARTESIAN_POINT('Ctrl Pts',(-1.51075548194581,11.8774764455751,-27.7596131452014));
#35961=CARTESIAN_POINT('Ctrl Pts',(-3.45469180565196,11.6504923923572,-23.7864536540749));
#35962=CARTESIAN_POINT('Ctrl Pts',(-4.73272035107421,11.4410171343385,-20.2068032096485));
#35963=CARTESIAN_POINT('Ctrl Pts',(-5.31112734453827,11.2882220371981,-17.7244763646882));
#35964=CARTESIAN_POINT('Ctrl Pts',(-5.59715265714841,11.1823584691134,-16.0644493054574));
#35965=CARTESIAN_POINT('Ctrl Pts',(-5.65857325334263,11.1565388193505,-15.6639265472815));
#35966=CARTESIAN_POINT('Ctrl Pts',(-5.71256297075867,11.1304479812224,-15.2630020264613));
#35967=CARTESIAN_POINT('Ctrl Pts',(27.7524631280282,15.9398275064074,-42.8755062279286));
#35968=CARTESIAN_POINT('Ctrl Pts',(27.3296292380419,15.9092719019138,-42.8377973240549));
#35969=CARTESIAN_POINT('Ctrl Pts',(26.9058773118923,15.8789225535602,-42.7926942326871));
#35970=CARTESIAN_POINT('Ctrl Pts',(25.0996377363701,15.7507918597713,-42.5689002608853));
#35971=CARTESIAN_POINT('Ctrl Pts',(22.3899228472107,15.5646999212503,-42.076390030712));
#35972=CARTESIAN_POINT('Ctrl Pts',(18.5099328809061,15.3133344724918,-40.9148965646952));
#35973=CARTESIAN_POINT('Ctrl Pts',(14.2260415512262,15.0487502016962,-39.0989822697625));
#35974=CARTESIAN_POINT('Ctrl Pts',(10.2799024562032,14.8142492774957,-36.7475381195557));
#35975=CARTESIAN_POINT('Ctrl Pts',(6.72287574105206,14.5991383033468,-33.9216147039428));
#35976=CARTESIAN_POINT('Ctrl Pts',(3.50443021549915,14.3930646018661,-30.7488263968559));
#35977=CARTESIAN_POINT('Ctrl Pts',(0.743246967286701,14.1899609567462,-27.1834418577565));
#35978=CARTESIAN_POINT('Ctrl Pts',(-1.50992084988385,13.977122935371,-23.2872040240248));
#35979=CARTESIAN_POINT('Ctrl Pts',(-3.06979700167895,13.7824369346935,-19.7490208233323));
#35980=CARTESIAN_POINT('Ctrl Pts',(-3.84678924988332,13.6409944051188,-17.2767648669773));
#35981=CARTESIAN_POINT('Ctrl Pts',(-4.26697517747692,13.5429643472183,-15.6171729631503));
#35982=CARTESIAN_POINT('Ctrl Pts',(-4.36090283399386,13.5190447294408,-15.2161420151018));
#35983=CARTESIAN_POINT('Ctrl Pts',(-4.44756309121091,13.4948677704672,-14.8140961072926));
#35984=CARTESIAN_POINT('Ctrl Pts',(32.1092038605354,18.188947172369,-40.7280566168821));
#35985=CARTESIAN_POINT('Ctrl Pts',(31.6765553815004,18.1597316481657,-40.7130636737339));
#35986=CARTESIAN_POINT('Ctrl Pts',(31.2426152350551,18.1307342364494,-40.6907406131988));
#35987=CARTESIAN_POINT('Ctrl Pts',(29.3914008267549,18.0083786966032,-40.5641260176311));
#35988=CARTESIAN_POINT('Ctrl Pts',(26.6040098369721,17.830846834045,-40.2176280285863));
#35989=CARTESIAN_POINT('Ctrl Pts',(22.5816971333687,17.5925027676131,-39.2649049617731));
#35990=CARTESIAN_POINT('Ctrl Pts',(18.1026055111639,17.3443426911773,-37.6779673237996));
#35991=CARTESIAN_POINT('Ctrl Pts',(13.9260329063887,17.1289494695207,-35.5339680565631));
#35992=CARTESIAN_POINT('Ctrl Pts',(10.1052117066657,16.9369213116231,-32.8890131586941));
#35993=CARTESIAN_POINT('Ctrl Pts',(6.59730531312819,16.7575317657622,-29.8733821949946));
#35994=CARTESIAN_POINT('Ctrl Pts',(3.5158662876463,16.5859876106103,-26.4321103440903));
#35995=CARTESIAN_POINT('Ctrl Pts',(0.913599505363284,16.4095763329362,-22.6220597413816));
#35996=CARTESIAN_POINT('Ctrl Pts',(-0.964389552830138,16.2491906636996,
-19.1295387897028));
#35997=CARTESIAN_POINT('Ctrl Pts',(-1.9654556525298,16.1323920433636,-16.6674580294462));
#35998=CARTESIAN_POINT('Ctrl Pts',(-2.53699602967554,16.0510402241362,-15.007420086541));
#35999=CARTESIAN_POINT('Ctrl Pts',(-2.66758615191287,16.0311583490605,-14.60568241689));
#36000=CARTESIAN_POINT('Ctrl Pts',(-2.79108562724462,16.01103806515,-14.2023282308814));
#36001=CARTESIAN_POINT('Ctrl Pts',(36.0546359053991,19.7983627848149,-38.7818450804867));
#36002=CARTESIAN_POINT('Ctrl Pts',(35.6136081827865,19.7720645135703,-38.7866824550858));
#36003=CARTESIAN_POINT('Ctrl Pts',(35.1709903510993,19.7460021313493,-38.7842339544363));
#36004=CARTESIAN_POINT('Ctrl Pts',(33.2815581289281,19.6361820466171,-38.742359341364));
#36005=CARTESIAN_POINT('Ctrl Pts',(30.4279662779038,19.4774394485581,-38.5231664068375));
#36006=CARTESIAN_POINT('Ctrl Pts',(26.2838812573179,19.2670183310104,-37.7523847452164));
#36007=CARTESIAN_POINT('Ctrl Pts',(21.6373652569733,19.0520629838802,-36.3648646999831));
#36008=CARTESIAN_POINT('Ctrl Pts',(17.2627637487776,18.8717166252608,-34.4013101103432));
#36009=CARTESIAN_POINT('Ctrl Pts',(13.2149882844746,18.7178122962125,-31.9134568102013));
#36010=CARTESIAN_POINT('Ctrl Pts',(9.45790253167546,18.5794411422907,-29.0339285444168));
#36011=CARTESIAN_POINT('Ctrl Pts',(6.10065537573886,18.4529446490623,-25.6996110869408));
#36012=CARTESIAN_POINT('Ctrl Pts',(3.19769760622167,18.3257380682571,-21.9630515161149));
#36013=CARTESIAN_POINT('Ctrl Pts',(1.04570997608589,18.2102139945187,-18.5086252116051));
#36014=CARTESIAN_POINT('Ctrl Pts',(-0.148334551971419,18.1249152482566,
-16.0540528873188));
#36015=CARTESIAN_POINT('Ctrl Pts',(-0.850211959005697,18.064727637235,-14.392650263373));
#36016=CARTESIAN_POINT('Ctrl Pts',(-1.01234491068815,18.0499634327475,-13.9901402067394));
#36017=CARTESIAN_POINT('Ctrl Pts',(-1.16751365266792,18.0349776243875,-13.5855669779328));
#36018=CARTESIAN_POINT('Ctrl Pts',(38.9437130531413,20.6836496418694,-37.3550102934179));
#36019=CARTESIAN_POINT('Ctrl Pts',(38.4969620505322,20.6606519170286,-37.3739256635358));
#36020=CARTESIAN_POINT('Ctrl Pts',(38.0484242481362,20.6379063239872,-37.3855784628576));
#36021=CARTESIAN_POINT('Ctrl Pts',(36.1329514022312,20.5422448076096,-37.4037961231016));
#36022=CARTESIAN_POINT('Ctrl Pts',(33.2340079962508,20.4047755971079,-37.2748703197067));
#36023=CARTESIAN_POINT('Ctrl Pts',(29.0058954113699,20.225761668211,-36.6330394337848));
#36024=CARTESIAN_POINT('Ctrl Pts',(24.243314845652,20.0475517349526,-35.3867546793722));
#36025=CARTESIAN_POINT('Ctrl Pts',(19.7309119375686,19.9048724048602,-33.550821780949));
#36026=CARTESIAN_POINT('Ctrl Pts',(15.5248315097876,19.790507905872,-31.1738206489958));
#36027=CARTESIAN_POINT('Ctrl Pts',(11.593709050744,19.6935273080542,-28.3900502035695));
#36028=CARTESIAN_POINT('Ctrl Pts',(8.04360552628351,19.6110850660289,-25.130528158443));
#36029=CARTESIAN_POINT('Ctrl Pts',(4.93025190736926,19.530779076001,-21.4446834603861));
#36030=CARTESIAN_POINT('Ctrl Pts',(2.58648434761514,19.4573327991495,-18.0158038661496));
#36031=CARTESIAN_POINT('Ctrl Pts',(1.25734840204799,19.4012238336331,-15.5653813052934));
#36032=CARTESIAN_POINT('Ctrl Pts',(0.46423054638623,19.3605693891818,-13.9021664678085));
#36033=CARTESIAN_POINT('Ctrl Pts',(0.280042164317415,19.3505226070412,-13.4989464907574));
#36034=CARTESIAN_POINT('Ctrl Pts',(0.10275343541301,19.3402634731691,-13.0933876689219));
#36035=CARTESIAN_POINT('Ctrl Pts',(40.5688973540866,21.117312799858,-36.551901496451));
#36036=CARTESIAN_POINT('Ctrl Pts',(40.1190235321024,21.0964267127388,-36.5786509976099));
#36037=CARTESIAN_POINT('Ctrl Pts',(39.66725798273,21.0758020890032,-36.5981477349547));
#36038=CARTESIAN_POINT('Ctrl Pts',(37.737597636275,20.9891913310095,-36.6497793174299));
#36039=CARTESIAN_POINT('Ctrl Pts',(34.8138724138779,20.8653273744228,-36.5710441821179));
#36040=CARTESIAN_POINT('Ctrl Pts',(30.5396616708079,20.7063681300896,-36.0009003281876));
#36041=CARTESIAN_POINT('Ctrl Pts',(25.7132460636541,20.5515335415639,-34.8331079770803));
#36042=CARTESIAN_POINT('Ctrl Pts',(21.1248952553841,20.4326519806542,-33.0680590907502));
#36043=CARTESIAN_POINT('Ctrl Pts',(16.8314507574351,20.3430531321453,-30.7525636742139));
#36044=CARTESIAN_POINT('Ctrl Pts',(12.804210193334,20.2718184169426,-28.0218547905441));
#36045=CARTESIAN_POINT('Ctrl Pts',(9.14752307967792,20.2165549432469,-24.8036643499281));
#36046=CARTESIAN_POINT('Ctrl Pts',(5.91784322010844,20.164982094833,-21.145672025709));
#36047=CARTESIAN_POINT('Ctrl Pts',(3.46801805054593,20.117197691553,-17.7306313359114));
#36048=CARTESIAN_POINT('Ctrl Pts',(2.0641638961292,20.0788282397779,-15.2822216218412));
#36049=CARTESIAN_POINT('Ctrl Pts',(1.22057987406261,20.0500302875854,-13.6177868335942));
#36050=CARTESIAN_POINT('Ctrl Pts',(1.02420216661473,20.0428451797642,-13.2141323698032));
#36051=CARTESIAN_POINT('Ctrl Pts',(0.834697633919559,20.0354515632684,-12.8079971705157));
#36052=CARTESIAN_POINT('Ctrl Pts',(41.0310809778576,21.2334813897109,-36.3234534242004));
#36053=CARTESIAN_POINT('Ctrl Pts',(40.5803248224942,21.2132228077857,-36.3524241259849));
#36054=CARTESIAN_POINT('Ctrl Pts',(40.1276475607981,21.1932283095702,-36.3741443398451));
#36055=CARTESIAN_POINT('Ctrl Pts',(38.1939810821135,21.1093059289188,-36.4352454955676));
#36056=CARTESIAN_POINT('Ctrl Pts',(35.2632566089281,20.9894835119608,-36.3707324792311));
#36057=CARTESIAN_POINT('Ctrl Pts',(30.9760261741618,20.8364792943525,-35.8208951740754));
#36058=CARTESIAN_POINT('Ctrl Pts',(26.1315861185953,20.6885792302246,-34.6753271627914));
#36059=CARTESIAN_POINT('Ctrl Pts',(21.5218030653981,20.5767478260626,-32.9303346052545));
#36060=CARTESIAN_POINT('Ctrl Pts',(17.2037226950434,20.4944756050622,-30.6322254140711));
#36061=CARTESIAN_POINT('Ctrl Pts',(13.1493988567874,20.4308554028779,-27.9164985852922));
#36062=CARTESIAN_POINT('Ctrl Pts',(9.46270544626104,20.3836340081555,-24.7099515839323));
#36063=CARTESIAN_POINT('Ctrl Pts',(6.20030107714963,20.340580727313,-21.0597648792395));
#36064=CARTESIAN_POINT('Ctrl Pts',(3.72065547802652,20.3004356869138,-17.6485527564509));
#36065=CARTESIAN_POINT('Ctrl Pts',(2.295793670099,20.2673681898868,-15.200636761067));
#36066=CARTESIAN_POINT('Ctrl Pts',(1.43801852688975,20.2421246596599,-13.5357989572919));
#36067=CARTESIAN_POINT('Ctrl Pts',(1.23821496048648,20.2357981340653,-13.1320096374851));
#36068=CARTESIAN_POINT('Ctrl Pts',(1.04527883727151,20.2292648564311,-12.7257013789351));
#36069=CARTESIAN_POINT('Ctrl Pts',(41.4945844892592,21.3428689572265,-36.094304790847));
#36070=CARTESIAN_POINT('Ctrl Pts',(41.0429495192362,21.323266505305,-36.1254953689207));
#36071=CARTESIAN_POINT('Ctrl Pts',(40.5893642151814,21.303930781031,-36.1494374678826));
#36072=CARTESIAN_POINT('Ctrl Pts',(38.6517079921192,21.2228186866547,-36.2200003189353));
#36073=CARTESIAN_POINT('Ctrl Pts',(35.7140114028846,21.1072213437662,-36.1696957800508));
#36074=CARTESIAN_POINT('Ctrl Pts',(31.4138119300288,20.9604400919523,-35.6401393145224));
#36075=CARTESIAN_POINT('Ctrl Pts',(26.5514224411379,20.819779963638,-34.5167581668256));
#36076=CARTESIAN_POINT('Ctrl Pts',(21.9203087230707,20.7152993064879,-32.791775100868));
#36077=CARTESIAN_POINT('Ctrl Pts',(17.5777272210475,20.6406553883908,-30.5109957831435));
#36078=CARTESIAN_POINT('Ctrl Pts',(13.4964895293743,20.5849601975755,-27.8101859299812));
#36079=CARTESIAN_POINT('Ctrl Pts',(9.7800037342825,20.5461109852346,-24.6152063244202));
#36080=CARTESIAN_POINT('Ctrl Pts',(6.48513371352389,20.5119420676311,-20.972735385183));
#36081=CARTESIAN_POINT('Ctrl Pts',(3.97592039392024,20.4797911688045,-17.5652597461339));
#36082=CARTESIAN_POINT('Ctrl Pts',(2.53023120471821,20.4522911786996,-15.1177639611188));
#36083=CARTESIAN_POINT('Ctrl Pts',(1.65838523268764,20.4307901345004,-13.4524688277451));
#36084=CARTESIAN_POINT('Ctrl Pts',(1.45518607757715,20.4253683033402,-13.0485330144838));
#36085=CARTESIAN_POINT('Ctrl Pts',(1.25884986838775,20.4197421663948,-12.6420414452013));
#36086=CARTESIAN_POINT('Ctrl Pts',(4.81048155583834,19.9464420456703,-20.0720152820648));
#36087=CARTESIAN_POINT('Ctrl Pts',(7.81583634933486,20.0189549105364,-24.1684379665366));
#36088=CARTESIAN_POINT('Ctrl Pts',(11.6050705594528,20.0954766247834,-27.675487418123));
#36089=CARTESIAN_POINT('Ctrl Pts',(20.1650060536999,20.2752040736289,-33.1377027463891));
#36090=CARTESIAN_POINT('Ctrl Pts',(24.9348834609741,20.3824974081049,-35.0946221674948));
#36091=CARTESIAN_POINT('Ctrl Pts',(29.9069010447471,20.5529756002056,-36.0949172314264));
#36092=CARTESIAN_POINT('Ctrl Pts',(39.2217566406836,20.9435908393615,-36.8146184333826));
#36093=CARTESIAN_POINT('Ctrl Pts',(39.0665136990626,20.9358615047579,-36.8200995370388));
#36094=CARTESIAN_POINT('Ctrl Pts',(38.9112707574417,20.9281321701544,-36.825580640695));
#36095=CARTESIAN_POINT('Ctrl Pts',(38.7560278158208,20.9204028355509,-36.8310617443513));
#36096=CARTESIAN_POINT('Ctrl Pts',(23.2317336537277,20.1474693751975,-37.3791721099748));
#36097=CARTESIAN_POINT('Ctrl Pts',(7.97122258304409,20.0812550388979,-28.0681800905232));
#36098=CARTESIAN_POINT('Ctrl Pts',(1.20708100656079,19.8399463130827,-14.0975769578644));
#36099=CARTESIAN_POINT('Ctrl Pts',(39.2216742354573,20.9469886892296,-36.8146659128868));
#36100=CARTESIAN_POINT('Ctrl Pts',(39.0664294181999,20.9392720585054,-36.8201548647248));
#36101=CARTESIAN_POINT('Ctrl Pts',(38.9111846009425,20.9315554277811,-36.8256438165629));
#36102=CARTESIAN_POINT('Ctrl Pts',(38.7559397836851,20.9238387970569,-36.831132768401));
#36103=CARTESIAN_POINT('Ctrl Pts',(23.2314580579417,20.1521757246323,-37.3800279522102));
#36104=CARTESIAN_POINT('Ctrl Pts',(7.9710320114852,20.0873688943554,-28.0685857559505));
#36105=CARTESIAN_POINT('Ctrl Pts',(1.20670795938283,19.8474084919615,-14.0981560611673));
#36106=CARTESIAN_POINT('Ctrl Pts',(39.2215918302311,20.9503865390978,-36.8147133923909));
#36107=CARTESIAN_POINT('Ctrl Pts',(39.0663451373372,20.9426826122528,-36.8202101924109));
#36108=CARTESIAN_POINT('Ctrl Pts',(38.9110984444433,20.9349786854078,-36.8257069924308));
#36109=CARTESIAN_POINT('Ctrl Pts',(38.7558517515493,20.9272747585629,-36.8312037924508));
#36110=CARTESIAN_POINT('Ctrl Pts',(23.2311824621557,20.1568820740671,-37.3808837944456));
#36111=CARTESIAN_POINT('Ctrl Pts',(7.97084143992632,20.093482749813,-28.0689914213779));
#36112=CARTESIAN_POINT('Ctrl Pts',(1.20633491220488,19.8548706708402,-14.0987351644701));
#36113=CARTESIAN_POINT('Ctrl Pts',(39.2215094250049,20.9537843889659,-36.8147608718951));
#36114=CARTESIAN_POINT('Ctrl Pts',(39.0662608564745,20.9460931660003,-36.8202655200969));
#36115=CARTESIAN_POINT('Ctrl Pts',(38.911012287944,20.9384019430346,-36.8257701682987));
#36116=CARTESIAN_POINT('Ctrl Pts',(38.7557637194136,20.9307107200689,-36.8312748165005));
#36117=CARTESIAN_POINT('Ctrl Pts',(23.2309068663697,20.1615884235019,-37.3817396366809));
#36118=CARTESIAN_POINT('Ctrl Pts',(7.97065086836744,20.0995966052706,-28.0693970868052));
#36119=CARTESIAN_POINT('Ctrl Pts',(1.20596186502693,19.862332849719,-14.099314267773));
#36120=CARTESIAN_POINT('Ctrl Pts',(39.2212591820617,20.9641027630587,-36.8149050546298));
#36121=CARTESIAN_POINT('Ctrl Pts',(39.0660049177178,20.9564501184246,-36.8204335356904));
#36122=CARTESIAN_POINT('Ctrl Pts',(38.9107506533739,20.9487974737906,-36.8259620167511));
#36123=CARTESIAN_POINT('Ctrl Pts',(38.75549638903,20.9411448291565,-36.8314904978117));
#36124=CARTESIAN_POINT('Ctrl Pts',(23.2300699546376,20.1758803657488,-37.3843386038783));
#36125=CARTESIAN_POINT('Ctrl Pts',(7.97007215279367,20.1181627721728,-28.0706289857407));
#36126=CARTESIAN_POINT('Ctrl Pts',(1.20482901911385,19.8849935193208,-14.1010728518038));
#36127=CARTESIAN_POINT('Ctrl Pts',(39.2207586959266,20.9847395112521,-36.8151934199635));
#36128=CARTESIAN_POINT('Ctrl Pts',(39.0654930400387,20.9771640232786,-36.8207695667871));
#36129=CARTESIAN_POINT('Ctrl Pts',(38.9102273841508,20.9695885353052,-36.8263457136107));
#36130=CARTESIAN_POINT('Ctrl Pts',(38.754961728263,20.9620130473318,-36.8319218604343));
#36131=CARTESIAN_POINT('Ctrl Pts',(23.2283961394753,20.2044642499886,-37.3895365427941));
#36132=CARTESIAN_POINT('Ctrl Pts',(7.96891471649109,20.1552951062578,-28.0730927828742));
#36133=CARTESIAN_POINT('Ctrl Pts',(1.20256332728765,19.9303148585245,-14.1045900198654));
#36134=CARTESIAN_POINT('Ctrl Pts',(39.2200079497906,21.0156946339229,-36.815625959386));
#36135=CARTESIAN_POINT('Ctrl Pts',(39.0647252122311,21.0082348808134,-36.8212736077134));
#36136=CARTESIAN_POINT('Ctrl Pts',(38.9094424746716,21.000775127704,-36.8269212560407));
#36137=CARTESIAN_POINT('Ctrl Pts',(38.7541597371122,20.9933153745945,-36.832568904368));
#36138=CARTESIAN_POINT('Ctrl Pts',(23.2258859811651,20.2473400636495,-37.3973337371021));
#36139=CARTESIAN_POINT('Ctrl Pts',(7.96717824152021,20.2109936225946,-28.0767884392132));
#36140=CARTESIAN_POINT('Ctrl Pts',(1.19916478954841,19.9982968673298,-14.1098657719579));
#36141=CARTESIAN_POINT('Ctrl Pts',(39.2192571813942,21.0466497571015,-36.8160584875007));
#36142=CARTESIAN_POINT('Ctrl Pts',(39.0639573695833,21.0393057386868,-36.8217776411011));
#36143=CARTESIAN_POINT('Ctrl Pts',(38.9086575577724,21.0319617202721,-36.8274967947015));
#36144=CARTESIAN_POINT('Ctrl Pts',(38.7533577459615,21.0246177018574,-36.8332159483019));
#36145=CARTESIAN_POINT('Ctrl Pts',(23.223376564873,20.2902158603888,-37.4051313083389));
#36146=CARTESIAN_POINT('Ctrl Pts',(7.96544134300785,20.2666921589687,-28.0804840413609));
#36147=CARTESIAN_POINT('Ctrl Pts',(1.19576625180914,20.0662788761352,-14.1151415240503));
#36148=CARTESIAN_POINT('Ctrl Pts',(39.2187566579113,21.0672865061488,-36.8163468338515));
#36149=CARTESIAN_POINT('Ctrl Pts',(39.0634454670057,21.0600196441101,-36.8221136595425));
#36150=CARTESIAN_POINT('Ctrl Pts',(38.9081342761,21.0527527820714,-36.8278804852334));
#36151=CARTESIAN_POINT('Ctrl Pts',(38.7528230851944,21.0454859200326,-36.8336473109243));
#36152=CARTESIAN_POINT('Ctrl Pts',(23.2217039946289,20.3187997161584,-37.4103298800174));
#36153=CARTESIAN_POINT('Ctrl Pts',(7.96428319555438,20.3038245267329,-28.0829477473042));
#36154=CARTESIAN_POINT('Ctrl Pts',(1.19350055998297,20.1116002153389,-14.1186586921119));
#36155=CARTESIAN_POINT('Ctrl Pts',(39.2185063960488,21.0776048806767,-36.8164910069587));
#36156=CARTESIAN_POINT('Ctrl Pts',(39.0631895156361,21.0703765968246,-36.8222816687177));
#36157=CARTESIAN_POINT('Ctrl Pts',(38.9078726352235,21.0631483129724,-36.8280723304767));
#36158=CARTESIAN_POINT('Ctrl Pts',(38.7525557548108,21.0559200291202,-36.8338629922356));
#36159=CARTESIAN_POINT('Ctrl Pts',(23.2208677135466,20.3330916439037,-37.4129291681314));
#36160=CARTESIAN_POINT('Ctrl Pts',(7.96370411918316,20.3223907107576,-28.0841795997822));
#36161=CARTESIAN_POINT('Ctrl Pts',(1.19236771406988,20.1342608849406,-14.1204172761427));
#36162=CARTESIAN_POINT('Ctrl Pts',(39.2184822807631,21.0785991614118,-36.8165048995096));
#36163=CARTESIAN_POINT('Ctrl Pts',(39.0631648521084,21.0713745949617,-36.8222978581171));
#36164=CARTESIAN_POINT('Ctrl Pts',(38.9078474234537,21.0641500285117,-36.8280908167246));
#36165=CARTESIAN_POINT('Ctrl Pts',(38.752529994799,21.0569254620617,-36.833883775332));
#36166=CARTESIAN_POINT('Ctrl Pts',(23.220787129326,20.3344688170607,-37.4131796360796));
#36167=CARTESIAN_POINT('Ctrl Pts',(7.9636483192625,20.3241797521467,-28.0842983013455));
#36168=CARTESIAN_POINT('Ctrl Pts',(1.19225855279994,20.1364444718193,-14.120586733669));
#36169=CARTESIAN_POINT('Ctrl Pts',(39.2184581654775,21.0795934421468,-36.8165187920605));
#36170=CARTESIAN_POINT('Ctrl Pts',(39.0631401885807,21.0723725930989,-36.8223140475165));
#36171=CARTESIAN_POINT('Ctrl Pts',(38.9078222116839,21.0651517440511,-36.8281093029725));
#36172=CARTESIAN_POINT('Ctrl Pts',(38.7525042347871,21.0579308950032,-36.8339045584284));
#36173=CARTESIAN_POINT('Ctrl Pts',(23.2207065451054,20.3358459902176,-37.4134301040277));
#36174=CARTESIAN_POINT('Ctrl Pts',(7.96359251934184,20.3259687935359,-28.0844170029088));
#36175=CARTESIAN_POINT('Ctrl Pts',(1.19214939153001,20.1386280586979,-14.1207561911953));
#36176=CARTESIAN_POINT('Ctrl Pts',(39.2184340501919,21.0805877228818,-36.8165326846113));
#36177=CARTESIAN_POINT('Ctrl Pts',(39.063115525053,21.0733705912361,-36.8223302369158));
#36178=CARTESIAN_POINT('Ctrl Pts',(38.9077969999141,21.0661534595904,-36.8281277892204));
#36179=CARTESIAN_POINT('Ctrl Pts',(38.7524784747752,21.0589363279447,-36.8339253415249));
#36180=CARTESIAN_POINT('Ctrl Pts',(23.2206259608848,20.3372231633746,-37.4136805719759));
#36181=CARTESIAN_POINT('Ctrl Pts',(7.96353671942118,20.327757834925,-28.0845357044721));
#36182=CARTESIAN_POINT('Ctrl Pts',(1.19204023026007,20.1408116455766,-14.1209256487216));
#36183=CARTESIAN_POINT('Ctrl Pts',(54.096233416894,21.2883239772394,9.98352735473641));
#36184=CARTESIAN_POINT('Ctrl Pts',(53.8409594097646,21.2711623310641,9.61248528230055));
#36185=CARTESIAN_POINT('Ctrl Pts',(53.5788530977531,21.2542807820542,9.24441890854599));
#36186=CARTESIAN_POINT('Ctrl Pts',(52.4311812489649,21.1834525291307,7.68716578714771));
#36187=CARTESIAN_POINT('Ctrl Pts',(50.5662584013097,21.0834264338425,5.42184195082861));
#36188=CARTESIAN_POINT('Ctrl Pts',(47.4787450278816,20.9598507183575,2.3893977933402));
#36189=CARTESIAN_POINT('Ctrl Pts',(43.575989077353,20.8461335954997,-0.713114551264511));
#36190=CARTESIAN_POINT('Ctrl Pts',(39.3448124775761,20.7684839093916,-3.2603433732672));
#36191=CARTESIAN_POINT('Ctrl Pts',(34.8565666606213,20.7206230093664,-5.23576668658806));
#36192=CARTESIAN_POINT('Ctrl Pts',(30.2008472528554,20.6916936542703,-6.74506250497749));
#36193=CARTESIAN_POINT('Ctrl Pts',(25.3835553034033,20.6796111419738,-7.66097308304403));
#36194=CARTESIAN_POINT('Ctrl Pts',(20.4764910470132,20.6722203558656,-7.96784585316283));
#36195=CARTESIAN_POINT('Ctrl Pts',(16.2417385179411,20.6630225594897,-7.80630362792482));
#36196=CARTESIAN_POINT('Ctrl Pts',(13.4213391185488,20.6508204531822,-7.4110411108956));
#36197=CARTESIAN_POINT('Ctrl Pts',(11.5740620400678,20.6394053700742,-7.05498278350414));
#36198=CARTESIAN_POINT('Ctrl Pts',(11.132952210758,20.6364191357732,-6.96256671604898));
#36199=CARTESIAN_POINT('Ctrl Pts',(10.694125226444,20.6332209087108,-6.8632653171979));
#36200=CARTESIAN_POINT('Ctrl Pts',(53.9830369457162,21.2398788304839,9.46171406818988));
#36201=CARTESIAN_POINT('Ctrl Pts',(53.7266004689061,21.2217224127637,9.09271470601715));
#36202=CARTESIAN_POINT('Ctrl Pts',(53.4633475549858,21.2038412173392,8.7267144505681));
#36203=CARTESIAN_POINT('Ctrl Pts',(52.3108518161382,21.1287309618461,7.17837913463006));
#36204=CARTESIAN_POINT('Ctrl Pts',(50.4392773471876,21.0222253289507,4.92722374819142));
#36205=CARTESIAN_POINT('Ctrl Pts',(47.3441140086114,20.8890564489947,1.91734732260939));
#36206=CARTESIAN_POINT('Ctrl Pts',(43.4352890996597,20.7641817659416,-1.15756126347997));
#36207=CARTESIAN_POINT('Ctrl Pts',(39.2017861763524,20.6752847595175,-3.67591975391337));
#36208=CARTESIAN_POINT('Ctrl Pts',(34.7152142664626,20.6159219251614,-5.62169100966009));
#36209=CARTESIAN_POINT('Ctrl Pts',(30.0645001982276,20.5752144761384,-7.1009771020976));
#36210=CARTESIAN_POINT('Ctrl Pts',(25.2565486693757,20.5509334123338,-7.98675116083998));
#36211=CARTESIAN_POINT('Ctrl Pts',(20.3634163558495,20.5308579865904,-8.26383905577707));
#36212=CARTESIAN_POINT('Ctrl Pts',(16.1438739001623,20.510426256151,-8.07723388342209));
#36213=CARTESIAN_POINT('Ctrl Pts',(13.335881648162,20.4905046142392,-7.66570489790757));
#36214=CARTESIAN_POINT('Ctrl Pts',(11.4975417212571,20.4739374093561,-7.29913696623926));
#36215=CARTESIAN_POINT('Ctrl Pts',(11.0586072647004,20.469713411733,-7.2042182379738));
#36216=CARTESIAN_POINT('Ctrl Pts',(10.6219862286722,20.4652767483487,-7.10243434478152));
#36217=CARTESIAN_POINT('Ctrl Pts',(53.8697370177666,21.1822016013635,8.93970129386049));
#36218=CARTESIAN_POINT('Ctrl Pts',(53.6121351567703,21.1630886105529,8.57276400445957));
#36219=CARTESIAN_POINT('Ctrl Pts',(53.3477329763492,21.1442460408093,8.20884980300576));
#36220=CARTESIAN_POINT('Ctrl Pts',(52.1904032008889,21.0650173413637,6.66951987973133));
#36221=CARTESIAN_POINT('Ctrl Pts',(50.312164897738,20.9522796229575,4.4326664265343));
#36222=CARTESIAN_POINT('Ctrl Pts',(47.2093446045204,20.8098799445818,1.44556050267551));
#36223=CARTESIAN_POINT('Ctrl Pts',(43.2944576422004,20.6742608619688,-1.60149992344141));
#36224=CARTESIAN_POINT('Ctrl Pts',(39.0586575078325,20.5745198093833,-4.09072706669367));
#36225=CARTESIAN_POINT('Ctrl Pts',(34.5738153175261,20.5040526001987,-6.00656185447961));
#36226=CARTESIAN_POINT('Ctrl Pts',(29.9281883187936,20.4519664047462,-7.45552706604719));
#36227=CARTESIAN_POINT('Ctrl Pts',(25.1296932182711,20.4158956934967,-8.31081715048489));
#36228=CARTESIAN_POINT('Ctrl Pts',(20.250643895266,20.3835681705302,-8.55773188003308));
#36229=CARTESIAN_POINT('Ctrl Pts',(16.0464632313985,20.3523071857454,-8.34569622092367));
#36230=CARTESIAN_POINT('Ctrl Pts',(13.2509884095923,20.3249607749065,-7.91763736285362));
#36231=CARTESIAN_POINT('Ctrl Pts',(11.4216589411055,20.3034475984546,-7.5403803228002));
#36232=CARTESIAN_POINT('Ctrl Pts',(10.9849194872874,20.2980359714688,-7.44291568157701));
#36233=CARTESIAN_POINT('Ctrl Pts',(10.5505259893207,20.29241155197,-7.33860589683737));
#36234=CARTESIAN_POINT('Ctrl Pts',(53.4644633086927,20.942701117012,7.07354901688149));
#36235=CARTESIAN_POINT('Ctrl Pts',(53.2026883461185,20.9203083949833,6.71404688513704));
#36236=CARTESIAN_POINT('Ctrl Pts',(52.9341714587248,20.898168919688,6.35765679911698));
#36237=CARTESIAN_POINT('Ctrl Pts',(51.7595381232525,20.8048139743737,4.85081887924358));
#36238=CARTESIAN_POINT('Ctrl Pts',(49.857453155798,20.6706999592586,2.66554851920846));
#36239=CARTESIAN_POINT('Ctrl Pts',(46.7272593393429,20.496623371127,-0.239462178198342));
#36240=CARTESIAN_POINT('Ctrl Pts',(42.7907482839516,20.3241023157428,-3.18613007185183));
#36241=CARTESIAN_POINT('Ctrl Pts',(38.5468554926957,20.1870685788371,-5.5703146686724));
#36242=CARTESIAN_POINT('Ctrl Pts',(34.0684049418232,20.0783595881962,-7.37814069679685));
#36243=CARTESIAN_POINT('Ctrl Pts',(29.4412586748499,19.9870599496472,-8.71762346866089));
#36244=CARTESIAN_POINT('Ctrl Pts',(24.6769789007594,19.9103458023656,-9.46271295215423));
#36245=CARTESIAN_POINT('Ctrl Pts',(19.8487996392098,19.8358125374395,-9.60038699181189));
#36246=CARTESIAN_POINT('Ctrl Pts',(15.7000560750932,19.767331746443,-9.29613511960772));
#36247=CARTESIAN_POINT('Ctrl Pts',(12.9497018486459,19.7145309927478,-8.8080470657374));
#36248=CARTESIAN_POINT('Ctrl Pts',(11.1528281593933,19.6760973304852,-8.39193939128734));
#36249=CARTESIAN_POINT('Ctrl Pts',(10.724004523227,19.6666248028076,-8.28521939042578));
#36250=CARTESIAN_POINT('Ctrl Pts',(10.2976530603138,19.6569408091057,-8.17172515586503));
#36251=CARTESIAN_POINT('Ctrl Pts',(52.8863153515536,20.4780024533914,4.41539935052617));
#36252=CARTESIAN_POINT('Ctrl Pts',(52.6185716797916,20.4514551579611,4.06672732948473));
#36253=CARTESIAN_POINT('Ctrl Pts',(52.344171576181,20.4251375618498,3.72130358184864));
#36254=CARTESIAN_POINT('Ctrl Pts',(51.1448075867849,20.3138746691076,2.2618508394985));
#36255=CARTESIAN_POINT('Ctrl Pts',(49.208673544985,20.1526659052326,0.151770647364792));
#36256=CARTESIAN_POINT('Ctrl Pts',(46.0395105548711,19.938389785095,-2.63365452435864));
#36257=CARTESIAN_POINT('Ctrl Pts',(42.0723996256245,19.7189203495023,-5.434144257564));
#36258=CARTESIAN_POINT('Ctrl Pts',(37.817410701173,19.5342279169114,-7.66541815032562));
#36259=CARTESIAN_POINT('Ctrl Pts',(33.3487384781665,19.3763677050182,-9.3160029447135));
#36260=CARTESIAN_POINT('Ctrl Pts',(28.7487915843048,19.2344308170631,-10.4960634080756));
#36261=CARTESIAN_POINT('Ctrl Pts',(24.0343837367008,19.1049298841923,-11.0806082778795));
#36262=CARTESIAN_POINT('Ctrl Pts',(19.2800719812092,18.9752993129734,-11.0590103243977));
#36263=CARTESIAN_POINT('Ctrl Pts',(15.2116924680306,18.8580619466085,-10.6201973999149));
#36264=CARTESIAN_POINT('Ctrl Pts',(12.5266729066911,18.7718242877839,-10.044424156308));
#36265=CARTESIAN_POINT('Ctrl Pts',(10.7767743381542,18.7111415689428,-9.57153073773204));
#36266=CARTESIAN_POINT('Ctrl Pts',(10.3594275150096,18.6963263828107,-9.45128055628077));
#36267=CARTESIAN_POINT('Ctrl Pts',(9.94475486011823,18.6812985797984,-9.32435816539428));
#36268=CARTESIAN_POINT('Ctrl Pts',(52.0406002125752,19.4355555088431,0.536630679855416));
#36269=CARTESIAN_POINT('Ctrl Pts',(51.7640075955767,19.4044605226273,0.204462065251584));
#36270=CARTESIAN_POINT('Ctrl Pts',(51.4808914055444,19.3735658358572,-0.124235214003335));
#36271=CARTESIAN_POINT('Ctrl Pts',(50.2449190227734,19.2426748194849,-1.51134745512144));
#36272=CARTESIAN_POINT('Ctrl Pts',(48.2584669237558,19.0517849995255,-3.50670891787662));
#36273=CARTESIAN_POINT('Ctrl Pts',(45.0320086735472,18.7933185397158,-6.10982075851879));
#36274=CARTESIAN_POINT('Ctrl Pts',(41.020376532225,18.5218580841843,-8.68754002034028));
#36275=CARTESIAN_POINT('Ctrl Pts',(36.7501523857616,18.2836948825759,-10.685800216972));
#36276=CARTESIAN_POINT('Ctrl Pts',(32.2975809316394,18.0697821020849,-12.0966666900533));
#36277=CARTESIAN_POINT('Ctrl Pts',(27.7398821156923,17.8693333343866,-13.0335373077252));
#36278=CARTESIAN_POINT('Ctrl Pts',(23.1017460362113,17.6778661310593,-13.3729183254776));
#36279=CARTESIAN_POINT('Ctrl Pts',(18.4597065884447,17.4826662284719,-13.1077148144475));
#36280=CARTESIAN_POINT('Ctrl Pts',(14.5131353656531,17.3068805329357,-12.4627659844579));
#36281=CARTESIAN_POINT('Ctrl Pts',(11.926957780631,17.1802068447994,-11.7524052617819));
#36282=CARTESIAN_POINT('Ctrl Pts',(10.2480732137341,17.0925519552341,-11.192249695301));
#36283=CARTESIAN_POINT('Ctrl Pts',(9.84812468771829,17.0712544126695,-11.0512080030603));
#36284=CARTESIAN_POINT('Ctrl Pts',(9.45120285539089,17.0497370990139,-10.9036522294195));
#36285=CARTESIAN_POINT('Ctrl Pts',(51.0842942568547,17.8320672383652,-3.84088922097839));
#36286=CARTESIAN_POINT('Ctrl Pts',(50.7974662443455,17.7976045693245,-4.1536391251297));
#36287=CARTESIAN_POINT('Ctrl Pts',(50.5042776068662,17.7633163796081,-4.46263132338155));
#36288=CARTESIAN_POINT('Ctrl Pts',(49.2260465041698,17.6178640028275,-5.7644191441608));
#36289=CARTESIAN_POINT('Ctrl Pts',(47.1815905690377,17.4049846203341,-7.62450873541984));
#36290=CARTESIAN_POINT('Ctrl Pts',(43.8893661957293,17.1135517229592,-10.0126928844568));
#36291=CARTESIAN_POINT('Ctrl Pts',(39.827079861979,16.8027253827761,-12.3277800623226));
#36292=CARTESIAN_POINT('Ctrl Pts',(35.5404007724829,16.523022337621,-14.0512431159597));
#36293=CARTESIAN_POINT('Ctrl Pts',(31.1079579099481,16.2641978724915,-15.1792080319066));
#36294=CARTESIAN_POINT('Ctrl Pts',(26.6009083346784,16.0157341831644,-15.8288669477005));
#36295=CARTESIAN_POINT('Ctrl Pts',(22.0531293441551,15.7719994721116,-15.8783661204877));
#36296=CARTESIAN_POINT('Ctrl Pts',(17.5434519798272,15.5202180684676,-15.3246701276807));
#36297=CARTESIAN_POINT('Ctrl Pts',(13.7401700421149,15.2931736272884,-14.4352340302876));
#36298=CARTESIAN_POINT('Ctrl Pts',(11.2700908184494,15.130708702949,-13.5649582362775));
#36299=CARTESIAN_POINT('Ctrl Pts',(9.67456871062958,15.0190926843839,-12.9010089872194));
#36300=CARTESIAN_POINT('Ctrl Pts',(9.29511173349696,14.9920326361705,-12.7352506969355));
#36301=CARTESIAN_POINT('Ctrl Pts',(8.91916102165301,14.9647422323135,-12.5631815717126));
#36302=CARTESIAN_POINT('Ctrl Pts',(50.1725377178788,15.7638142683891,-8.00723153985461));
#36303=CARTESIAN_POINT('Ctrl Pts',(49.8755477488999,15.7283726072843,-8.30050397680349));
#36304=CARTESIAN_POINT('Ctrl Pts',(49.5723712501119,15.6930928161318,-8.58970540631576));
#36305=CARTESIAN_POINT('Ctrl Pts',(48.2522976624192,15.543379415412,-9.80568727794157));
#36306=CARTESIAN_POINT('Ctrl Pts',(46.1504868067129,15.3241289383934,-11.5297341520232));
#36307=CARTESIAN_POINT('Ctrl Pts',(42.7935015732012,15.0227233638938,-13.7016902252622));
#36308=CARTESIAN_POINT('Ctrl Pts',(38.6817671766857,14.6988957424381,-15.7524134665736));
#36309=CARTESIAN_POINT('Ctrl Pts',(34.3798754649118,14.4035050799014,-17.1990244745944));
#36310=CARTESIAN_POINT('Ctrl Pts',(29.9688301701935,14.1252237593235,-18.0416345493436));
#36311=CARTESIAN_POINT('Ctrl Pts',(25.5137144392418,13.8539516979883,-18.4012723388184));
#36312=CARTESIAN_POINT('Ctrl Pts',(21.0575892960011,13.5829362127958,-18.1575891929838));
#36313=CARTESIAN_POINT('Ctrl Pts',(16.6815712532013,13.2994842764397,-17.3115432147165));
#36314=CARTESIAN_POINT('Ctrl Pts',(13.0226854098743,13.0425486753816,-16.1739021884697));
#36315=CARTESIAN_POINT('Ctrl Pts',(10.6694354351882,12.8585920936854,-15.1409396349232));
#36316=CARTESIAN_POINT('Ctrl Pts',(9.1577531507647,12.7324540777387,-14.3712708374681));
#36317=CARTESIAN_POINT('Ctrl Pts',(8.79897600642064,12.7018988467546,-14.1803688483644));
#36318=CARTESIAN_POINT('Ctrl Pts',(8.44425573048895,12.6711030837425,-13.9833955784899));
#36319=CARTESIAN_POINT('Ctrl Pts',(49.3152608397176,13.2592937677246,-11.9222078443566));
#36320=CARTESIAN_POINT('Ctrl Pts',(49.0081288955748,13.2252177231213,-12.1961718735344));
#36321=CARTESIAN_POINT('Ctrl Pts',(48.6949962864853,13.191306123502,-12.4657287651272));
#36322=CARTESIAN_POINT('Ctrl Pts',(47.3332740813492,13.0474600457288,-13.596431013652));
#36323=CARTESIAN_POINT('Ctrl Pts',(45.1744154124219,12.8372075593629,-15.1851844684315));
#36324=CARTESIAN_POINT('Ctrl Pts',(41.7531577370126,12.5484949329477,-17.1418284947311));
#36325=CARTESIAN_POINT('Ctrl Pts',(37.5925733551791,12.2377054846042,-18.9289743222429));
#36326=CARTESIAN_POINT('Ctrl Pts',(33.2760966864303,11.9522310106351,-20.0991214081145));
#36327=CARTESIAN_POINT('Ctrl Pts',(28.8870963556916,11.6797819251771,-20.6563051510431));
#36328=CARTESIAN_POINT('Ctrl Pts',(24.4845718229607,11.4108111467242,-20.725453230849));
#36329=CARTESIAN_POINT('Ctrl Pts',(20.1207628048483,11.1374939458242,-20.1875872960187));
#36330=CARTESIAN_POINT('Ctrl Pts',(15.8790594562062,10.8473681096278,-19.0476098848715));
#36331=CARTESIAN_POINT('Ctrl Pts',(12.3651212340625,10.5820480444149,-17.6599891786549));
#36332=CARTESIAN_POINT('Ctrl Pts',(10.1290577747649,10.3910369789073,-16.4628640701335));
#36333=CARTESIAN_POINT('Ctrl Pts',(8.70144575840633,10.2599216927486,-15.5864046825366));
#36334=CARTESIAN_POINT('Ctrl Pts',(8.36346441706814,10.2281653805015,-15.3701525403304));
#36335=CARTESIAN_POINT('Ctrl Pts',(8.03014834074206,10.1961599190035,-15.1481197425553));
#36336=CARTESIAN_POINT('Ctrl Pts',(48.5068954184471,10.420684636249,-15.6143972186621));
#36337=CARTESIAN_POINT('Ctrl Pts',(48.1896003239712,10.3898269637342,-15.8693164159478));
#36338=CARTESIAN_POINT('Ctrl Pts',(47.8665042940188,10.3591499865554,-16.1194724741786));
#36339=CARTESIAN_POINT('Ctrl Pts',(46.463169475174,10.2291883131935,-17.1658511436441));
#36340=CARTESIAN_POINT('Ctrl Pts',(44.2473255358791,10.0401067219452,-18.6207182709661));
#36341=CARTESIAN_POINT('Ctrl Pts',(40.7619090059636,9.78206378055234,-20.3639629021039));
#36342=CARTESIAN_POINT('Ctrl Pts',(36.5526268350307,9.50499638561923,-21.8895038071216));
#36343=CARTESIAN_POINT('Ctrl Pts',(32.2217373255655,9.24981780003299,-22.7848040491436));
#36344=CARTESIAN_POINT('Ctrl Pts',(27.8549660182239,9.00337535985762,-23.057781793126));
#36345=CARTESIAN_POINT('Ctrl Pts',(23.5052216104395,8.75677479408939,-22.8373239688022));
#36346=CARTESIAN_POINT('Ctrl Pts',(19.2339176885499,8.50116890088297,-22.0057156544696));
#36347=CARTESIAN_POINT('Ctrl Pts',(15.1267085905075,8.22444592813344,-20.5717738964972));
#36348=CARTESIAN_POINT('Ctrl Pts',(11.757861066389,7.96804930448713,-18.9338087527527));
#36349=CARTESIAN_POINT('Ctrl Pts',(9.63906942037282,7.78162503245108,-17.5720463596553));
#36350=CARTESIAN_POINT('Ctrl Pts',(8.29557955058743,7.65323614745839,-16.5884059526543));
#36351=CARTESIAN_POINT('Ctrl Pts',(7.97844957882663,7.62212996336316,-16.3467742297976));
#36352=CARTESIAN_POINT('Ctrl Pts',(7.66663340357728,7.59076668565169,-16.0997163540814));
#36353=CARTESIAN_POINT('Ctrl Pts',(47.7663041384592,7.18298363715391,-19.0008728096664));
#36354=CARTESIAN_POINT('Ctrl Pts',(47.4387949271775,7.15763661423686,-19.2372123412692));
#36355=CARTESIAN_POINT('Ctrl Pts',(47.1056968685837,7.13250342173354,-19.4684182906929));
#36356=CARTESIAN_POINT('Ctrl Pts',(45.6606453368009,7.02634360727853,-20.4323367979011));
#36357=CARTESIAN_POINT('Ctrl Pts',(43.3876649619329,6.87350147707393,-21.7560858428746));
#36358=CARTESIAN_POINT('Ctrl Pts',(39.8378843858508,6.66841421880391,-23.2897975200252));
#36359=CARTESIAN_POINT('Ctrl Pts',(35.5796858561183,6.45075222930465,-24.557880503093));
#36360=CARTESIAN_POINT('Ctrl Pts',(31.2341850293128,6.25122984378583,-25.181992433157));
#36361=CARTESIAN_POINT('Ctrl Pts',(26.8894543185663,6.05595707526583,-25.1738921979679));
#36362=CARTESIAN_POINT('Ctrl Pts',(22.592303780841,5.8568061689083,-24.6665137174336));
#36363=CARTESIAN_POINT('Ctrl Pts',(18.4133138682224,5.64398234710963,-23.5432735796297));
#36364=CARTESIAN_POINT('Ctrl Pts',(14.4403913295249,5.40587468584602,-21.8168778028767));
#36365=CARTESIAN_POINT('Ctrl Pts',(11.2164396726889,5.18017895256177,-19.9294422021648));
#36366=CARTESIAN_POINT('Ctrl Pts',(9.21477519698173,5.01301666232781,-18.4033400289031));
#36367=CARTESIAN_POINT('Ctrl Pts',(7.9553063361445,4.89707445701614,-17.3126195831835));
#36368=CARTESIAN_POINT('Ctrl Pts',(7.65902789693625,4.86894780999335,-17.0457039568974));
#36369=CARTESIAN_POINT('Ctrl Pts',(7.3687334895065,4.84055053954568,-16.773786950835));
#36370=CARTESIAN_POINT('Ctrl Pts',(47.1034759657558,3.57357815210241,-22.0401821714072));
#36371=CARTESIAN_POINT('Ctrl Pts',(46.7656567924019,3.55599962931061,-22.258629623147));
#36372=CARTESIAN_POINT('Ctrl Pts',(46.422469525106,3.53868515668548,-22.4715649470704));
#36373=CARTESIAN_POINT('Ctrl Pts',(44.9353728299774,3.46609807861293,-23.3558908474528));
#36374=CARTESIAN_POINT('Ctrl Pts',(42.6047596053836,3.36435917107101,-24.5528077821968));
#36375=CARTESIAN_POINT('Ctrl Pts',(38.9898867387259,3.23426720235262,-25.883075497778));
#36376=CARTESIAN_POINT('Ctrl Pts',(34.6819369539376,3.10147907156715,-26.9003845437934));
#36377=CARTESIAN_POINT('Ctrl Pts',(30.3210023530336,2.98285053627008,-27.2594428206669));
#36378=CARTESIAN_POINT('Ctrl Pts',(25.9974922221956,2.86388130857434,-26.9758226313354));
#36379=CARTESIAN_POINT('Ctrl Pts',(21.7521116924467,2.73730530568202,-26.1866104301047));
#36380=CARTESIAN_POINT('Ctrl Pts',(17.6645996841604,2.59247375589619,-24.7762264723451));
#36381=CARTESIAN_POINT('Ctrl Pts',(13.8251038305928,2.41842603756845,-22.7612587515336));
#36382=CARTESIAN_POINT('Ctrl Pts',(10.745289428394,2.24547053120763,-20.6272650645164));
#36383=CARTESIAN_POINT('Ctrl Pts',(8.86022855638182,2.11246131963295,-18.9384898393954));
#36384=CARTESIAN_POINT('Ctrl Pts',(7.68442932568005,2.01884144332686,-17.7416968510392));
#36385=CARTESIAN_POINT('Ctrl Pts',(7.40891951245342,1.99605339732081,-17.4498093694952));
#36386=CARTESIAN_POINT('Ctrl Pts',(7.14006311638173,1.9729679754383,-17.1534135736909));
#36387=CARTESIAN_POINT('Ctrl Pts',(46.5932402567772,0.237308438758995,-24.3880208385881));
#36388=CARTESIAN_POINT('Ctrl Pts',(46.2464938933772,0.227921876287717,-24.5917084460452));
#36389=CARTESIAN_POINT('Ctrl Pts',(45.8945747997372,0.218854274805993,-24.789555458612));
#36390=CARTESIAN_POINT('Ctrl Pts',(44.3711113907725,0.181679983795775,-25.6080867216743));
#36391=CARTESIAN_POINT('Ctrl Pts',(41.9905999455746,0.133848323063104,-26.6999270667671));
#36392=CARTESIAN_POINT('Ctrl Pts',(38.3191944032503,0.0830496793456984,
-27.8610127422469));
#36393=CARTESIAN_POINT('Ctrl Pts',(33.9677453036371,0.0403924264632703,
-28.6691257307571));
#36394=CARTESIAN_POINT('Ctrl Pts',(29.592731205814,0.00837005963384143,
-28.8063457531801));
#36395=CARTESIAN_POINT('Ctrl Pts',(25.2865576591566,-0.0279539839125438,
-28.2915019174398));
#36396=CARTESIAN_POINT('Ctrl Pts',(21.0846934817227,-0.0750512999789021,
-27.2653201831544));
#36397=CARTESIAN_POINT('Ctrl Pts',(17.0747213437724,-0.14423024726241,-25.6129959380492));
#36398=CARTESIAN_POINT('Ctrl Pts',(13.3487019191347,-0.245792879606331,
-23.3544485950546));
#36399=CARTESIAN_POINT('Ctrl Pts',(10.3916545614428,-0.358291148292244,
-21.0120689099268));
#36400=CARTESIAN_POINT('Ctrl Pts',(8.60600662574962,-0.451704594358635,
-19.1856437846783));
#36401=CARTESIAN_POINT('Ctrl Pts',(7.50156840296396,-0.519340602547392,
-17.8990473762172));
#36402=CARTESIAN_POINT('Ctrl Pts',(7.24376168775053,-0.535923052101836,
-17.5860758002247));
#36403=CARTESIAN_POINT('Ctrl Pts',(6.9931674919517,-0.552841667182328,-17.2690690103583));
#36404=CARTESIAN_POINT('Ctrl Pts',(46.2947220098623,-2.14030259993981,-25.7688006063388));
#36405=CARTESIAN_POINT('Ctrl Pts',(45.941959111431,-2.14321532053782,-25.9630972825016));
#36406=CARTESIAN_POINT('Ctrl Pts',(45.5841524820316,-2.14576465810466,-26.15133557776));
#36407=CARTESIAN_POINT('Ctrl Pts',(44.036157375114,-2.15494826818845,-26.9279311689218));
#36408=CARTESIAN_POINT('Ctrl Pts',(41.6219424526533,-2.16016260296573,-27.9526124656332));
#36409=CARTESIAN_POINT('Ctrl Pts',(37.9121954585346,-2.1481556077715,-29.0050620130212));
#36410=CARTESIAN_POINT('Ctrl Pts',(33.5309876602201,-2.11918777525101,-29.678331446371));
#36411=CARTESIAN_POINT('Ctrl Pts',(29.1458287536112,-2.08197924289826,-29.6719949919839));
#36412=CARTESIAN_POINT('Ctrl Pts',(24.850450699298,-2.05170003121316,-29.0070497291441));
#36413=CARTESIAN_POINT('Ctrl Pts',(20.6768296464201,-2.03426137368081,-27.8267065281117));
#36414=CARTESIAN_POINT('Ctrl Pts',(16.7177727938086,-2.04135770257883,-26.0166226684537));
#36415=CARTESIAN_POINT('Ctrl Pts',(13.0666111841149,-2.08278583441843,-23.5989471937519));
#36416=CARTESIAN_POINT('Ctrl Pts',(10.1907160216954,-2.14471303148954,-21.1202535264619));
#36417=CARTESIAN_POINT('Ctrl Pts',(8.47087180152222,-2.20477046252904,-19.2036851023432));
#36418=CARTESIAN_POINT('Ctrl Pts',(7.4136936437243,-2.25046208753918,-17.8582514463191));
#36419=CARTESIAN_POINT('Ctrl Pts',(7.16760061362021,-2.26180965939547,-17.5314923980718));
#36420=CARTESIAN_POINT('Ctrl Pts',(6.92907933707999,-2.27353152926925,-17.2010333337206));
#36421=CARTESIAN_POINT('Ctrl Pts',(46.1037904071156,-3.83428286431684,-26.6551216886457));
#36422=CARTESIAN_POINT('Ctrl Pts',(45.7468392473426,-3.83237339034492,-26.8431064726811));
#36423=CARTESIAN_POINT('Ctrl Pts',(45.384933450483,-3.83006698099443,-27.0248826050977));
#36424=CARTESIAN_POINT('Ctrl Pts',(43.8198552158363,-3.81839846831683,-27.7732596177199));
#36425=CARTESIAN_POINT('Ctrl Pts',(41.3821512642932,-3.79185933798401,-28.7526727554059));
#36426=CARTESIAN_POINT('Ctrl Pts',(37.6456155051948,-3.73301479320489,-29.7316906927672));
#36427=CARTESIAN_POINT('Ctrl Pts',(33.2435059855666,-3.65055513724086,-30.3136066492174));
#36428=CARTESIAN_POINT('Ctrl Pts',(28.8510048450698,-3.56151400652134,-30.2097891824573));
#36429=CARTESIAN_POINT('Ctrl Pts',(24.5627595764646,-3.48120332570528,-29.4427347388257));
#36430=CARTESIAN_POINT('Ctrl Pts',(20.4083312364158,-3.41513875248544,-28.1573941121625));
#36431=CARTESIAN_POINT('Ctrl Pts',(16.4841372973616,-3.37526128513496,-26.2397257261537));
#36432=CARTESIAN_POINT('Ctrl Pts',(12.8843854212511,-3.37099617994084,-23.7134252414379));
#36433=CARTESIAN_POINT('Ctrl Pts',(10.0642958903975,-3.39437469848804,-21.1416193490947));
#36434=CARTESIAN_POINT('Ctrl Pts',(8.38974213062551,-3.42893690611626,-19.1634442433015));
#36435=CARTESIAN_POINT('Ctrl Pts',(7.36510236943545,-3.45783930783476,-17.7777914941477));
#36436=CARTESIAN_POINT('Ctrl Pts',(7.1270679382079,-3.46518513130081,-17.441619342386));
#36437=CARTESIAN_POINT('Ctrl Pts',(6.89684614274116,-3.47293757911652,-17.1019872449569));
#36438=CARTESIAN_POINT('Ctrl Pts',(46.0528159428914,-4.30636894546118,-26.8921103922779));
#36439=CARTESIAN_POINT('Ctrl Pts',(45.6947067519107,-4.3031084050989,-27.0783820415091));
#36440=CARTESIAN_POINT('Ctrl Pts',(45.3316670409603,-4.29944065268701,-27.2584034254891));
#36441=CARTESIAN_POINT('Ctrl Pts',(43.7618609679394,-4.28192251284736,-27.9991144594585));
#36442=CARTESIAN_POINT('Ctrl Pts',(41.3176536774688,-4.24645759656194,-28.9662083465854));
#36443=CARTESIAN_POINT('Ctrl Pts',(37.573695569515,-4.17439213330946,-29.9251866742588));
#36444=CARTESIAN_POINT('Ctrl Pts',(33.165788764262,-4.07676875425951,-30.4821188840162));
#36445=CARTESIAN_POINT('Ctrl Pts',(28.7712425645872,-3.97294922980807,-30.3515908256571));
#36446=CARTESIAN_POINT('Ctrl Pts',(24.4849562345802,-3.87828739688684,-29.5565265077524));
#36447=CARTESIAN_POINT('Ctrl Pts',(20.3358191796481,-3.79820251809058,-28.2423765542426));
#36448=CARTESIAN_POINT('Ctrl Pts',(16.4212365487571,-3.74469501429227,-26.2951939954818));
#36449=CARTESIAN_POINT('Ctrl Pts',(12.835640508744,-3.72710099262819,-23.7391203941118));
#36450=CARTESIAN_POINT('Ctrl Pts',(10.0308926410816,-3.7392015362719,-21.1418289429546));
#36451=CARTESIAN_POINT('Ctrl Pts',(8.36877216587862,-3.76629674044718,-19.1468130501193));
#36452=CARTESIAN_POINT('Ctrl Pts',(7.35305705617724,-3.79028538091932,-17.7501753024402));
#36453=CARTESIAN_POINT('Ctrl Pts',(7.11723098643449,-3.79646095010219,-17.4114340805589));
#36454=CARTESIAN_POINT('Ctrl Pts',(6.88928170242563,-3.80305340259771,-17.0693002554959));
#36455=CARTESIAN_POINT('Ctrl Pts',(46.0037076365571,-4.78145508078572,-27.120777531992));
#36456=CARTESIAN_POINT('Ctrl Pts',(45.6444433560399,-4.77682808742727,-27.305369940422));
#36457=CARTESIAN_POINT('Ctrl Pts',(45.2802717676693,-4.7717826224726,-27.4836706378466));
#36458=CARTESIAN_POINT('Ctrl Pts',(43.7057426010136,-4.74834091216943,-28.2168616760953));
#36459=CARTESIAN_POINT('Ctrl Pts',(41.2550359871502,-4.70381966688121,-29.1718493157503));
#36460=CARTESIAN_POINT('Ctrl Pts',(37.5036551789753,-4.61828583278682,-30.1110783850339));
#36461=CARTESIAN_POINT('Ctrl Pts',(33.0899455447831,-4.50515190400754,-30.6433355850274));
#36462=CARTESIAN_POINT('Ctrl Pts',(28.6933453214368,-4.38613315046716,-30.4863760222648));
#36463=CARTESIAN_POINT('Ctrl Pts',(24.4090037684511,-4.27662792828432,-29.6635634830365));
#36464=CARTESIAN_POINT('Ctrl Pts',(20.2651358983066,-4.18197237106197,-28.3208663256634));
#36465=CARTESIAN_POINT('Ctrl Pts',(16.3601222932309,-4.11421750462538,-26.3444433325659));
#36466=CARTESIAN_POINT('Ctrl Pts',(12.7886013364524,-4.08262421860679,-23.7588994143533));
#36467=CARTESIAN_POINT('Ctrl Pts',(9.99908233100923,-4.0828488851085,-21.1364173862108));
#36468=CARTESIAN_POINT('Ctrl Pts',(8.34928571759199,-4.10207414795096,-19.1247770659859));
#36469=CARTESIAN_POINT('Ctrl Pts',(7.34240870565719,-4.12088738197538,-17.7173046985667));
#36470=CARTESIAN_POINT('Ctrl Pts',(7.10876813411939,-4.12583098108427,-17.3760304556457));
#36471=CARTESIAN_POINT('Ctrl Pts',(6.88306649246102,-4.13120272145022,-17.0314308181555));
#36472=CARTESIAN_POINT('',(46.8671786463539,20.7105311502984,0.856680668514059));
#36473=CARTESIAN_POINT('Ctrl Pts',(46.8671786463539,20.7105311502984,0.85668066851405));
#36474=CARTESIAN_POINT('Ctrl Pts',(42.9014764671361,20.5483438544848,-2.48144010722812));
#36475=CARTESIAN_POINT('Ctrl Pts',(38.2828465564874,20.4520245495079,-5.02872828673426));
#36476=CARTESIAN_POINT('Ctrl Pts',(28.4491423215176,20.3052748660675,-8.30400152038972));
#36477=CARTESIAN_POINT('Ctrl Pts',(23.2335530202462,20.248474007324,-9.03506651020502));
#36478=CARTESIAN_POINT('Ctrl Pts',(18.0621112303383,20.1925493450898,-8.74422771304759));
#36479=CARTESIAN_POINT('',(36.2576798233721,-3.27137091447503,-29.7093686459786));
#36480=CARTESIAN_POINT('Ctrl Pts',(46.8671786463482,20.7105311502992,0.856680668513758));
#36481=CARTESIAN_POINT('Ctrl Pts',(46.9249887269589,19.9641948262067,-2.30600051616087));
#36482=CARTESIAN_POINT('Ctrl Pts',(46.6560935232336,18.7336174322536,-5.37662766955232));
#36483=CARTESIAN_POINT('Ctrl Pts',(45.5710956442331,15.6437709263415,-11.4562521714677));
#36484=CARTESIAN_POINT('Ctrl Pts',(44.6678816065033,13.6706054953476,-14.5214537476068));
#36485=CARTESIAN_POINT('Ctrl Pts',(42.5169745662042,9.45712578015162,-19.9441390711336));
#36486=CARTESIAN_POINT('Ctrl Pts',(41.2615426847051,7.18268855808127,-22.3812734554399));
#36487=CARTESIAN_POINT('Ctrl Pts',(38.6998696152663,2.26699026933656,-26.5599268565702));
#36488=CARTESIAN_POINT('Ctrl Pts',(37.3979964354348,-0.36522399219511,-28.317712640974));
#36489=CARTESIAN_POINT('Ctrl Pts',(36.2576793998219,-3.27137053313468,-29.709369095263));
#36490=CARTESIAN_POINT('Ctrl Pts',(36.2576797497044,-3.2713710013512,-29.7093681727007));
#36491=CARTESIAN_POINT('Ctrl Pts',(35.4899009191443,-3.25992112204952,-29.8267742981394));
#36492=CARTESIAN_POINT('Ctrl Pts',(34.7207207197571,-3.24789096533568,-29.9144772584936));
#36493=CARTESIAN_POINT('Ctrl Pts',(33.9517915369502,-3.23555894384663,-29.9728534820301));
#36494=CARTESIAN_POINT('Ctrl Pts',(32.0686564302618,-3.2053573815679,-30.1158189441238));
#36495=CARTESIAN_POINT('Ctrl Pts',(30.1870269834765,-3.17334534347451,-30.0828890834105));
#36496=CARTESIAN_POINT('Ctrl Pts',(28.3311759587029,-3.14345008158505,-29.8797419860564));
#36497=CARTESIAN_POINT('Ctrl Pts',(27.0939418794257,-3.12351990598108,-29.7443105809502));
#36498=CARTESIAN_POINT('Ctrl Pts',(25.8681648777386,-3.10453051989494,-29.5332270629972));
#36499=CARTESIAN_POINT('Ctrl Pts',(24.6610277249437,-3.08752071373525,-29.2482168634081));
#36500=CARTESIAN_POINT('Ctrl Pts',(23.4538905727806,-3.07051090758448,-28.9632066639682));
#36501=CARTESIAN_POINT('Ctrl Pts',(22.2653932694828,-3.0554806813514,-28.6042697829724));
#36502=CARTESIAN_POINT('Ctrl Pts',(21.1027127831863,-3.04339100491456,-28.1731487078922));
#36503=CARTESIAN_POINT('Ctrl Pts',(19.358692055909,-3.02525649028182,-27.5264670960756));
#36504=CARTESIAN_POINT('Ctrl Pts',(17.6727591667208,-3.01373821257335,-26.7173710480374));
#36505=CARTESIAN_POINT('Ctrl Pts',(16.0690765496337,-3.01128625574909,-25.7518436565054));
#36506=CARTESIAN_POINT('Ctrl Pts',(14.9999548074193,-3.00965161787008,-25.1081587303288));
#36507=CARTESIAN_POINT('Ctrl Pts',(13.9673887414643,-3.01204645592803,-24.3949487628904));
#36508=CARTESIAN_POINT('Ctrl Pts',(12.9785164402689,-3.01891855380822,-23.6140047827048));
#36509=CARTESIAN_POINT('Ctrl Pts',(11.9896442576446,-3.02579065086441,-22.8330608961585));
#36510=CARTESIAN_POINT('Ctrl Pts',(11.0444658292623,-3.03714000665748,-21.9843830131019));
#36511=CARTESIAN_POINT('Ctrl Pts',(10.1501043009641,-3.05321938564873,-21.069763289763));
#36512=CARTESIAN_POINT('Ctrl Pts',(9.78156805938634,-3.05984515577954,-20.6928793288064));
#36513=CARTESIAN_POINT('Ctrl Pts',(9.42166046939857,-3.06727406915266,-20.3047985397277));
#36514=CARTESIAN_POINT('Ctrl Pts',(9.07087845564185,-3.07550335254719,-19.9056465116819));
#36515=CARTESIAN_POINT('Ctrl Pts',(45.973362676981,-4.68328060676847,-27.2756663271766));
#36516=CARTESIAN_POINT('Ctrl Pts',(45.6126991612577,-4.67927906663786,-27.4604236536159));
#36517=CARTESIAN_POINT('Ctrl Pts',(45.2471033099969,-4.67486342687383,-27.6388296622253));
#36518=CARTESIAN_POINT('Ctrl Pts',(43.6710473719894,-4.65418501649615,-28.3700492381431));
#36519=CARTESIAN_POINT('Ctrl Pts',(41.2202507588911,-4.61395560865182,-29.3209731200025));
#36520=CARTESIAN_POINT('Ctrl Pts',(37.4689495057187,-4.53496565777432,-30.2540302896408));
#36521=CARTESIAN_POINT('Ctrl Pts',(33.055595633981,-4.42959393838223,-30.7790187239315));
#36522=CARTESIAN_POINT('Ctrl Pts',(28.659697939306,-4.31850354734918,-30.6147326637025));
#36523=CARTESIAN_POINT('Ctrl Pts',(24.3764348754538,-4.2170896233612,-29.7845731359287));
#36524=CARTESIAN_POINT('Ctrl Pts',(20.2339666249731,-4.13063759391767,-28.4345208839583));
#36525=CARTESIAN_POINT('Ctrl Pts',(16.3307767357573,-4.07121155600733,-26.4507623239868));
#36526=CARTESIAN_POINT('Ctrl Pts',(12.7615353803547,-4.04803120464602,-23.8579397816895));
#36527=CARTESIAN_POINT('Ctrl Pts',(9.97429755410247,-4.055480889925,-21.2292769138081));
#36528=CARTESIAN_POINT('Ctrl Pts',(8.32624150720379,-4.07952578289679,-19.2135755950718));
#36529=CARTESIAN_POINT('Ctrl Pts',(7.31929162466779,-4.10152925776619,-17.801647007576));
#36530=CARTESIAN_POINT('Ctrl Pts',(7.08474911781699,-4.1072571624472,-17.4579084277431));
#36531=CARTESIAN_POINT('Ctrl Pts',(6.85824142480293,-4.11341014061892,-17.1108288866612));
#36532=CARTESIAN_POINT('Ctrl Pts',(46.0345375598687,-4.24009445412503,-26.9919991555953));
#36533=CARTESIAN_POINT('Ctrl Pts',(45.6750556727933,-4.23725223817857,-27.1786531095111));
#36534=CARTESIAN_POINT('Ctrl Pts',(45.3106133083243,-4.23400446880359,-27.3590016647185));
#36535=CARTESIAN_POINT('Ctrl Pts',(43.7393368113889,-4.21832863439708,-28.0986817692919));
#36536=CARTESIAN_POINT('Ctrl Pts',(41.2950934490877,-4.18572164472913,-29.0631532067729));
#36537=CARTESIAN_POINT('Ctrl Pts',(37.5512149138899,-4.11799618192084,-30.0181518488659));
#36538=CARTESIAN_POINT('Ctrl Pts',(33.1435649281886,-4.02550335874969,-30.5704030878674));
#36539=CARTESIAN_POINT('Ctrl Pts',(28.7494912840676,-3.92690475481451,-30.4351662245983));
#36540=CARTESIAN_POINT('Ctrl Pts',(24.4639098993022,-3.83755718932749,-29.6353920659615));
#36541=CARTESIAN_POINT('Ctrl Pts',(20.3156741014525,-3.76285616468038,-28.3165409874486));
#36542=CARTESIAN_POINT('Ctrl Pts',(16.4022501763199,-3.71481495977278,-26.3646862042512));
#36543=CARTESIAN_POINT('Ctrl Pts',(12.8180874502053,-3.70275434803773,-23.8039921794956));
#36544=CARTESIAN_POINT('Ctrl Pts',(10.014764308943,-3.71962751323487,-21.2027861208478));
#36545=CARTESIAN_POINT('Ctrl Pts',(8.35372688131093,-3.74992063397164,-19.2052003915485));
#36546=CARTESIAN_POINT('Ctrl Pts',(7.3374661001949,-3.77604797989279,-17.8050928273303));
#36547=CARTESIAN_POINT('Ctrl Pts',(7.10061080602625,-3.78276245762616,-17.464127862853));
#36548=CARTESIAN_POINT('Ctrl Pts',(6.87172363105669,-3.78989370687861,-17.1197471100359));
#36549=CARTESIAN_POINT('Ctrl Pts',(46.0970059190559,-3.80075287541765,-26.7026202149032));
#36550=CARTESIAN_POINT('Ctrl Pts',(45.7387037966384,-3.79905339336963,-26.8911923080337));
#36551=CARTESIAN_POINT('Ctrl Pts',(45.3754124664879,-3.79695621683146,-27.0735048418965));
#36552=CARTESIAN_POINT('Ctrl Pts',(43.8089024562329,-3.78620663871065,-27.8217362732406));
#36553=CARTESIAN_POINT('Ctrl Pts',(41.371192364366,-3.76109400159902,-28.7998819866087));
#36554=CARTESIAN_POINT('Ctrl Pts',(37.6347096129005,-3.70440674399875,-29.7769780940438));
#36555=CARTESIAN_POINT('Ctrl Pts',(33.2327383479775,-3.62448835210827,-30.3566365749797));
#36556=CARTESIAN_POINT('Ctrl Pts',(28.8404756925361,-3.53802316526296,-30.250552988433));
#36557=CARTESIAN_POINT('Ctrl Pts',(24.5525760323583,-3.46032715355504,-29.4812382422582));
#36558=CARTESIAN_POINT('Ctrl Pts',(20.3985825728977,-3.39690914788247,-28.1936488639279));
#36559=CARTESIAN_POINT('Ctrl Pts',(16.4749395169915,-3.35971861494906,-26.2737543336035));
#36560=CARTESIAN_POINT('Ctrl Pts',(12.8758609544234,-3.35817927654809,-23.7452608637003));
#36561=CARTESIAN_POINT('Ctrl Pts',(10.056435360143,-3.38391914529348,-21.1716020610987));
#36562=CARTESIAN_POINT('Ctrl Pts',(8.38238397495209,-3.42007079724739,-19.1922119346188));
#36563=CARTESIAN_POINT('Ctrl Pts',(7.35678013783898,-3.45006162272336,-17.8039874884584));
#36564=CARTESIAN_POINT('Ctrl Pts',(7.11760246326198,-3.45770043113048,-17.4658116774344));
#36565=CARTESIAN_POINT('Ctrl Pts',(6.8863244697825,-3.46574819271174,-17.1241457257504));
#36566=CARTESIAN_POINT('Ctrl Pts',(46.3218499125173,-2.2653457359543,-25.6621009480906));
#36567=CARTESIAN_POINT('Ctrl Pts',(45.9676956475964,-2.26761569662348,-25.8575133309122));
#36568=CARTESIAN_POINT('Ctrl Pts',(45.6084503547893,-2.26951335386862,-26.0468269264624));
#36569=CARTESIAN_POINT('Ctrl Pts',(44.0586916831692,-2.27586002752392,-26.8255305361844));
#36570=CARTESIAN_POINT('Ctrl Pts',(41.6439336730249,-2.27671432942662,-27.8523380738304));
#36571=CARTESIAN_POINT('Ctrl Pts',(37.9334156521198,-2.25814179129592,-28.9078977789232));
#36572=CARTESIAN_POINT('Ctrl Pts',(33.5513614110281,-2.2214798205824,-29.5846993393589));
#36573=CARTESIAN_POINT('Ctrl Pts',(29.1654252452448,-2.17652897108851,-29.5817711347714));
#36574=CARTESIAN_POINT('Ctrl Pts',(24.8693434695226,-2.13845241575724,-28.9201093573139));
#36575=CARTESIAN_POINT('Ctrl Pts',(20.6950799083771,-2.11316923258448,-27.7429517662975));
#36576=CARTESIAN_POINT('Ctrl Pts',(16.7354600708946,-2.11235831802136,-25.9359348634863));
#36577=CARTESIAN_POINT('Ctrl Pts',(13.0838196040227,-2.14581153060268,-23.5212178093802));
#36578=CARTESIAN_POINT('Ctrl Pts',(10.2075738210828,-2.20085463389179,-21.0449921098509));
#36579=CARTESIAN_POINT('Ctrl Pts',(8.48753717971688,-2.25628908058851,-19.1300289525424));
#36580=CARTESIAN_POINT('Ctrl Pts',(7.42888933073493,-2.29898278275007,-17.7839145087321));
#36581=CARTESIAN_POINT('Ctrl Pts',(7.18149013898659,-2.30966173471912,-17.4556298037868));
#36582=CARTESIAN_POINT('Ctrl Pts',(6.94174097526185,-2.32072459453129,-17.1235981440825));
#36583=CARTESIAN_POINT('Ctrl Pts',(46.7450706088707,0.42091842584111,-23.7082581849838));
#36584=CARTESIAN_POINT('Ctrl Pts',(46.3983038112075,0.412015546281074,-23.9161367305282));
#36585=CARTESIAN_POINT('Ctrl Pts',(46.0462690198602,0.403442573942463,-24.1182027052624));
#36586=CARTESIAN_POINT('Ctrl Pts',(44.5263831245904,0.368526239150617,-24.9523849210783));
#36587=CARTESIAN_POINT('Ctrl Pts',(42.1525358259181,0.324281374370589,-26.0676939450635));
#36588=CARTESIAN_POINT('Ctrl Pts',(38.4882271453103,0.279215865745994,-27.2657018770151));
#36589=CARTESIAN_POINT('Ctrl Pts',(34.1415021026478,0.243759038204317,-28.1186055579968));
#36590=CARTESIAN_POINT('Ctrl Pts',(29.7665531301524,0.21967725703067,-28.3023951485284));
#36591=CARTESIAN_POINT('Ctrl Pts',(25.4554695335823,0.192114722189047,-27.8353545953069));
#36592=CARTESIAN_POINT('Ctrl Pts',(21.2445496907064,0.154437491851918,-26.8576751479132));
#36593=CARTESIAN_POINT('Ctrl Pts',(17.2201347615873,0.0954817696064694,
-25.2543692928801));
#36594=CARTESIAN_POINT('Ctrl Pts',(13.4739839232542,0.0048363712043943,
-23.0448309980406));
#36595=CARTESIAN_POINT('Ctrl Pts',(10.4956451040933,-0.0979118428630517,
-20.7442185796579));
#36596=CARTESIAN_POINT('Ctrl Pts',(8.6930230569115,-0.184631554593919,-18.945324770953));
#36597=CARTESIAN_POINT('Ctrl Pts',(7.57504200713313,-0.247909792323189,
-17.6750591709347));
#36598=CARTESIAN_POINT('Ctrl Pts',(7.31286586886589,-0.263520166061751,
-17.3646161592107));
#36599=CARTESIAN_POINT('Ctrl Pts',(7.05787648054576,-0.279478515480188,
-17.0499880689702));
#36600=CARTESIAN_POINT('Ctrl Pts',(47.404986111522,3.93922736422659,-20.6755997409199));
#36601=CARTESIAN_POINT('Ctrl Pts',(47.0684640420326,3.92273017306588,-20.9015567403437));
#36602=CARTESIAN_POINT('Ctrl Pts',(46.7264339108031,3.90651491483579,-21.122098655959));
#36603=CARTESIAN_POINT('Ctrl Pts',(45.2480229962362,3.83888692720806,-22.0365898282304));
#36604=CARTESIAN_POINT('Ctrl Pts',(42.9309251724468,3.74496038387833,-23.27972878241));
#36605=CARTESIAN_POINT('Ctrl Pts',(39.3305341019574,3.6271896762232,-24.6827159172831));
#36606=CARTESIAN_POINT('Ctrl Pts',(35.0323762557642,3.50969140214063,-25.7882334176081));
#36607=CARTESIAN_POINT('Ctrl Pts',(30.6719240550635,3.40771510315772,-26.2389829367879));
#36608=CARTESIAN_POINT('Ctrl Pts',(26.3389517794478,3.30695483103527,-26.0494460750817));
#36609=CARTESIAN_POINT('Ctrl Pts',(22.075820938881,3.1998573133211,-25.3556539412325));
#36610=CARTESIAN_POINT('Ctrl Pts',(17.9597861203445,3.07607789704229,-24.0416439011457));
#36611=CARTESIAN_POINT('Ctrl Pts',(14.0803885674248,2.92448144596071,-22.1229486412386));
#36612=CARTESIAN_POINT('Ctrl Pts',(10.9582980306177,2.77158317941627,-20.0709337271445));
#36613=CARTESIAN_POINT('Ctrl Pts',(9.03949054530486,2.65236568914073,-18.4361422761851));
#36614=CARTESIAN_POINT('Ctrl Pts',(7.83806324235876,2.56779645721963,-17.2730525922546));
#36615=CARTESIAN_POINT('Ctrl Pts',(7.55508253700517,2.54707902977605,-16.9878808614455));
#36616=CARTESIAN_POINT('Ctrl Pts',(7.27861346550577,2.52604544176493,-16.6979630171119));
#36617=CARTESIAN_POINT('Ctrl Pts',(48.2293875139225,7.64857049485316,-16.8981516990451));
#36618=CARTESIAN_POINT('Ctrl Pts',(47.9044854606453,7.62538079009264,-17.1453036599416));
#36619=CARTESIAN_POINT('Ctrl Pts',(47.5738209702538,7.6024320797305,-17.387480874535));
#36620=CARTESIAN_POINT('Ctrl Pts',(46.142612130283,7.50598047950645,-18.3959113196943));
#36621=CARTESIAN_POINT('Ctrl Pts',(43.8900756880785,7.36825978906471,-19.7883331202706));
#36622=CARTESIAN_POINT('Ctrl Pts',(40.3623101677245,7.18657585481396,-21.4300219986148));
#36623=CARTESIAN_POINT('Ctrl Pts',(36.1191823553037,6.99739878870591,-22.8289978138919));
#36624=CARTESIAN_POINT('Ctrl Pts',(31.7748392253983,6.82819742189185,-23.5890542762665));
#36625=CARTESIAN_POINT('Ctrl Pts',(27.4163985899668,6.66543158101024,-23.7203074035036));
#36626=CARTESIAN_POINT('Ctrl Pts',(23.0931437411946,6.50060855796851,-23.3541400227856));
#36627=CARTESIAN_POINT('Ctrl Pts',(18.871936060649,6.32441606849526,-22.3733522608672));
#36628=CARTESIAN_POINT('Ctrl Pts',(14.8397692169601,6.12505774886043,-20.789058032324));
#36629=CARTESIAN_POINT('Ctrl Pts',(11.5529516632508,5.93384517916791,-19.022472123698));
#36630=CARTESIAN_POINT('Ctrl Pts',(9.50104963584418,5.79035915091665,-17.5758361408519));
#36631=CARTESIAN_POINT('Ctrl Pts',(8.2040429508047,5.69001969995687,-16.53554757429));
#36632=CARTESIAN_POINT('Ctrl Pts',(7.89722279090849,5.66551509710643,-16.2794272231178));
#36633=CARTESIAN_POINT('Ctrl Pts',(7.59612832462127,5.64071489355821,-16.0180105688444));
#36634=CARTESIAN_POINT('Ctrl Pts',(49.0074290450359,10.6050661536892,-13.3398928188639));
#36635=CARTESIAN_POINT('Ctrl Pts',(48.6926428289153,10.5777689837161,-13.6059506753262));
#36636=CARTESIAN_POINT('Ctrl Pts',(48.3718894359035,10.5506896266998,-13.867401871622));
#36637=CARTESIAN_POINT('Ctrl Pts',(46.9819221114144,10.4365567481294,-14.9594187343244));
#36638=CARTESIAN_POINT('Ctrl Pts',(44.785792189829,10.2719415070743,-16.4845031570036));
#36639=CARTESIAN_POINT('Ctrl Pts',(41.3214668828266,10.0511774947007,-18.3378392475286));
#36640=CARTESIAN_POINT('Ctrl Pts',(37.1263846220837,9.81863871620139,-19.9964958281689));
#36641=CARTESIAN_POINT('Ctrl Pts',(32.7960498298375,9.60967367489776,-21.0296519428195));
#36642=CARTESIAN_POINT('Ctrl Pts',(28.4152465042761,9.41153176383594,-21.4435784231541));
#36643=CARTESIAN_POINT('Ctrl Pts',(24.0393070860599,9.21500541081661,-21.3656747993208));
#36644=CARTESIAN_POINT('Ctrl Pts',(19.7259921649729,9.01175979868378,-20.6775485689242));
#36645=CARTESIAN_POINT('Ctrl Pts',(15.5600549717428,8.78956564702969,-19.3864322787829));
#36646=CARTESIAN_POINT('Ctrl Pts',(12.1290015717314,8.58124477590158,-17.8697330625877));
#36647=CARTESIAN_POINT('Ctrl Pts',(9.96056099183191,8.42762540105217,-16.5875825895315));
#36648=CARTESIAN_POINT('Ctrl Pts',(8.57986327584419,8.32086564673385,-15.6545659656521));
#36649=CARTESIAN_POINT('Ctrl Pts',(8.25218357257416,8.29482075310626,-15.4239074282687));
#36650=CARTESIAN_POINT('Ctrl Pts',(7.9295530816775,8.26849188852043,-15.1875542054435));
#36651=CARTESIAN_POINT('Ctrl Pts',(49.9530904856153,13.6252616883324,-9.01825571656003));
#36652=CARTESIAN_POINT('Ctrl Pts',(49.6498521530964,13.5952855444977,-9.30614285476429));
#36653=CARTESIAN_POINT('Ctrl Pts',(49.3404326906899,13.5655149131873,-9.58981807772683));
#36654=CARTESIAN_POINT('Ctrl Pts',(47.9977231570628,13.4398628522405,-10.7780905257659));
#36655=CARTESIAN_POINT('Ctrl Pts',(45.8662585664357,13.2576618204372,-12.4558237781188));
#36656=CARTESIAN_POINT('Ctrl Pts',(42.474764561552,13.0115743729063,-14.5523271530002));
#36657=CARTESIAN_POINT('Ctrl Pts',(38.3350016346459,12.751644575675,-16.5089212299443));
#36658=CARTESIAN_POINT('Ctrl Pts',(34.0211144068637,12.5189796899122,-17.8548947174334));
#36659=CARTESIAN_POINT('Ctrl Pts',(29.615209004902,12.301865256328,-18.5920822373384));
#36660=CARTESIAN_POINT('Ctrl Pts',(25.1795213846675,12.0904144587841,-18.8434107242654));
#36661=CARTESIAN_POINT('Ctrl Pts',(20.7614048765242,11.8774764455751,-18.4889962355741));
#36662=CARTESIAN_POINT('Ctrl Pts',(16.4430392282013,11.6504923923572,-17.5316024294851));
#36663=CARTESIAN_POINT('Ctrl Pts',(12.8475180499629,11.4410171343385,-16.2989298354701));
#36664=CARTESIAN_POINT('Ctrl Pts',(10.5461259110488,11.2882220371981,-15.2034411599271));
#36665=CARTESIAN_POINT('Ctrl Pts',(9.06993062890748,11.1823584691134,-14.3920548118685));
#36666=CARTESIAN_POINT('Ctrl Pts',(8.71849421176945,11.1565388193505,-14.1903535125101));
#36667=CARTESIAN_POINT('Ctrl Pts',(8.37137676108469,11.1304479812224,-13.982592023269));
#36668=CARTESIAN_POINT('Ctrl Pts',(50.8248043471025,15.9398275064074,-5.03469583101935));
#36669=CARTESIAN_POINT('Ctrl Pts',(50.531689720598,15.9092719019138,-5.34176956106061));
#36670=CARTESIAN_POINT('Ctrl Pts',(50.2322216993377,15.8789225535602,-5.64495084018071));
#36671=CARTESIAN_POINT('Ctrl Pts',(48.9310805715447,15.7507918597713,-6.91759254606773));
#36672=CARTESIAN_POINT('Ctrl Pts',(46.856540968822,15.5646999212503,-8.72905784910073));
#36673=CARTESIAN_POINT('Ctrl Pts',(43.5293146351041,15.3133344724918,-11.0383768254307));
#36674=CARTESIAN_POINT('Ctrl Pts',(39.4386131135355,15.0487502016962,-13.2554538905063));
#36675=CARTESIAN_POINT('Ctrl Pts',(35.1398025651756,14.8142492774957,-14.8745682218989));
#36676=CARTESIAN_POINT('Ctrl Pts',(30.7126367899701,14.5991383033468,-15.8936292613155));
#36677=CARTESIAN_POINT('Ctrl Pts',(26.225383041263,14.3930646018661,-16.4317101448757));
#36678=CARTESIAN_POINT('Ctrl Pts',(21.7162835651667,14.1899609567462,-16.3675092373584));
#36679=CARTESIAN_POINT('Ctrl Pts',(17.26525500769,13.977122935371,-15.6998422171581));
#36680=CARTESIAN_POINT('Ctrl Pts',(13.5264251178423,13.7824369346935,-14.713381358643));
#36681=CARTESIAN_POINT('Ctrl Pts',(11.1090908355661,13.6409944051188,-13.7794319835509));
#36682=CARTESIAN_POINT('Ctrl Pts',(9.54958799636594,13.5429643472183,-13.0732079429502));
#36683=CARTESIAN_POINT('Ctrl Pts',(9.17748643978684,13.5190447294408,-12.8966048355516));
#36684=CARTESIAN_POINT('Ctrl Pts',(8.80912250506288,13.4948677704672,-12.7136870295246));
#36685=CARTESIAN_POINT('Ctrl Pts',(51.8622440502334,18.188947172369,-0.289545832901423));
#36686=CARTESIAN_POINT('Ctrl Pts',(51.5807701807973,18.1597316481657,-0.618456087500125));
#36687=CARTESIAN_POINT('Ctrl Pts',(51.2927600533601,18.1307342364494,-0.943805954907987));
#36688=CARTESIAN_POINT('Ctrl Pts',(50.0395554717762,18.0083786966032,-2.31220075101254));
#36689=CARTESIAN_POINT('Ctrl Pts',(48.0307425794066,17.830846834045,-4.27543281823846));
#36690=CARTESIAN_POINT('Ctrl Pts',(44.778002741115,17.5925027676131,-6.82619040609315));
#36691=CARTESIAN_POINT('Ctrl Pts',(40.7446169869983,17.3443426911773,-9.33864581572932));
#36692=CARTESIAN_POINT('Ctrl Pts',(36.4643204356845,17.1289494695207,-11.2672600886416));
#36693=CARTESIAN_POINT('Ctrl Pts',(32.0141683740696,16.9369213116231,-12.6053959862687));
#36694=CARTESIAN_POINT('Ctrl Pts',(27.4693092848983,16.7575317657622,-13.4677724902511));
#36695=CARTESIAN_POINT('Ctrl Pts',(22.8575688046928,16.5859876106103,-13.7313406272161));
#36696=CARTESIAN_POINT('Ctrl Pts',(18.2562644932297,16.4095763329362,-13.3903470280312));
#36697=CARTESIAN_POINT('Ctrl Pts',(14.3547946342421,16.2491906636996,-12.6810668013076));
#36698=CARTESIAN_POINT('Ctrl Pts',(11.8057078793454,16.1323920433636,-11.9286495487117));
#36699=CARTESIAN_POINT('Ctrl Pts',(10.1514883569898,16.0510402241362,-11.3404810809659));
#36700=CARTESIAN_POINT('Ctrl Pts',(9.75597558972479,16.0311583490605,-11.1921012097805));
#36701=CARTESIAN_POINT('Ctrl Pts',(9.36361992511381,16.01103806515,-11.0371697661498));
#36702=CARTESIAN_POINT('Ctrl Pts',(52.8005712434362,19.7983627848149,4.00856019691356));
#36703=CARTESIAN_POINT('Ctrl Pts',(52.5293769678043,19.7720645135703,3.66073478500352));
#36704=CARTESIAN_POINT('Ctrl Pts',(52.2514949487339,19.7460021313493,3.31620884467359));
#36705=CARTESIAN_POINT('Ctrl Pts',(51.0407143360908,19.6361820466171,1.86509964359795));
#36706=CARTESIAN_POINT('Ctrl Pts',(49.0901569813625,19.4774394485581,-0.229263744330297));
#36707=CARTESIAN_POINT('Ctrl Pts',(45.9037408638273,19.2670183310104,-2.98866537396808));
#36708=CARTESIAN_POINT('Ctrl Pts',(41.9218786695201,19.0520629838802,-5.75635326875137));
#36709=CARTESIAN_POINT('Ctrl Pts',(37.6591904462393,18.8717166252608,-7.95229818907755));
#36710=CARTESIAN_POINT('Ctrl Pts',(33.1903616902194,18.7178122962125,-9.5658253198722));
#36711=CARTESIAN_POINT('Ctrl Pts',(28.5965511857935,18.5794411422907,-10.707876735862));
#36712=CARTESIAN_POINT('Ctrl Pts',(23.8964674609503,18.4529446490623,-11.2537653259037));
#36713=CARTESIAN_POINT('Ctrl Pts',(19.1651429878408,18.3257380682571,-11.1936823159398));
#36714=CARTESIAN_POINT('Ctrl Pts',(15.1226214079936,18.2102139945187,-10.7223744229274));
#36715=CARTESIAN_POINT('Ctrl Pts',(12.4590849026629,18.1249152482566,-10.125515214314));
#36716=CARTESIAN_POINT('Ctrl Pts',(10.7225346207661,18.064727637235,-9.63839747515494));
#36717=CARTESIAN_POINT('Ctrl Pts',(10.3067513445607,18.0499634327475,-9.51419720566911));
#36718=CARTESIAN_POINT('Ctrl Pts',(9.89369712912435,18.0349776243875,-9.38326573097788));
#36719=CARTESIAN_POINT('Ctrl Pts',(53.4863370250255,20.6836496418694,7.15694860497204));
#36720=CARTESIAN_POINT('Ctrl Pts',(53.2225809627893,20.6606519170286,6.79587106594126));
#36721=CARTESIAN_POINT('Ctrl Pts',(52.952032742616,20.6379063239872,6.43792468941075));
#36722=CARTESIAN_POINT('Ctrl Pts',(51.7719980977726,20.5422448076096,4.92898918929371));
#36723=CARTESIAN_POINT('Ctrl Pts',(49.8637381959815,20.4047755971079,2.74288789221826));
#36724=CARTESIAN_POINT('Ctrl Pts',(46.7257495251636,20.225761668211,-0.162608626170642));
#36725=CARTESIAN_POINT('Ctrl Pts',(42.7819444547883,20.0475517349526,-3.10909821565097));
#36726=CARTESIAN_POINT('Ctrl Pts',(38.5331171200345,19.9048724048602,-5.49235143170712));
#36727=CARTESIAN_POINT('Ctrl Pts',(34.0522545486923,19.790507905872,-7.29876156315941));
#36728=CARTESIAN_POINT('Ctrl Pts',(29.4248004114224,19.6935273080542,-8.63658437963781));
#36729=CARTESIAN_POINT('Ctrl Pts',(24.6629501157001,19.6110850660289,-9.37988832701164));
#36730=CARTESIAN_POINT('Ctrl Pts',(19.8400964602983,19.530779076001,-9.51591962186098));
#36731=CARTESIAN_POINT('Ctrl Pts',(15.697975272498,19.4573327991495,-9.21047942885606));
#36732=CARTESIAN_POINT('Ctrl Pts',(12.9534550617257,19.4012238336331,-8.72182627864199));
#36733=CARTESIAN_POINT('Ctrl Pts',(11.1586004449949,19.3605693891818,-8.30491329803392));
#36734=CARTESIAN_POINT('Ctrl Pts',(10.7285107947356,19.3505226070412,-8.19751403024314));
#36735=CARTESIAN_POINT('Ctrl Pts',(10.3008944253755,19.3402634731691,-8.08326215051905));
#36736=CARTESIAN_POINT('Ctrl Pts',(53.8717271214901,21.117312799858,8.92829900095583));
#36737=CARTESIAN_POINT('Ctrl Pts',(53.6121489835061,21.0964267127388,8.55989544261294));
#36738=CARTESIAN_POINT('Ctrl Pts',(53.3457209337029,21.0758020890032,8.19453489651512));
#36739=CARTESIAN_POINT('Ctrl Pts',(52.1829645833057,20.9891913310095,6.6536739220593));
#36740=CARTESIAN_POINT('Ctrl Pts',(50.2984941161407,20.8653273744228,4.41690405101842));
#36741=CARTESIAN_POINT('Ctrl Pts',(47.1878108923031,20.7063681300896,1.43067040790121));
#36742=CARTESIAN_POINT('Ctrl Pts',(43.2655731566299,20.5515335415639,-1.6146666396427));
#36743=CARTESIAN_POINT('Ctrl Pts',(39.0248124328953,20.4326519806542,-4.10149377374684));
#36744=CARTESIAN_POINT('Ctrl Pts',(34.5375663594191,20.3430531321453,-6.01455607201149));
#36745=CARTESIAN_POINT('Ctrl Pts',(29.8916687633621,20.2718184169426,-7.46061039168494));
#36746=CARTESIAN_POINT('Ctrl Pts',(25.095679036358,20.2165549432469,-8.31301457851303));
#36747=CARTESIAN_POINT('Ctrl Pts',(20.222073018947,20.164982094833,-8.55735906158925));
#36748=CARTESIAN_POINT('Ctrl Pts',(16.0246456841948,20.117197691553,-8.34346646267442));
#36749=CARTESIAN_POINT('Ctrl Pts',(13.2351131391784,20.0788282397779,-7.91448534989634));
#36750=CARTESIAN_POINT('Ctrl Pts',(11.4078395864424,20.0500302875854,-7.53626778012411));
#36751=CARTESIAN_POINT('Ctrl Pts',(10.9698103207056,20.0428451797642,-7.43812761261326));
#36752=CARTESIAN_POINT('Ctrl Pts',(10.5341268922228,20.0354515632684,-7.33306706741316));
#36753=CARTESIAN_POINT('Ctrl Pts',(53.9812860025028,21.2334813897109,9.43208375200366));
#36754=CARTESIAN_POINT('Ctrl Pts',(53.722894343233,21.2132228077857,9.06160546170904));
#36755=CARTESIAN_POINT('Ctrl Pts',(53.457636234034,21.1932283095702,8.69414579528152));
#36756=CARTESIAN_POINT('Ctrl Pts',(52.2997857115371,21.1093059289188,7.14424851817797));
#36757=CARTESIAN_POINT('Ctrl Pts',(50.4220705832473,20.9894835119608,4.89313906637515));
#36758=CARTESIAN_POINT('Ctrl Pts',(47.3191460135461,20.8364792943525,1.88406529232576));
#36759=CARTESIAN_POINT('Ctrl Pts',(43.4030459066543,20.6885792302246,-1.18922048567419));
#36760=CARTESIAN_POINT('Ctrl Pts',(39.1646030660498,20.5767478260626,-3.70530894006767));
#36761=CARTESIAN_POINT('Ctrl Pts',(34.675589875711,20.4944756050622,-5.64847247317747));
#36762=CARTESIAN_POINT('Ctrl Pts',(30.0245195766032,20.4308554028779,-7.12504250766887));
#36763=CARTESIAN_POINT('Ctrl Pts',(25.2189244368836,20.3836340081555,-8.00816612769719));
#36764=CARTESIAN_POINT('Ctrl Pts',(20.3310177005882,20.340580727313,-8.28296238675351));
#36765=CARTESIAN_POINT('Ctrl Pts',(16.1179909263383,20.3004356869138,-8.09477141097565));
#36766=CARTESIAN_POINT('Ctrl Pts',(13.3157463284093,20.2673681898868,-7.682522571651));
#36767=CARTESIAN_POINT('Ctrl Pts',(11.4793096661362,20.2421246596599,-7.31514879108788));
#36768=CARTESIAN_POINT('Ctrl Pts',(11.0390389775994,20.2357981340653,-7.21960298661229));
#36769=CARTESIAN_POINT('Ctrl Pts',(10.6010806842436,20.2292648564311,-7.11711746623022));
#36770=CARTESIAN_POINT('Ctrl Pts',(54.0911200992672,21.3428689572265,9.93733722545763));
#36771=CARTESIAN_POINT('Ctrl Pts',(53.8339160771895,21.323266505305,9.56478777996708));
#36772=CARTESIAN_POINT('Ctrl Pts',(53.5698289525631,21.303930781031,9.1952328547344));
#36773=CARTESIAN_POINT('Ctrl Pts',(52.4168883164214,21.2228186866547,7.63631699932278));
#36774=CARTESIAN_POINT('Ctrl Pts',(50.5459347798675,21.1072213437662,5.37089768690188));
#36775=CARTESIAN_POINT('Ctrl Pts',(47.4507803460891,20.9604400919523,2.33903941389612));
#36776=CARTESIAN_POINT('Ctrl Pts',(43.5408353390201,20.819779963638,-0.762113079351122));
#36777=CARTESIAN_POINT('Ctrl Pts',(39.3047370968672,20.7152993064879,-3.30735423302198));
#36778=CARTESIAN_POINT('Ctrl Pts',(34.8139967414564,20.6406553883908,-5.28047852159549));
#36779=CARTESIAN_POINT('Ctrl Pts',(30.1578084903746,20.5849601975755,-6.78739123617449));
#36780=CARTESIAN_POINT('Ctrl Pts',(25.342681856911,20.5461109852346,-7.70101963370857));
#36781=CARTESIAN_POINT('Ctrl Pts',(20.4405655462474,20.5119420676311,-8.00600926239656));
#36782=CARTESIAN_POINT('Ctrl Pts',(16.212024900435,20.4797911688045,-7.84326492086165));
#36783=CARTESIAN_POINT('Ctrl Pts',(13.3971231763776,20.4522911786996,-7.44756158079435));
#36784=CARTESIAN_POINT('Ctrl Pts',(11.5515559411525,20.4307901345004,-7.09090367684731));
#36785=CARTESIAN_POINT('Ctrl Pts',(11.1090536044908,20.4253683033402,-6.99792131334964));
#36786=CARTESIAN_POINT('Ctrl Pts',(10.6688320741027,20.4197421663948,-6.89797979485316));
#36787=CARTESIAN_POINT('',(46.8667964697728,20.5529756002067,0.877339649208841));
#36788=CARTESIAN_POINT('Ctrl Pts',(36.2576800729436,-3.27137127985418,-29.7093682737774));
#36789=CARTESIAN_POINT('Ctrl Pts',(38.8712563024324,1.76302065360657,-26.519728653349));
#36790=CARTESIAN_POINT('Ctrl Pts',(41.7528145455644,6.26298702224536,-22.1049479564332));
#36791=CARTESIAN_POINT('Ctrl Pts',(44.8544505987311,12.5188402724798,-13.9136701764686));
#36792=CARTESIAN_POINT('Ctrl Pts',(45.663807377154,14.4577038717083,-11.0195527891233));
#36793=CARTESIAN_POINT('Ctrl Pts',(46.6763124148208,17.8486374263941,-5.17928678953648));
#36794=CARTESIAN_POINT('Ctrl Pts',(46.9241791761197,19.3555632898772,-2.18801330074644));
#36795=CARTESIAN_POINT('Ctrl Pts',(46.8667964697728,20.5529756002057,0.877339649209231));
#36796=CARTESIAN_POINT('Ctrl Pts',(18.6922256707601,19.9464420456703,-8.75371524283479));
#36797=CARTESIAN_POINT('Ctrl Pts',(23.7687459556886,20.0189549105364,-8.95811201716394));
#36798=CARTESIAN_POINT('Ctrl Pts',(28.8732165143738,20.0954766247834,-8.18217898492732));
#36799=CARTESIAN_POINT('Ctrl Pts',(38.4807809072633,20.2752040736289,-4.89538748035974));
#36800=CARTESIAN_POINT('Ctrl Pts',(42.9847320388888,20.3824974081049,-2.38626645795844));
#36801=CARTESIAN_POINT('Ctrl Pts',(46.8667964697727,20.5529756002056,0.877339649208949));
#36802=CARTESIAN_POINT('Ctrl Pts',(53.2371989972853,20.9435908393615,7.71126064895046));
#36803=CARTESIAN_POINT('Ctrl Pts',(53.1446919057712,20.9358615047579,7.58646941752768));
#36804=CARTESIAN_POINT('Ctrl Pts',(53.0521848142571,20.9281321701544,7.4616781861049));
#36805=CARTESIAN_POINT('Ctrl Pts',(52.959677722743,20.9204028355509,7.33688695468212));
#36806=CARTESIAN_POINT('Ctrl Pts',(43.7089685713345,20.1474693751975,-5.14223618759627));
#36807=CARTESIAN_POINT('Ctrl Pts',(26.9145688537952,20.0812550388979,-11.2680756118925));
#36808=CARTESIAN_POINT('Ctrl Pts',(11.77453820435,19.8399463130827,-7.84596586922967));
#36809=CARTESIAN_POINT('Ctrl Pts',(53.2371847394383,20.9469886892296,7.71116661896362));
#36810=CARTESIAN_POINT('Ctrl Pts',(53.1446826144396,20.9392720585054,7.58636902784782));
#36811=CARTESIAN_POINT('Ctrl Pts',(53.0521804894409,20.9315554277811,7.46157143673202));
#36812=CARTESIAN_POINT('Ctrl Pts',(52.9596783644423,20.9238387970569,7.33677384561622));
#36813=CARTESIAN_POINT('Ctrl Pts',(43.7094658645762,20.1521757246323,-5.14298526596396));
#36814=CARTESIAN_POINT('Ctrl Pts',(26.9147671963741,20.0873688943554,-11.2684775349938));
#36815=CARTESIAN_POINT('Ctrl Pts',(11.7747583744327,19.8474084919615,-7.8466185942614));
#36816=CARTESIAN_POINT('Ctrl Pts',(53.2371704815913,20.9503865390978,7.71107258897678));
#36817=CARTESIAN_POINT('Ctrl Pts',(53.144673323108,20.9426826122528,7.58626863816796));
#36818=CARTESIAN_POINT('Ctrl Pts',(53.0521761646248,20.9349786854078,7.46146468735915));
#36819=CARTESIAN_POINT('Ctrl Pts',(52.9596790061415,20.9272747585629,7.33666073655033));
#36820=CARTESIAN_POINT('Ctrl Pts',(43.7099631578178,20.1568820740671,-5.14373434433165));
#36821=CARTESIAN_POINT('Ctrl Pts',(26.9149655389531,20.093482749813,-11.2688794580951));
#36822=CARTESIAN_POINT('Ctrl Pts',(11.7749785445154,19.8548706708402,-7.84727131929312));
#36823=CARTESIAN_POINT('Ctrl Pts',(53.2371562237442,20.9537843889659,7.71097855898994));
#36824=CARTESIAN_POINT('Ctrl Pts',(53.1446640317764,20.9460931660003,7.58616824848811));
#36825=CARTESIAN_POINT('Ctrl Pts',(53.0521718398086,20.9384019430346,7.46135793798627));
#36826=CARTESIAN_POINT('Ctrl Pts',(52.9596796478408,20.9307107200689,7.33654762748443));
#36827=CARTESIAN_POINT('Ctrl Pts',(43.7104604510594,20.1615884235019,-5.14448342269933));
#36828=CARTESIAN_POINT('Ctrl Pts',(26.915163881532,20.0995966052706,-11.2692813811964));
#36829=CARTESIAN_POINT('Ctrl Pts',(11.7751987145981,19.862332849719,-7.84792404432485));
#36830=CARTESIAN_POINT('Ctrl Pts',(53.2371129264224,20.9641027630587,7.71069301471406));
#36831=CARTESIAN_POINT('Ctrl Pts',(53.1446358164523,20.9564501184246,7.58586339150147));
#36832=CARTESIAN_POINT('Ctrl Pts',(53.0521587064822,20.9487974737906,7.46103376828889));
#36833=CARTESIAN_POINT('Ctrl Pts',(52.9596815965122,20.9411448291565,7.3362041450763));
#36834=CARTESIAN_POINT('Ctrl Pts',(43.7119705995062,20.1758803657488,-5.14675817618243));
#36835=CARTESIAN_POINT('Ctrl Pts',(26.9157661956446,20.1181627721728,-11.2705019156746));
#36836=CARTESIAN_POINT('Ctrl Pts',(11.7758673130841,19.8849935193208,-7.8499061981334));
#36837=CARTESIAN_POINT('Ctrl Pts',(53.2370263315175,20.9847395112521,7.71012192605225));
#36838=CARTESIAN_POINT('Ctrl Pts',(53.1445793856301,20.9771640232786,7.58525367745488));
#36839=CARTESIAN_POINT('Ctrl Pts',(53.0521324397426,20.9695885353052,7.4603854288575));
#36840=CARTESIAN_POINT('Ctrl Pts',(52.9596854938552,20.9620130473318,7.33551718026014));
#36841=CARTESIAN_POINT('Ctrl Pts',(43.7149909051107,20.2044642499886,-5.15130767947685));
#36842=CARTESIAN_POINT('Ctrl Pts',(26.916970820079,20.1552951062578,-11.2729429882015));
#36843=CARTESIAN_POINT('Ctrl Pts',(11.777204510056,19.9303148585245,-7.85387050575054));
#36844=CARTESIAN_POINT('Ctrl Pts',(53.2368964218958,21.0156946339229,7.70926528516895));
#36845=CARTESIAN_POINT('Ctrl Pts',(53.144494727887,21.0082348808134,7.58433910112455));
#36846=CARTESIAN_POINT('Ctrl Pts',(53.0520930338782,21.000775127704,7.45941291708015));
#36847=CARTESIAN_POINT('Ctrl Pts',(52.9596913398694,20.9933153745945,7.33448673303575));
#36848=CARTESIAN_POINT('Ctrl Pts',(43.7195219389881,20.2473400636495,-5.15813167140387));
#36849=CARTESIAN_POINT('Ctrl Pts',(26.9187775261177,20.2109936225946,-11.2766048230408));
#36850=CARTESIAN_POINT('Ctrl Pts',(11.779210305514,19.9982968673298,-7.85981696717621));
#36851=CARTESIAN_POINT('Ctrl Pts',(53.2367664895543,21.0466497571015,7.70840863393207));
#36852=CARTESIAN_POINT('Ctrl Pts',(53.1444100549975,21.0393057386868,7.58342451789186));
#36853=CARTESIAN_POINT('Ctrl Pts',(53.0520536204406,21.0319617202721,7.45844040185166));
#36854=CARTESIAN_POINT('Ctrl Pts',(52.9596971858838,21.0246177018574,7.33345628581145));
#36855=CARTESIAN_POINT('Ctrl Pts',(43.7240537302011,20.2902158603888,-5.16495531820909));
#36856=CARTESIAN_POINT('Ctrl Pts',(26.9205839257141,20.2666921589687,-11.2802669552304));
#36857=CARTESIAN_POINT('Ctrl Pts',(11.7812161009719,20.0662788761352,-7.86576342860189));
#36858=CARTESIAN_POINT('Ctrl Pts',(53.236679856522,21.0672865061488,7.70783752790633));
#36859=CARTESIAN_POINT('Ctrl Pts',(53.1443535987569,21.0600196441101,7.5828147922693));
#36860=CARTESIAN_POINT('Ctrl Pts',(53.0520273409918,21.0527527820714,7.45779205663226));
#36861=CARTESIAN_POINT('Ctrl Pts',(52.9597010832266,21.0454859200326,7.33276932099522));
#36862=CARTESIAN_POINT('Ctrl Pts',(43.7270753067131,20.3187997161584,-5.16950424270833));
#36863=CARTESIAN_POINT('Ctrl Pts',(26.9217880354578,20.3038245267329,-11.2827085269013));
#36864=CARTESIAN_POINT('Ctrl Pts',(11.7825532979438,20.1116002153389,-7.86972773621902));
#36865=CARTESIAN_POINT('Ctrl Pts',(53.236636539877,21.0776048806767,7.70755197484126));
#36866=CARTESIAN_POINT('Ctrl Pts',(53.1443253705507,21.0703765968246,7.58250992942321));
#36867=CARTESIAN_POINT('Ctrl Pts',(53.0520142012244,21.0631483129724,7.45746788400516));
#36868=CARTESIAN_POINT('Ctrl Pts',(52.9597030318981,21.0559200291202,7.33242583858711));
#36869=CARTESIAN_POINT('Ctrl Pts',(43.7285860992663,20.3330916439037,-5.17177870321784));
#36870=CARTESIAN_POINT('Ctrl Pts',(26.9223900882949,20.3223907107576,-11.2839293144965));
#36871=CARTESIAN_POINT('Ctrl Pts',(11.7832218964298,20.1342608849406,-7.87170989002758));
#36872=CARTESIAN_POINT('Ctrl Pts',(53.236632365876,21.0785991614118,7.70752445888798));
#36873=CARTESIAN_POINT('Ctrl Pts',(53.1443226504748,21.0713745949617,7.58248055277538));
#36874=CARTESIAN_POINT('Ctrl Pts',(53.0520129350737,21.0641500285117,7.45743664666278));
#36875=CARTESIAN_POINT('Ctrl Pts',(52.9597032196725,21.0569254620617,7.33239274055018));
#36876=CARTESIAN_POINT('Ctrl Pts',(43.7287316795538,20.3344688170607,-5.17199787070987));
#36877=CARTESIAN_POINT('Ctrl Pts',(26.9224481022327,20.3241797521467,-11.2840469498454));
#36878=CARTESIAN_POINT('Ctrl Pts',(11.7832863227202,20.1364444718193,-7.87190089078457));
#36879=CARTESIAN_POINT('Ctrl Pts',(53.236628191875,21.0795934421468,7.7074969429347));
#36880=CARTESIAN_POINT('Ctrl Pts',(53.144319930399,21.0723725930989,7.58245117612755));
#36881=CARTESIAN_POINT('Ctrl Pts',(53.0520116689229,21.0651517440511,7.4574054093204));
#36882=CARTESIAN_POINT('Ctrl Pts',(52.9597034074469,21.0579308950032,7.33235964251325));
#36883=CARTESIAN_POINT('Ctrl Pts',(43.7288772598413,20.3358459902176,-5.17221703820191));
#36884=CARTESIAN_POINT('Ctrl Pts',(26.9225061161704,20.3259687935359,-11.2841645851943));
#36885=CARTESIAN_POINT('Ctrl Pts',(11.7833507490106,20.1386280586979,-7.87209189154155));
#36886=CARTESIAN_POINT('Ctrl Pts',(53.236624017874,21.0805877228818,7.70746942698142));
#36887=CARTESIAN_POINT('Ctrl Pts',(53.1443172103231,21.0733705912361,7.58242179947972));
#36888=CARTESIAN_POINT('Ctrl Pts',(53.0520104027722,21.0661534595904,7.45737417197801));
#36889=CARTESIAN_POINT('Ctrl Pts',(52.9597035952212,21.0589363279447,7.33232654447631));
#36890=CARTESIAN_POINT('Ctrl Pts',(43.7290228401288,20.3372231633746,-5.17243620569395));
#36891=CARTESIAN_POINT('Ctrl Pts',(26.9225641301082,20.327757834925,-11.2842822205432));
#36892=CARTESIAN_POINT('Ctrl Pts',(11.783415175301,20.1408116455766,-7.87228289229854));
#36893=CARTESIAN_POINT('',(46.8667964697728,20.5529756002067,0.877339649208832));
#36894=CARTESIAN_POINT('Ctrl Pts',(25.9230198769569,21.2883239772394,48.5187615226217));
#36895=CARTESIAN_POINT('Ctrl Pts',(26.0539515103827,21.2711623310641,48.0878393189679));
#36896=CARTESIAN_POINT('Ctrl Pts',(26.1782967764799,21.2542807820542,47.6534307220407));
#36897=CARTESIAN_POINT('Ctrl Pts',(26.6802445993609,21.1834525291307,45.7852132990113));
#36898=CARTESIAN_POINT('Ctrl Pts',(27.288585715814,21.0834264338425,42.914751594488));
#36899=CARTESIAN_POINT('Ctrl Pts',(27.7344129255298,20.9598507183575,38.6101384297008));
#36900=CARTESIAN_POINT('Ctrl Pts',(27.7267262169894,20.8461335954997,33.6244561521861));
#36901=CARTESIAN_POINT('Ctrl Pts',(27.0801344432569,20.7684839093916,28.7282178850793));
#36902=CARTESIAN_POINT('Ctrl Pts',(25.8262070857061,20.7206230093664,23.987509714119));
#36903=CARTESIAN_POINT('Ctrl Pts',(24.1034285018224,20.6916936542703,19.4064911568363));
#36904=CARTESIAN_POINT('Ctrl Pts',(21.8159838238208,20.6796111419738,15.0691197456759));
#36905=CARTESIAN_POINT('Ctrl Pts',(18.9964020956871,20.6722203558656,11.0412903808993));
#36906=CARTESIAN_POINT('Ctrl Pts',(16.2297782829761,20.6630225594897,7.83114746321505));
#36907=CARTESIAN_POINT('Ctrl Pts',(14.1622593406336,20.6508204531822,5.87251256806097));
#36908=CARTESIAN_POINT('Ctrl Pts',(12.7321233110437,20.6394053700742,4.6502519272584));
#36909=CARTESIAN_POINT('Ctrl Pts',(12.3848420399471,20.6364191357732,4.36299885106413));
#36910=CARTESIAN_POINT('Ctrl Pts',(12.033600930572,20.6332209087108,4.0818235088649));
#36911=CARTESIAN_POINT('Ctrl Pts',(26.2604130869634,21.2398788304839,48.1049156951145));
#36912=CARTESIAN_POINT('Ctrl Pts',(26.3890228772049,21.2217224127637,47.6743582450841));
#36913=CARTESIAN_POINT('Ctrl Pts',(26.5110378923674,21.2038412173392,47.2403414023796));
#36914=CARTESIAN_POINT('Ctrl Pts',(27.0030058479278,21.1287309618461,45.3739126709932));
#36915=CARTESIAN_POINT('Ctrl Pts',(27.5961224061632,21.0222253289507,42.5070844035404));
#36916=CARTESIAN_POINT('Ctrl Pts',(28.0195357773322,20.8890564489947,38.2105610058552));
#36917=CARTESIAN_POINT('Ctrl Pts',(27.9864836476654,20.7641817659416,33.237344487507));
#36918=CARTESIAN_POINT('Ctrl Pts',(27.3158697008056,20.6752847595175,28.3572877847353));
#36919=CARTESIAN_POINT('Ctrl Pts',(26.0398030951076,20.6159219251614,23.6363760825188));
#36920=CARTESIAN_POINT('Ctrl Pts',(24.2966827408469,20.5752144761384,19.0779816153495));
#36921=CARTESIAN_POINT('Ctrl Pts',(21.991500040255,20.5509334123338,14.7667026515359));
#36922=CARTESIAN_POINT('Ctrl Pts',(19.1573179832986,20.5308579865904,10.7683362842277));
#36923=CARTESIAN_POINT('Ctrl Pts',(16.3805824951291,20.510426256151,7.58571157269837));
#36924=CARTESIAN_POINT('Ctrl Pts',(14.3080816454852,20.4905046142392,5.64691895319579));
#36925=CARTESIAN_POINT('Ctrl Pts',(12.8753010992689,20.4739374093561,4.43819828994725));
#36926=CARTESIAN_POINT('Ctrl Pts',(12.5274194918876,20.469713411733,4.15420637215013));
#36927=CARTESIAN_POINT('Ctrl Pts',(12.1756128765411,20.4652767483487,3.87630351967435));
#36928=CARTESIAN_POINT('Ctrl Pts',(26.5978977585567,21.1822016013635,47.6908646032478));
#36929=CARTESIAN_POINT('Ctrl Pts',(26.7241687502308,21.1630886105529,47.2606817005154));
#36930=CARTESIAN_POINT('Ctrl Pts',(26.8438362667628,21.1442460408093,46.827066958471));
#36931=CARTESIAN_POINT('Ctrl Pts',(27.3257495502969,21.0650173413637,44.9624735955608));
#36932=CARTESIAN_POINT('Ctrl Pts',(27.9035295741986,20.9522796229575,42.0993524422593));
#36933=CARTESIAN_POINT('Ctrl Pts',(28.3043662171167,20.8098799445818,37.8110397719833));
#36934=CARTESIAN_POINT('Ctrl Pts',(28.2457618908011,20.6742608619688,32.8504467932067));
#36935=CARTESIAN_POINT('Ctrl Pts',(27.5509398519194,20.5745198093833,27.9867571563878));
#36936=CARTESIAN_POINT('Ctrl Pts',(26.2525464356161,20.5040526001987,23.2858628858746));
#36937=CARTESIAN_POINT('Ctrl Pts',(24.4888919980713,20.4519664047462,18.7503504098016));
#36938=CARTESIAN_POINT('Ctrl Pts',(22.1657719532826,20.4158956934967,14.4654712264667));
#36939=CARTESIAN_POINT('Ctrl Pts',(19.316780166669,20.3835681705302,10.496928045425));
#36940=CARTESIAN_POINT('Ctrl Pts',(16.5297402438784,20.3523071857454,7.34216931551517));
#36941=CARTESIAN_POINT('Ctrl Pts',(14.4521203095409,20.3249607749065,5.42346942398235));
#36942=CARTESIAN_POINT('Ctrl Pts',(13.0166006108032,20.3034475984546,4.22845797086557));
#36943=CARTESIAN_POINT('Ctrl Pts',(12.6680970903426,20.2980359714688,3.9477695260792));
#36944=CARTESIAN_POINT('Ctrl Pts',(12.3157045007277,20.29241155197,3.67318310060867));
#36945=CARTESIAN_POINT('Ctrl Pts',(27.8042303352092,20.942701117012,46.2104819450654));
#36946=CARTESIAN_POINT('Ctrl Pts',(27.9220864002744,20.9203083949833,45.7816721251138));
#36947=CARTESIAN_POINT('Ctrl Pts',(28.0333058486476,20.898168919688,45.3495315848581));
#36948=CARTESIAN_POINT('Ctrl Pts',(28.479027267791,20.8048139743737,43.4916681867343));
#36949=CARTESIAN_POINT('Ctrl Pts',(29.001609853494,20.6706999592586,40.6420644930631));
#36950=CARTESIAN_POINT('Ctrl Pts',(29.321194751232,20.496623371127,36.3835358770081));
#36951=CARTESIAN_POINT('Ctrl Pts',(29.1706179809275,20.3241023157428,31.4686302216622));
#36952=CARTESIAN_POINT('Ctrl Pts',(28.3886246832073,20.1870685788371,26.664106447373));
#36953=CARTESIAN_POINT('Ctrl Pts',(27.0097717402225,20.0783595881962,22.0355517219541));
#36954=CARTESIAN_POINT('Ctrl Pts',(25.1720430323228,19.9870599496472,17.5827492484273));
#36955=CARTESIAN_POINT('Ctrl Pts',(22.7840975954265,19.9103458023656,13.3933296353274));
#36956=CARTESIAN_POINT('Ctrl Pts',(19.8814149628274,19.8358125374395,9.53266872594138));
#36957=CARTESIAN_POINT('Ctrl Pts',(17.0568419677846,19.767331746443,6.47874833434411));
#36958=CARTESIAN_POINT('Ctrl Pts',(14.9604215493633,19.7145309927478,4.63275273616586));
#36959=CARTESIAN_POINT('Ctrl Pts',(13.5147630489044,19.6760973304852,3.48733920738447));
#36960=CARTESIAN_POINT('Ctrl Pts',(13.1639588284761,19.6666248028076,3.21861022039478));
#36961=CARTESIAN_POINT('Ctrl Pts',(12.809399673684,19.6569408091057,2.95603772191131));
#36962=CARTESIAN_POINT('Ctrl Pts',(29.521986074236,20.4780024533914,44.1011384618627));
#36963=CARTESIAN_POINT('Ctrl Pts',(29.6276533884862,20.4514551579611,43.6744145807348));
#36964=CARTESIAN_POINT('Ctrl Pts',(29.7266308829499,20.4251375618498,43.2445117569686));
#36965=CARTESIAN_POINT('Ctrl Pts',(30.1198857679885,20.3138746691076,41.3968573299702));
#36966=CARTESIAN_POINT('Ctrl Pts',(30.5624530626371,20.1526659052326,38.5675133009135));
#36967=CARTESIAN_POINT('Ctrl Pts',(30.7642453491852,19.938389785095,34.3530777137597));
#36968=CARTESIAN_POINT('Ctrl Pts',(30.4803031817061,19.7189203495023,29.5053887059681));
#36969=CARTESIAN_POINT('Ctrl Pts',(29.5718411556588,19.5342279169114,24.7875278899887));
#36970=CARTESIAN_POINT('Ctrl Pts',(28.0761487535003,19.3763677050182,20.2646564748078));
#36971=CARTESIAN_POINT('Ctrl Pts',(26.1307371975581,19.2344308170631,15.9325175110228));
#36972=CARTESIAN_POINT('Ctrl Pts',(23.6483675649021,19.1049298841923,11.88218726952));
#36973=CARTESIAN_POINT('Ctrl Pts',(20.667216710507,18.9752993129734,8.17858276534581));
#36974=CARTESIAN_POINT('Ctrl Pts',(17.7875458146746,18.8580619466085,5.27139096265361));
#36975=CARTESIAN_POINT('Ctrl Pts',(15.6633058517737,18.7718242877839,3.53114688412792));
#36976=CARTESIAN_POINT('Ctrl Pts',(14.2025389775091,18.7111415689428,2.45786531596827));
#36977=CARTESIAN_POINT('Ctrl Pts',(13.8483121118092,18.6963263828107,2.2065451923323));
#36978=CARTESIAN_POINT('Ctrl Pts',(13.4905360193496,18.6812985797984,1.96147587216487));
#36979=CARTESIAN_POINT('Ctrl Pts',(32.0272347697465,19.4355555088431,41.0215590310772));
#36980=CARTESIAN_POINT('Ctrl Pts',(32.1144819741636,19.4044605226273,40.5982064715866));
#36981=CARTESIAN_POINT('Ctrl Pts',(32.1949477980604,19.3735658358572,40.1719179195087));
#36982=CARTESIAN_POINT('Ctrl Pts',(32.5088196418466,19.2426748194849,38.3407454628268));
#36983=CARTESIAN_POINT('Ctrl Pts',(32.8303234267137,19.0517849995255,35.5435871503504));
#36984=CARTESIAN_POINT('Ctrl Pts',(32.853854400985,18.7933185397158,31.3980268277304));
#36985=CARTESIAN_POINT('Ctrl Pts',(32.3679847439182,18.5218580841843,26.6544248517635));
#36986=CARTESIAN_POINT('Ctrl Pts',(31.2678462688368,18.2836948825759,22.0699343228032));
#36987=CARTESIAN_POINT('Ctrl Pts',(29.594773201358,18.0697821020849,17.7091129242814));
#36988=CARTESIAN_POINT('Ctrl Pts',(27.4855694135664,17.8693333343866,13.5616312265872));
#36989=CARTESIAN_POINT('Ctrl Pts',(24.8590776326079,17.6778661310593,9.72378981616505));
#36990=CARTESIAN_POINT('Ctrl Pts',(21.757468922915,17.4826662284719,6.25984891758698));
#36991=CARTESIAN_POINT('Ctrl Pts',(18.7925807133286,17.3068805329357,3.57641430602537));
#36992=CARTESIAN_POINT('Ctrl Pts',(16.6247429863748,17.1802068447994,1.99736191703145));
#36993=CARTESIAN_POINT('Ctrl Pts',(15.1400283234621,17.0925519552341,1.03400839035698));
#36994=CARTESIAN_POINT('Ctrl Pts',(14.7803936608885,17.0712544126695,0.809254098100135));
#36995=CARTESIAN_POINT('Ctrl Pts',(14.417553197045,17.0497370990139,0.590927633578045));
#36996=CARTESIAN_POINT('Ctrl Pts',(34.8534706325002,17.8320672383652,37.5445499124197));
#36997=CARTESIAN_POINT('Ctrl Pts',(34.9191540130177,17.7976045693245,37.1253023664157));
#36998=CARTESIAN_POINT('Ctrl Pts',(34.9779337159588,17.7633163796081,36.7034247748685));
#36999=CARTESIAN_POINT('Ctrl Pts',(35.1987483607876,17.6178640028275,34.8924120264708));
#37000=CARTESIAN_POINT('Ctrl Pts',(35.3783275375406,17.4049846203341,32.1342451211723));
#37001=CARTESIAN_POINT('Ctrl Pts',(35.1928167690002,17.1135517229592,28.071271996886));
#37002=CARTESIAN_POINT('Ctrl Pts',(34.4700307079904,16.8027253827761,23.4518154045472));
#37003=CARTESIAN_POINT('Ctrl Pts',(33.1447876860525,16.523022337621,19.0257930993187));
#37004=CARTESIAN_POINT('Ctrl Pts',(31.2630832463472,16.2641978724915,14.8570951032009));
#37005=CARTESIAN_POINT('Ctrl Pts',(28.9609075929285,16.0157341831644,10.9282861435268));
#37006=CARTESIAN_POINT('Ctrl Pts',(26.164113782871,15.7719994721116,7.34182712399574));
#37007=CARTESIAN_POINT('Ctrl Pts',(22.9194789776465,15.5202180684676,4.16124318963596));
#37008=CARTESIAN_POINT('Ctrl Pts',(19.852782333304,15.2931736272884,1.74227197016013));
#37009=CARTESIAN_POINT('Ctrl Pts',(17.6323041133784,15.130708702949,0.353694351278024));
#37010=CARTESIAN_POINT('Ctrl Pts',(16.118415924838,15.0190926843839,-0.479769477849797));
#37011=CARTESIAN_POINT('Ctrl Pts',(15.7522333195276,14.9920326361705,-0.673092285248657));
#37012=CARTESIAN_POINT('Ctrl Pts',(15.3833028254314,14.9647422323135,-0.859739042833271));
#37013=CARTESIAN_POINT('Ctrl Pts',(37.542377320307,15.7638142683891,34.2340379990305));
#37014=CARTESIAN_POINT('Ctrl Pts',(37.5864967275411,15.7283726072843,33.8189895177017));
#37015=CARTESIAN_POINT('Ctrl Pts',(37.623576054751,15.6930928161318,33.4016424442209));
#37016=CARTESIAN_POINT('Ctrl Pts',(37.751216544469,15.543379415412,31.6114150579845));
#37017=CARTESIAN_POINT('Ctrl Pts',(37.7886730339078,15.3241289383934,28.8932275168839));
#37018=CARTESIAN_POINT('Ctrl Pts',(37.3937306124187,15.0227233638938,24.9144383133945));
#37019=CARTESIAN_POINT('Ctrl Pts',(36.4334261401257,14.6988957424381,20.4211498872596));
#37020=CARTESIAN_POINT('Ctrl Pts',(34.8822465580896,14.4035050799014,16.155848302069));
#37021=CARTESIAN_POINT('Ctrl Pts',(32.7907838851794,14.1252237593235,12.1817954315162));
#37022=CARTESIAN_POINT('Ctrl Pts',(30.2942408069272,13.8539516979883,8.47441520091897));
#37023=CARTESIAN_POINT('Ctrl Pts',(27.32537306915,13.5829362127958,5.14241023042879));
#37024=CARTESIAN_POINT('Ctrl Pts',(23.9355050652897,13.2994842764397,2.24860259607305));
#37025=CARTESIAN_POINT('Ctrl Pts',(20.764783485743,13.0425486753816,0.0972780310443223));
#37026=CARTESIAN_POINT('Ctrl Pts',(18.4899534807288,12.8585920936854,-1.09852526744414));
#37027=CARTESIAN_POINT('Ctrl Pts',(16.9456836958165,12.7324540777387,-1.80052542287351));
#37028=CARTESIAN_POINT('Ctrl Pts',(16.5727366200309,12.7018988467546,-1.96200324615093));
#37029=CARTESIAN_POINT('Ctrl Pts',(16.1975722418824,12.6711030837425,-2.11652390033856));
#37030=CARTESIAN_POINT('Ctrl Pts',(40.0687256573802,13.2592937677246,31.1228441461166));
#37031=CARTESIAN_POINT('Ctrl Pts',(40.0914257254572,13.2252177231213,30.7119049446456));
#37032=CARTESIAN_POINT('Ctrl Pts',(40.1069388012238,13.191306123502,30.2990220397433));
#37033=CARTESIAN_POINT('Ctrl Pts',(40.141937508551,13.0474600457288,28.5294034284981));
#37034=CARTESIAN_POINT('Ctrl Pts',(40.038048613647,12.8372075593629,25.8509681782089));
#37035=CARTESIAN_POINT('Ctrl Pts',(39.4346952432425,12.5484949329477,21.9561736216729));
#37036=CARTESIAN_POINT('Ctrl Pts',(38.2378601831066,12.2377054846042,17.5890305686027));
#37037=CARTESIAN_POINT('Ctrl Pts',(36.4614388310332,11.9522310106351,13.4846984409205));
#37038=CARTESIAN_POINT('Ctrl Pts',(34.160565676204,11.6797819251771,9.70584142430889));
#37039=CARTESIAN_POINT('Ctrl Pts',(31.4696986733579,11.4108111467242,6.22069601970489));
#37040=CARTESIAN_POINT('Ctrl Pts',(28.3283877321082,11.1374939458242,3.1442866710006));
#37041=CARTESIAN_POINT('Ctrl Pts',(24.7924587223825,10.8473681096278,0.538753743941756));
#37042=CARTESIAN_POINT('Ctrl Pts',(21.5166685226697,10.5820480444149,-1.3433864264039));
#37043=CARTESIAN_POINT('Ctrl Pts',(19.1865556611937,10.3910369789073,-2.34521593896695));
#37044=CARTESIAN_POINT('Ctrl Pts',(17.6112105856552,10.2599216927486,-2.91490446819573));
#37045=CARTESIAN_POINT('Ctrl Pts',(17.2314099331844,10.2281653805015,-3.04431791604507));
#37046=CARTESIAN_POINT('Ctrl Pts',(16.8499985273585,10.1961599190035,-3.1664797330386));
#37047=CARTESIAN_POINT('Ctrl Pts',(42.4513879531089,10.420684636249,28.1887961890181));
#37048=CARTESIAN_POINT('Ctrl Pts',(42.4528615514467,10.3898269637342,27.7817853751185));
#37049=CARTESIAN_POINT('Ctrl Pts',(42.4469943536053,10.3591499865554,27.3732089758612));
#37050=CARTESIAN_POINT('Ctrl Pts',(42.3901211918335,10.2291883131935,25.6236312047506));
#37051=CARTESIAN_POINT('Ctrl Pts',(42.1460260161208,10.0401067219452,22.984119835829));
#37052=CARTESIAN_POINT('Ctrl Pts',(41.3358278887554,9.78206378055234,19.1722162135672));
#37053=CARTESIAN_POINT('Ctrl Pts',(39.9040992893687,9.50499638561923,14.9301076971436));
#37054=CARTESIAN_POINT('Ctrl Pts',(37.9038077627142,9.24981780003299,10.9858713610508));
#37055=CARTESIAN_POINT('Ctrl Pts',(35.394592979796,9.00337535985762,7.40159323672565));
#37056=CARTESIAN_POINT('Ctrl Pts',(32.5102108332376,8.75677479408939,4.13827932323636));
#37057=CARTESIAN_POINT('Ctrl Pts',(29.1969188360728,8.50116890088297,1.31733874904121));
#37058=CARTESIAN_POINT('Ctrl Pts',(25.5150150389335,8.22444592813344,-0.999758566332292));
#37059=CARTESIAN_POINT('Ctrl Pts',(22.1339602470639,7.96804930448713,-2.61237505739787));
#37060=CARTESIAN_POINT('Ctrl Pts',(19.7482465529448,7.78162503245108,-3.4198681063926));
#37061=CARTESIAN_POINT('Ctrl Pts',(18.1415532826121,7.65323614745839,-3.85696102050637));
#37062=CARTESIAN_POINT('Ctrl Pts',(17.7549106912631,7.62212996336316,-3.95424830145647));
#37063=CARTESIAN_POINT('Ctrl Pts',(17.3673388607139,7.59076668565169,-4.04399793803123));
#37064=CARTESIAN_POINT('Ctrl Pts',(44.6372900743475,7.18298363715391,25.4983456154475));
#37065=CARTESIAN_POINT('Ctrl Pts',(44.6178691074574,7.15763661423686,25.0949333155389));
#37066=CARTESIAN_POINT('Ctrl Pts',(44.5909499550986,7.13250342173354,24.6903522149865));
#37067=CARTESIAN_POINT('Ctrl Pts',(44.4435968973406,7.02634360727853,22.9595720745829));
#37068=CARTESIAN_POINT('Ctrl Pts',(44.0613654920327,6.87350147707393,20.3571404287178));
#37069=CARTESIAN_POINT('Ctrl Pts',(43.0472175782345,6.66841421880391,16.6255566287883));
#37070=CARTESIAN_POINT('Ctrl Pts',(41.3837014192008,6.45075222930465,12.505726151791));
#37071=CARTESIAN_POINT('Ctrl Pts',(39.1622763252268,6.25122984378583,8.71914937469031));
#37072=CARTESIAN_POINT('Ctrl Pts',(36.4470480163677,6.05595707526583,5.32735253621606));
#37073=CARTESIAN_POINT('Ctrl Pts',(33.3711340094357,5.8568061689083,2.28405026921364));
#37074=CARTESIAN_POINT('Ctrl Pts',(29.8873919147407,5.64398234710963,-0.282886838428735));
#37075=CARTESIAN_POINT('Ctrl Pts',(26.0605646588228,5.40587468584602,-2.31265259581178));
#37076=CARTESIAN_POINT('Ctrl Pts',(22.5748071053324,5.18017895256177,-3.6564426503721));
#37077=CARTESIAN_POINT('Ctrl Pts',(20.1336349934671,5.01301666232781,-4.26989781319475));
#37078=CARTESIAN_POINT('Ctrl Pts',(18.4956094199414,4.89707445701614,-4.57453714520048));
#37079=CARTESIAN_POINT('Ctrl Pts',(18.1021997947913,4.86894780999335,-4.63975778560386));
#37080=CARTESIAN_POINT('Ctrl Pts',(17.7086109162641,4.84055053954568,-4.69718161228497));
#37081=CARTESIAN_POINT('Ctrl Pts',(46.6002512122511,3.57357815210241,23.0851472908221));
#37082=CARTESIAN_POINT('Ctrl Pts',(46.5604134978277,3.55599962931061,22.6848298673109));
#37083=CARTESIAN_POINT('Ctrl Pts',(46.5129192765137,3.53868515668548,22.2837522544351));
#37084=CARTESIAN_POINT('Ctrl Pts',(46.2771234824041,3.46609807861293,20.5697250603014));
#37085=CARTESIAN_POINT('Ctrl Pts',(45.7597972462748,3.36435917107101,18.0013127653728));
#37086=CARTESIAN_POINT('Ctrl Pts',(44.5460060590501,3.23426720235262,14.3456829986935));
#37087=CARTESIAN_POINT('Ctrl Pts',(42.6554075408894,3.10147907156715,10.3433104165254));
#37088=CARTESIAN_POINT('Ctrl Pts',(40.2171323555533,2.98285053627008,6.70992527865091));
#37089=CARTESIAN_POINT('Ctrl Pts',(37.29972468766,2.86388130857434,3.50650323924174));
#37090=CARTESIAN_POINT('Ctrl Pts',(34.0357422770818,2.73730530568202,0.679396844997027));
#37091=CARTESIAN_POINT('Ctrl Pts',(30.384537644396,2.59247375589619,-1.63698871367901));
#37092=CARTESIAN_POINT('Ctrl Pts',(26.4152859351303,2.41842603756845,-3.38251562380317));
#37093=CARTESIAN_POINT('Ctrl Pts',(22.8266296158437,2.24547053120763,-4.45988818251451));
#37094=CARTESIAN_POINT('Ctrl Pts',(20.3309757484496,2.11246131963295,-4.88075398812767));
#37095=CARTESIAN_POINT('Ctrl Pts',(18.6621864827798,2.01884144332686,-5.05384262057585));
#37096=CARTESIAN_POINT('Ctrl Pts',(18.2622021015115,1.99605339732081,-5.08725599825241));
#37097=CARTESIAN_POINT('Ctrl Pts',(17.8628413159654,1.9729679754383,-5.11265663696635));
#37098=CARTESIAN_POINT('Ctrl Pts',(48.1177386369166,0.237308438758995,21.2223754846663));
#37099=CARTESIAN_POINT('Ctrl Pts',(48.0607951996036,0.227921876287717,20.8242811153145));
#37100=CARTESIAN_POINT('Ctrl Pts',(47.9960602567766,0.218854274805993,20.4257840939615));
#37101=CARTESIAN_POINT('Ctrl Pts',(47.6861498686287,0.181679983795775,18.724346543423));
#37102=CARTESIAN_POINT('Ctrl Pts',(47.0555604149621,0.133848323063104,16.1824364307684));
#37103=CARTESIAN_POINT('Ctrl Pts',(45.6742498357681,0.0830496793456984,
12.5880909151258));
#37104=CARTESIAN_POINT('Ctrl Pts',(43.5929738746605,0.0403924264632703,
8.68214080760531));
#37105=CARTESIAN_POINT('Ctrl Pts',(40.9724801352348,0.00837005963384143,
5.17606176509414));
#37106=CARTESIAN_POINT('Ctrl Pts',(37.8851037245238,-0.0279539839125438,
2.13035959848029));
#37107=CARTESIAN_POINT('Ctrl Pts',(34.4629830745002,-0.0750512999789021,
-0.51497625431155));
#37108=CARTESIAN_POINT('Ctrl Pts',(30.6709672266821,-0.14423024726241,-2.61989139939369));
#37109=CARTESIAN_POINT('Ctrl Pts',(26.5820286964953,-0.245792879606331,
-4.12482945449056));
#37110=CARTESIAN_POINT('Ctrl Pts',(22.9069936436346,-0.358291148292244,
-4.97629232812478));
#37111=CARTESIAN_POINT('Ctrl Pts',(20.3657037027299,-0.451704594358635,
-5.23361066140274));
#37112=CARTESIAN_POINT('Ctrl Pts',(18.6711961566749,-0.519340602547392,
-5.29491549463405));
#37113=CARTESIAN_POINT('Ctrl Pts',(18.26576526766,-0.535923052101836,-5.30134231507661));
#37114=CARTESIAN_POINT('Ctrl Pts',(17.8616764537007,-0.552841667182328,
-5.29961424607418));
#37115=CARTESIAN_POINT('Ctrl Pts',(49.0111526470788,-2.14030259993981,20.1280824173318));
#37116=CARTESIAN_POINT('Ctrl Pts',(48.9431158357957,-2.14321532053782,19.7311392813689));
#37117=CARTESIAN_POINT('Ctrl Pts',(48.8671976767669,-2.14576465810466,19.3340301364558));
#37118=CARTESIAN_POINT('Ctrl Pts',(48.5092053965927,-2.15494826818845,17.6395593959033));
#37119=CARTESIAN_POINT('Ctrl Pts',(47.8050951102084,-2.16016260296573,15.1131718254244));
#37120=CARTESIAN_POINT('Ctrl Pts',(46.3149438817565,-2.1481556077715,11.556583273664));
#37121=CARTESIAN_POINT('Ctrl Pts',(44.1096887388597,-2.11918777525101,7.71144046011049));
#37122=CARTESIAN_POINT('Ctrl Pts',(41.370632841532,-2.08197924289826,4.28693588598887));
#37123=CARTESIAN_POINT('Ctrl Pts',(38.1726332889339,-2.05170003121316,1.34326068419944));
#37124=CARTESIAN_POINT('Ctrl Pts',(34.6475936509573,-2.03426137368081,-1.18387570229488));
#37125=CARTESIAN_POINT('Ctrl Pts',(30.7639815309873,-2.04135770257883,-3.15062216354145));
#37126=CARTESIAN_POINT('Ctrl Pts',(26.5973047018925,-2.08278583441843,-4.49781925489811));
#37127=CARTESIAN_POINT('Ctrl Pts',(22.8662926524275,-2.14471303148954,-5.20084440966807));
#37128=CARTESIAN_POINT('Ctrl Pts',(20.2955537880838,-2.20477046252904,-5.35051189893769));
#37129=CARTESIAN_POINT('Ctrl Pts',(18.5845115980973,-2.25046208753918,-5.33818290167311));
#37130=CARTESIAN_POINT('Ctrl Pts',(18.1756045924178,-2.26180965939547,-5.3268552459772));
#37131=CARTESIAN_POINT('Ctrl Pts',(17.7685257087919,-2.27353152926925,-5.30730083266003));
#37132=CARTESIAN_POINT('Ctrl Pts',(49.5850624656363,-3.83428286431684,19.4261939233155));
#37133=CARTESIAN_POINT('Ctrl Pts',(49.5094794801401,-3.83237339034492,19.0299116731508));
#37134=CARTESIAN_POINT('Ctrl Pts',(49.4259532096492,-3.83006698099443,18.6336267626953));
#37135=CARTESIAN_POINT('Ctrl Pts',(49.0352476004593,-3.81839846831683,16.9433938910075));
#37136=CARTESIAN_POINT('Ctrl Pts',(48.2811000721071,-3.79185933798401,14.4268660936007));
#37137=CARTESIAN_POINT('Ctrl Pts',(46.7168351773588,-3.73301479320489,10.8951171019885));
#37138=CARTESIAN_POINT('Ctrl Pts',(44.4271250001086,-3.65055513724086,7.09059062588532));
#37139=CARTESIAN_POINT('Ctrl Pts',(41.6072775704128,-3.56151400652134,3.72112407924795));
#37140=CARTESIAN_POINT('Ctrl Pts',(38.3338930647704,-3.48120332570528,0.846689546782518));
#37141=CARTESIAN_POINT('Ctrl Pts',(34.7387295945766,-3.41513875248544,-1.59997654848575));
#37142=CARTESIAN_POINT('Ctrl Pts',(30.7927411759451,-3.37526128513496,-3.47238823132519));
#37143=CARTESIAN_POINT('Ctrl Pts',(26.5731913388433,-3.37099617994084,-4.71166498849067));
#37144=CARTESIAN_POINT('Ctrl Pts',(22.8041754625968,-3.39437469848804,-5.31300502085438));
#37145=CARTESIAN_POINT('Ctrl Pts',(20.2135086951711,-3.42893690611626,-5.38885186457644));
#37146=CARTESIAN_POINT('Ctrl Pts',(18.4913093104333,-3.45783930783476,-5.32600713004844));
#37147=CARTESIAN_POINT('Ctrl Pts',(18.0800672982954,-3.46518513130081,-5.30251003400118));
#37148=CARTESIAN_POINT('Ctrl Pts',(17.6709912904296,-3.47293757911652,-5.27074753251649));
#37149=CARTESIAN_POINT('Ctrl Pts',(49.7385656365263,-4.30636894546118,19.2385804425128));
#37150=CARTESIAN_POINT('Ctrl Pts',(49.6609212476581,-4.3031084050989,18.8424609291718));
#37151=CARTESIAN_POINT('Ctrl Pts',(49.5753160757238,-4.29944065268701,18.4463835567366));
#37152=CARTESIAN_POINT('Ctrl Pts',(49.1756692040682,-4.28192251284736,16.7572339716752));
#37153=CARTESIAN_POINT('Ctrl Pts',(48.4078353322892,-4.24645759656194,14.2433025862439));
#37154=CARTESIAN_POINT('Ctrl Pts',(46.8232750809732,-4.17439213330946,10.7182450608962));
#37155=CARTESIAN_POINT('Ctrl Pts',(44.5104172755431,-4.07676875425951,6.92476319565399));
#37156=CARTESIAN_POINT('Ctrl Pts',(41.6684115908783,-3.97294922980807,3.57035153883128));
#37157=CARTESIAN_POINT('Ctrl Pts',(38.3743494619475,-3.87828739688684,0.714912437194819));
#37158=CARTESIAN_POINT('Ctrl Pts',(34.7599610153453,-3.79820251809058,-1.70965444329932));
#37159=CARTESIAN_POINT('Ctrl Pts',(30.7968900398997,-3.74469501429227,-3.55614991710789));
#37160=CARTESIAN_POINT('Ctrl Pts',(26.5628886623099,-3.72710099262819,-4.76579596134831));
#37161=CARTESIAN_POINT('Ctrl Pts',(22.7835127443776,-3.7392015362719,-5.33925141242045));
#37162=CARTESIAN_POINT('Ctrl Pts',(20.1874313455853,-3.76629674044718,-5.39487746385998));
#37163=CARTESIAN_POINT('Ctrl Pts',(18.4622079723539,-3.79028538091932,-5.31820612127411));
#37164=CARTESIAN_POINT('Ctrl Pts',(18.0503342711803,-3.79646095010219,-5.29138066967352));
#37165=CARTESIAN_POINT('Ctrl Pts',(17.6407192216084,-3.80305340259771,-5.25628164552003));
#37166=CARTESIAN_POINT('Ctrl Pts',(49.8867262771747,-4.78145508078572,19.0576143929379));
#37167=CARTESIAN_POINT('Ctrl Pts',(49.8070488184353,-4.77682808742727,18.6616387837467));
#37168=CARTESIAN_POINT('Ctrl Pts',(49.7193926455521,-4.7717826224726,18.2657493044296));
#37169=CARTESIAN_POINT('Ctrl Pts',(49.3109216037794,-4.74834091216943,16.5775956967118));
#37170=CARTESIAN_POINT('Ctrl Pts',(48.5295704247379,-4.70381966688121,14.0661310574747));
#37171=CARTESIAN_POINT('Ctrl Pts',(46.9249416035674,-4.61828583278682,10.5475836926096));
#37172=CARTESIAN_POINT('Ctrl Pts',(44.5891740940081,-4.50515190400754,6.76494960996389));
#37173=CARTESIAN_POINT('Ctrl Pts',(41.7252227642596,-4.38613315046716,3.42541182621241));
#37174=CARTESIAN_POINT('Ctrl Pts',(38.4106787509553,-4.27662792828432,0.58879394549261));
#37175=CARTESIAN_POINT('Ctrl Pts',(34.7772564846155,-4.18197237106197,-1.81385442996729));
#37176=CARTESIAN_POINT('Ctrl Pts',(30.7972906070539,-4.11421750462538,-3.63463742552607));
#37177=CARTESIAN_POINT('Ctrl Pts',(26.5490240788154,-4.08262421860679,-4.81490468456639));
#37178=CARTESIAN_POINT('Ctrl Pts',(22.759448415022,-4.0828488851085,-5.36074766386016));
#37179=CARTESIAN_POINT('Ctrl Pts',(20.1580533176614,-4.10207414795096,-5.39637337123085));
#37180=CARTESIAN_POINT('Ctrl Pts',(18.429869561442,-4.12088738197538,-5.30603685065097));
#37181=CARTESIAN_POINT('Ctrl Pts',(18.0173781005166,-4.12583098108427,-5.27592339496274));
#37182=CARTESIAN_POINT('Ctrl Pts',(17.607236583243,-4.13120272145022,-5.23752968435663));
#37183=CARTESIAN_POINT('',(28.5514340253946,20.7105311502984,37.17636308254));
#37184=CARTESIAN_POINT('Ctrl Pts',(28.5514340253946,20.7105311502984,37.17636308254));
#37185=CARTESIAN_POINT('Ctrl Pts',(28.6887070741992,20.5483438544848,31.9945680076874));
#37186=CARTESIAN_POINT('Ctrl Pts',(27.8005885200067,20.4520245495079,26.7953695353565));
#37187=CARTESIAN_POINT('Ctrl Pts',(24.2300859427647,20.3052748660675,17.0649705156928));
#37188=CARTESIAN_POINT('Ctrl Pts',(21.5497888275062,20.248474007324,12.5314470346895));
#37189=CARTESIAN_POINT('Ctrl Pts',(18.0980606826517,20.1925493450898,8.66958605760119));
#37190=CARTESIAN_POINT('',(45.834019355174,-3.27137091447504,9.82390285882801));
#37191=CARTESIAN_POINT('Ctrl Pts',(28.5514340253913,20.7105311502992,37.1763630825353));
#37192=CARTESIAN_POINT('Ctrl Pts',(31.0601642882562,19.9641940681954,35.2496594015446));
#37193=CARTESIAN_POINT('Ctrl Pts',(33.2932193363368,18.7336189223949,33.1249281443677));
#37194=CARTESIAN_POINT('Ctrl Pts',(37.3699780270222,15.6437709263415,28.4860565308901));
#37195=CARTESIAN_POINT('Ctrl Pts',(39.2033043779382,13.6706054953475,25.8687734374218));
#37196=CARTESIAN_POINT('Ctrl Pts',(42.1018618790161,9.45712578015146,20.8061375995457));
#37197=CARTESIAN_POINT('Ctrl Pts',(43.224541292629,7.18268855808118,18.3050729961215));
#37198=CARTESIAN_POINT('Ctrl Pts',(44.8943670414634,2.26699026933697,13.6969285615372));
#37199=CARTESIAN_POINT('Ctrl Pts',(45.4569546562068,-0.365223992194631,
11.583121612936));
#37200=CARTESIAN_POINT('Ctrl Pts',(45.8340194423595,-3.27137053313469,9.82390224755894));
#37201=CARTESIAN_POINT('Ctrl Pts',(45.8340189392194,-3.27137100135121,9.82390309631628));
#37202=CARTESIAN_POINT('Ctrl Pts',(45.4471084733847,-3.25992112204953,9.15042791312507));
#37203=CARTESIAN_POINT('Ctrl Pts',(45.0361013987857,-3.24789096533569,8.49437671617948));
#37204=CARTESIAN_POINT('Ctrl Pts',(44.6023222643424,-3.23555894384663,7.85680669322666));
#37205=CARTESIAN_POINT('Ctrl Pts',(43.5399816289705,-3.2053573815679,6.29537487344335));
#37206=CARTESIAN_POINT('Ctrl Pts',(42.3410592562038,-3.17334534347451,4.84478916593907));
#37207=CARTESIAN_POINT('Ctrl Pts',(41.025128272205,-3.14345008158506,3.52048655147805));
#37208=CARTESIAN_POINT('Ctrl Pts',(40.1478409050367,-3.12351990598108,2.63761809705187));
#37209=CARTESIAN_POINT('Ctrl Pts',(39.2185497053661,-3.10453051989494,1.81087546743184));
#37210=CARTESIAN_POINT('Ctrl Pts',(38.2430820542904,-3.08752071373526,1.04479859058942));
#37211=CARTESIAN_POINT('Ctrl Pts',(37.2676144037253,-3.07051090758448,0.278721714147996));
#37212=CARTESIAN_POINT('Ctrl Pts',(36.245970301801,-3.0554806813514,-0.426689409586692));
#37213=CARTESIAN_POINT('Ctrl Pts',(35.183986846522,-3.04339100491455,-1.06691002414564));
#37214=CARTESIAN_POINT('Ctrl Pts',(33.5910116655829,-3.02525649028182,-2.02724094479067));
#37215=CARTESIAN_POINT('Ctrl Pts',(31.9072729398591,-3.01373821257335,-2.8408932202102));
#37216=CARTESIAN_POINT('Ctrl Pts',(30.1525134708022,-3.01128625574909,-3.49270629610018));
#37217=CARTESIAN_POINT('Ctrl Pts',(28.9826738275111,-3.00965161787009,-3.92724834567317));
#37218=CARTESIAN_POINT('Ctrl Pts',(27.7812694094895,-3.01204645592803,-4.2898618624831));
#37219=CARTESIAN_POINT('Ctrl Pts',(26.5541510246005,-3.01891855380822,-4.57608275222957));
#37220=CARTESIAN_POINT('Ctrl Pts',(25.3270327868496,-3.02579065086441,-4.86230360765662));
#37221=CARTESIAN_POINT('Ctrl Pts',(24.0742005883685,-3.03714000665748,-5.07213185436673));
#37222=CARTESIAN_POINT('Ctrl Pts',(22.8014968021072,-3.05321938564873,-5.20111578381779));
#37223=CARTESIAN_POINT('Ctrl Pts',(22.277058467955,-3.05984515577954,-5.25426571377315));
#37224=CARTESIAN_POINT('Ctrl Pts',(21.7492459773433,-3.06727406915266,-5.29368838411695));
#37225=CARTESIAN_POINT('Ctrl Pts',(21.2184673472733,-3.07550335254719,-5.31907358707771));
#37226=CARTESIAN_POINT('Ctrl Pts',(49.988903440698,-4.68328060676847,18.9373181639873));
#37227=CARTESIAN_POINT('Ctrl Pts',(49.9084825111689,-4.67927906663786,18.5401457639636));
#37228=CARTESIAN_POINT('Ctrl Pts',(49.8200206604983,-4.67486342687383,18.1430770906299));
#37229=CARTESIAN_POINT('Ctrl Pts',(49.4090563410411,-4.65418501649615,16.4549589916609));
#37230=CARTESIAN_POINT('Ctrl Pts',(48.6244718746128,-4.61395560865182,13.9459576997312));
#37231=CARTESIAN_POINT('Ctrl Pts',(47.0150672697257,-4.53496565777432,10.4313206499587));
#37232=CARTESIAN_POINT('Ctrl Pts',(44.6738386245635,-4.42959393838223,6.65349671488799));
#37233=CARTESIAN_POINT('Ctrl Pts',(41.8045972279016,-4.31850354734918,3.31907618662271));
#37234=CARTESIAN_POINT('Ctrl Pts',(38.4849815346274,-4.2170896233612,0.487882275093385));
#37235=CARTESIAN_POINT('Ctrl Pts',(34.8466814723617,-4.13063759391767,-1.90908600717672));
#37236=CARTESIAN_POINT('Ctrl Pts',(30.8621174859164,-4.07121155600733,-3.72386951312436));
#37237=CARTESIAN_POINT('Ctrl Pts',(26.6095816084296,-4.04803120464602,-4.89781636015318));
#37238=CARTESIAN_POINT('Ctrl Pts',(22.816595861502,-4.055480889925,-5.43802215119413));
#37239=CARTESIAN_POINT('Ctrl Pts',(20.2131109731287,-4.07952578289679,-5.46975503770605));
#37240=CARTESIAN_POINT('Ctrl Pts',(18.4813977696839,-4.10152925776619,-5.37669708188378));
#37241=CARTESIAN_POINT('Ctrl Pts',(18.0664172651078,-4.1072571624472,-5.34575229868548));
#37242=CARTESIAN_POINT('Ctrl Pts',(17.6538343163326,-4.11341014061892,-5.3064425898067));
#37243=CARTESIAN_POINT('Ctrl Pts',(49.8052654310235,-4.24009445412503,19.1620102019682));
#37244=CARTESIAN_POINT('Ctrl Pts',(49.7270640779776,-4.23725223817857,18.7645791085326));
#37245=CARTESIAN_POINT('Ctrl Pts',(49.6408401586447,-4.23400446880359,18.3672011094939));
#37246=CARTESIAN_POINT('Ctrl Pts',(49.2394704796158,-4.21832863439708,16.6775446746884));
#37247=CARTESIAN_POINT('Ctrl Pts',(48.469563803724,-4.18572164472913,14.1652201577743));
#37248=CARTESIAN_POINT('Ctrl Pts',(46.8819417217329,-4.11799618192084,10.6427061382864));
#37249=CARTESIAN_POINT('Ctrl Pts',(44.5655843103686,-4.02550335874969,6.85234360018412));
#37250=CARTESIAN_POINT('Ctrl Pts',(41.720191767349,-3.92690475481451,3.50123729401103));
#37251=CARTESIAN_POINT('Ctrl Pts',(38.4228868628256,-3.83755718932749,0.649285878422626));
#37252=CARTESIAN_POINT('Ctrl Pts',(34.8053848532926,-3.76285616468038,-1.771645267414));
#37253=CARTESIAN_POINT('Ctrl Pts',(30.8393834269129,-3.71481495977278,-3.61432174429343));
#37254=CARTESIAN_POINT('Ctrl Pts',(26.6026633134566,-3.70275434803773,-4.81996639174259));
#37255=CARTESIAN_POINT('Ctrl Pts',(22.8211151345275,-3.71962751323487,-5.38986722901264));
#37256=CARTESIAN_POINT('Ctrl Pts',(20.2236998257982,-3.74992063397164,-5.44304425293645));
#37257=CARTESIAN_POINT('Ctrl Pts',(18.4954234201959,-3.77604797989279,-5.36463613821515));
#37258=CARTESIAN_POINT('Ctrl Pts',(18.0811694161186,-3.78276245762616,-5.33722888584272));
#37259=CARTESIAN_POINT('Ctrl Pts',(17.6692128822404,-3.78989370687861,-5.30146219782923));
#37260=CARTESIAN_POINT('Ctrl Pts',(49.6179682497192,-3.80075287541765,19.3912747502332));
#37261=CARTESIAN_POINT('Ctrl Pts',(49.5420021295319,-3.79905339336963,18.9935700937101));
#37262=CARTESIAN_POINT('Ctrl Pts',(49.4580313687019,-3.79695621683146,18.5958674888762));
#37263=CARTESIAN_POINT('Ctrl Pts',(49.0663192419952,-3.78620663871065,16.9046059783843));
#37264=CARTESIAN_POINT('Ctrl Pts',(48.3111769729803,-3.76109400159902,14.3888636064159));
#37265=CARTESIAN_POINT('Ctrl Pts',(46.7454425808103,-3.70440674399875,10.8583542991997));
#37266=CARTESIAN_POINT('Ctrl Pts',(44.4540536385309,-3.62448835210827,7.05534342793885));
#37267=CARTESIAN_POINT('Ctrl Pts',(41.632583178043,-3.53802316526296,3.6874762390026));
#37268=CARTESIAN_POINT('Ctrl Pts',(38.3576469800422,-3.46032715355504,0.814721189671188));
#37269=CARTESIAN_POINT('Ctrl Pts',(34.7609965086106,-3.39690914788247,-1.63020282853092));
#37270=CARTESIAN_POINT('Ctrl Pts',(30.8136110902934,-3.35971861494906,-3.50079583530382));
#37271=CARTESIAN_POINT('Ctrl Pts',(26.5927665124587,-3.35817927654809,-4.73817887084428));
#37272=CARTESIAN_POINT('Ctrl Pts',(22.8227159303205,-3.38391914529348,-5.33784454604279));
#37273=CARTESIAN_POINT('Ctrl Pts',(20.2314124468981,-3.42007079724739,-5.41254106449418));
#37274=CARTESIAN_POINT('Ctrl Pts',(18.5066013369709,-3.45006162272336,-5.34884664801723));
#37275=CARTESIAN_POINT('Ctrl Pts',(18.0930800003721,-3.45770043113048,-5.32499411449625));
#37276=CARTESIAN_POINT('Ctrl Pts',(17.6817553325294,-3.46574819271174,-5.29278929448323));
#37277=CARTESIAN_POINT('Ctrl Pts',(48.944645465743,-2.2653457359543,20.2158180144603));
#37278=CARTESIAN_POINT('Ctrl Pts',(48.876613446234,-2.26761569662348,19.8170914326486));
#37279=CARTESIAN_POINT('Ctrl Pts',(48.8006389988634,-2.26951335386862,19.4181870566248));
#37280=CARTESIAN_POINT('Ctrl Pts',(48.4431952693583,-2.27586002752392,17.7210231775921));
#37281=CARTESIAN_POINT('Ctrl Pts',(47.7404087354438,-2.27671432942662,15.1928853145256));
#37282=CARTESIAN_POINT('Ctrl Pts',(46.2522083988626,-2.25814179129592,11.6337547981385));
#37283=CARTESIAN_POINT('Ctrl Pts',(44.0491870356822,-2.2214798205824,7.78574796375675));
#37284=CARTESIAN_POINT('Ctrl Pts',(41.3123112021794,-2.17652897108851,4.35851069495035));
#37285=CARTESIAN_POINT('Ctrl Pts',(38.1164400187034,-2.13845241575724,1.41223808195806));
#37286=CARTESIAN_POINT('Ctrl Pts',(34.5934903935758,-2.11316923258448,-1.11738683308532));
#37287=CARTESIAN_POINT('Ctrl Pts',(30.7119251016983,-2.11235831802136,-3.086485669945));
#37288=CARTESIAN_POINT('Ctrl Pts',(26.5472626963964,-2.14581153060268,-4.4359016919901));
#37289=CARTESIAN_POINT('Ctrl Pts',(22.8179615735058,-2.20085463389179,-5.14073972565149));
#37290=CARTESIAN_POINT('Ctrl Pts',(20.2483577846406,-2.25628908058851,-5.29155852335286));
#37291=CARTESIAN_POINT('Ctrl Pts',(18.5358669958649,-2.29898278275007,-5.27995411268357));
#37292=CARTESIAN_POINT('Ctrl Pts',(18.1249528052827,-2.30966173471912,-5.26869642388997));
#37293=CARTESIAN_POINT('Ctrl Pts',(17.7158788419632,-2.32072459453129,-5.24912151426549));
#37294=CARTESIAN_POINT('Ctrl Pts',(47.6809434698657,0.42091842584111,21.764906316134));
#37295=CARTESIAN_POINT('Ctrl Pts',(47.6272638993357,0.412015546281074,21.3641829634742));
#37296=CARTESIAN_POINT('Ctrl Pts',(47.565755337614,0.403442573942463,20.9629650061253));
#37297=CARTESIAN_POINT('Ctrl Pts',(47.2703119003642,0.368526239150617,19.2545662589912));
#37298=CARTESIAN_POINT('Ctrl Pts',(46.6622260261044,0.324281374370589,16.7032339039416));
#37299=CARTESIAN_POINT('Ctrl Pts',(45.3142072503292,0.279215865745994,13.0914162878439));
#37300=CARTESIAN_POINT('Ctrl Pts',(43.2708954640494,0.243759038204317,9.1612330567983));
#37301=CARTESIAN_POINT('Ctrl Pts',(40.6868518840738,0.21967725703067,5.62616928052599));
#37302=CARTESIAN_POINT('Ctrl Pts',(37.633788218554,0.192114722189047,2.54682342316403));
#37303=CARTESIAN_POINT('Ctrl Pts',(34.243942068342,0.154437491851918,-0.135833115208792));
#37304=CARTESIAN_POINT('Ctrl Pts',(30.4812454080981,0.0954817696064694,
-2.28260255543497));
#37305=CARTESIAN_POINT('Ctrl Pts',(26.4180719635485,0.0048363712043943,
-3.83383662526902));
#37306=CARTESIAN_POINT('Ctrl Pts',(22.7624168656732,-0.0979118428630517,
-4.72798729865453));
#37307=CARTESIAN_POINT('Ctrl Pts',(20.2320685893873,-0.184631554593919,
-5.01574202177787));
#37308=CARTESIAN_POINT('Ctrl Pts',(18.5418851689888,-0.247909792323189,
-5.09781715603392));
#37309=CARTESIAN_POINT('Ctrl Pts',(18.1357069004105,-0.263520166061751,
-5.10923666301494));
#37310=CARTESIAN_POINT('Ctrl Pts',(17.7307374709918,-0.279478515480188,
-5.11242798885562));
#37311=CARTESIAN_POINT('Ctrl Pts',(45.7213662087155,3.93922736422659,24.1716806442701));
#37312=CARTESIAN_POINT('Ctrl Pts',(45.688208426122,3.92273017306588,23.7676952109987));
#37313=CARTESIAN_POINT('Ctrl Pts',(45.6473827402039,3.90651491483579,23.3627796511822));
#37314=CARTESIAN_POINT('Ctrl Pts',(45.4405866009357,3.83888692720806,21.6367355343485));
#37315=CARTESIAN_POINT('Ctrl Pts',(44.9678249093539,3.74496038387833,19.0500710475274));
#37316=CARTESIAN_POINT('Ctrl Pts',(43.8199173057419,3.6271896762232,15.3604237886896));
#37317=CARTESIAN_POINT('Ctrl Pts',(42.0043881080348,3.50969140214063,11.3107097806898));
#37318=CARTESIAN_POINT('Ctrl Pts',(39.6381007942075,3.40771510315772,7.62053324398369));
#37319=CARTESIAN_POINT('Ctrl Pts',(36.7883508830545,3.30695483103527,4.35105340659633));
#37320=CARTESIAN_POINT('Ctrl Pts',(33.5879037474396,3.1998573133211,1.45057582162554));
#37321=CARTESIAN_POINT('Ctrl Pts',(29.9942635963678,3.07607789704229,-0.948197922906822));
#37322=CARTESIAN_POINT('Ctrl Pts',(26.075402425309,2.92448144596071,-2.7849461353621));
#37323=CARTESIAN_POINT('Ctrl Pts',(22.5244809527974,2.77158317941627,-3.9464844359537));
#37324=CARTESIAN_POINT('Ctrl Pts',(20.049992630345,2.65236568914073,-4.42739273892755));
#37325=CARTESIAN_POINT('Ctrl Pts',(18.3915748274528,2.56779645721963,-4.6415318716897));
#37326=CARTESIAN_POINT('Ctrl Pts',(17.9921830064857,2.54707902977605,-4.68497343012829));
#37327=CARTESIAN_POINT('Ctrl Pts',(17.5931404618472,2.52604544176493,-4.72036483483639));
#37328=CARTESIAN_POINT('Ctrl Pts',(43.2820442732254,7.64857049485316,27.1714239460178));
#37329=CARTESIAN_POINT('Ctrl Pts',(43.2727023403867,7.62538079009264,26.7633085649188));
#37330=CARTESIAN_POINT('Ctrl Pts',(43.2558781734963,7.6024320797305,26.353789632655));
#37331=CARTESIAN_POINT('Ctrl Pts',(43.1519567273492,7.50598047950645,24.6060794051385));
#37332=CARTESIAN_POINT('Ctrl Pts',(42.8361624278849,7.36825978906471,21.9768147066715));
#37333=CARTESIAN_POINT('Ctrl Pts',(41.9201606521025,7.18657585481396,18.195120286621));
#37334=CARTESIAN_POINT('Ctrl Pts',(40.3683770686699,6.99739878870591,14.0054622248624));
#37335=CARTESIAN_POINT('Ctrl Pts',(38.2539595021366,6.82819742189185,10.1350305421312));
#37336=CARTESIAN_POINT('Ctrl Pts',(35.6391340409848,6.66543158101024,6.64562945258854));
#37337=CARTESIAN_POINT('Ctrl Pts',(32.6573475458408,6.50060855796851,3.49387433273689));
#37338=CARTESIAN_POINT('Ctrl Pts',(29.2586568556057,6.32441606849526,0.805112441394477));
#37339=CARTESIAN_POINT('Ctrl Pts',(25.5059908438053,6.12505774886043,-1.35957124492499));
#37340=CARTESIAN_POINT('Ctrl Pts',(22.075521138649,5.93384517916791,-2.82786038740783));
#37341=CARTESIAN_POINT('Ctrl Pts',(19.6651555950876,5.79035915091665,-3.53013920906786));
#37342=CARTESIAN_POINT('Ctrl Pts',(18.0431548018333,5.69001969995687,-3.89557055616166));
#37343=CARTESIAN_POINT('Ctrl Pts',(17.6516126072861,5.66551509710643,-3.97576378962003));
#37344=CARTESIAN_POINT('Ctrl Pts',(17.2594995078076,5.64071489355821,-4.04817830458482));
#37345=CARTESIAN_POINT('Ctrl Pts',(40.985186418,10.6050661536892,29.9982594338762));
#37346=CARTESIAN_POINT('Ctrl Pts',(40.9969328308233,10.5777689837161,29.5862652996575));
#37347=CARTESIAN_POINT('Ctrl Pts',(41.0013571377618,10.5506896266998,29.1724780443182));
#37348=CARTESIAN_POINT('Ctrl Pts',(40.9884998486727,10.4365567481294,27.404896453078));
#37349=CARTESIAN_POINT('Ctrl Pts',(40.8115942540796,10.2719415070743,24.7370183562784));
#37350=CARTESIAN_POINT('Ctrl Pts',(40.1006192580091,10.0511774947007,20.8729636138941));
#37351=CARTESIAN_POINT('Ctrl Pts',(38.7818181838249,9.81863871620139,16.5589607680871));
#37352=CARTESIAN_POINT('Ctrl Pts',(36.8896525789635,9.60967367489776,12.5292063966697));
#37353=CARTESIAN_POINT('Ctrl Pts',(34.4818871352799,9.41153176383594,8.84607749903719));
#37354=CARTESIAN_POINT('Ctrl Pts',(31.6926260287593,9.21500541081661,5.47340241149087));
#37355=CARTESIAN_POINT('Ctrl Pts',(28.4653194124203,9.01175979868378,2.53015669942969));
#37356=CARTESIAN_POINT('Ctrl Pts',(24.8584646940975,8.78956564702969,0.0780936876946292));
#37357=CARTESIAN_POINT('Ctrl Pts',(21.5334346929017,8.58124477590158,-1.6587653846784));
#37358=CARTESIAN_POINT('Ctrl Pts',(19.1790085003012,8.42762540105217,-2.55471275350617));
#37359=CARTESIAN_POINT('Ctrl Pts',(17.5886957847182,8.32086564673385,-3.05245934568359));
#37360=CARTESIAN_POINT('Ctrl Pts',(17.2040547252269,8.29482075310626,-3.16483640809568));
#37361=CARTESIAN_POINT('Ctrl Pts',(16.8181095137966,8.26849188852043,-3.26971525901482));
#37362=CARTESIAN_POINT('Ctrl Pts',(38.1960047398292,13.6252616883324,33.4321039804979));
#37363=CARTESIAN_POINT('Ctrl Pts',(38.2320179600167,13.5952855444977,33.0155280106869));
#37364=CARTESIAN_POINT('Ctrl Pts',(38.2608843008179,13.5655149131873,32.596745525132));
#37365=CARTESIAN_POINT('Ctrl Pts',(38.3527474093692,13.4398628522405,30.8060971867503));
#37366=CARTESIAN_POINT('Ctrl Pts',(38.3355056499632,13.2576618204372,28.0936014929509));
#37367=CARTESIAN_POINT('Ctrl Pts',(37.860056066436,13.0115743729063,24.1348762335303));
#37368=CARTESIAN_POINT('Ctrl Pts',(36.8086829471625,12.751644575675,19.6783627939692));
#37369=CARTESIAN_POINT('Ctrl Pts',(35.171342701358,12.5189796899122,15.4664292044507));
#37370=CARTESIAN_POINT('Ctrl Pts',(33.0006620268248,12.301865256328,11.5621247517028));
#37371=CARTESIAN_POINT('Ctrl Pts',(30.4315525548981,12.0904144587841,7.93746377529417));
#37372=CARTESIAN_POINT('Ctrl Pts',(27.3998095635454,11.8774764455751,4.70421501534603));
#37373=CARTESIAN_POINT('Ctrl Pts',(23.9588320023988,11.6504923923572,1.92490607313789));
#37374=CARTESIAN_POINT('Ctrl Pts',(20.7533189738236,11.4410171343385,-0.117626788490311));
#37375=CARTESIAN_POINT('Ctrl Pts',(18.461936909906,11.2882220371981,-1.23390159894501));
#37376=CARTESIAN_POINT('Ctrl Pts',(16.907176814582,11.1823584691134,-1.88214643141196));
#37377=CARTESIAN_POINT('Ctrl Pts',(16.5303633666016,11.1565388193505,-2.03115178324461));
#37378=CARTESIAN_POINT('Ctrl Pts',(16.1515047029193,11.1304479812224,-2.17300196454322));
#37379=CARTESIAN_POINT('Ctrl Pts',(35.6250369117929,15.9398275064074,36.5973462848406));
#37380=CARTESIAN_POINT('Ctrl Pts',(35.6823628409769,15.9092719019138,36.176722702768));
#37381=CARTESIAN_POINT('Ctrl Pts',(35.7326842526493,15.8789225535602,35.7535587401085));
#37382=CARTESIAN_POINT('Ctrl Pts',(35.9164273802557,15.7507918597713,33.9428065182253));
#37383=CARTESIAN_POINT('Ctrl Pts',(36.0392336977157,15.5646999212503,31.191436002328));
#37384=CARTESIAN_POINT('Ctrl Pts',(35.7702402889224,15.3133344724918,27.15026887435));
#37385=CARTESIAN_POINT('Ctrl Pts',(34.9531102563103,15.0487502016962,22.5697046993983));
#37386=CARTESIAN_POINT('Ctrl Pts',(33.5387202772831,14.8142492774957,18.1992580018583));
#37387=CARTESIAN_POINT('Ctrl Pts',(31.5751615684769,14.5991383033468,14.1025862551498));
#37388=CARTESIAN_POINT('Ctrl Pts',(29.1980931926873,14.3930646018661,10.2588220611129));
#37389=CARTESIAN_POINT('Ctrl Pts',(26.3365213630746,14.1899609567462,6.77349474422793));
#37390=CARTESIAN_POINT('Ctrl Pts',(23.0393473535078,13.977122935371,3.70982406676064));
#37391=CARTESIAN_POINT('Ctrl Pts',(19.9369788908936,13.7824369346935,1.40173743650218));
#37392=CARTESIAN_POINT('Ctrl Pts',(17.6996045937325,13.6409944051188,0.0940973017916472));
#37393=CARTESIAN_POINT('Ctrl Pts',(16.175122288904,13.5429643472183,-0.684847627751295));
#37394=CARTESIAN_POINT('Ctrl Pts',(15.8050468938553,13.5190447294408,-0.865658102920624));
#37395=CARTESIAN_POINT('Ctrl Pts',(15.4323648377265,13.4948677704672,-1.0396092374574));
#37396=CARTESIAN_POINT('Ctrl Pts',(32.5619623291767,18.188947172369,40.3670019380271));
#37397=CARTESIAN_POINT('Ctrl Pts',(32.6436186340454,18.1597316481657,39.9418646159408));
#37398=CARTESIAN_POINT('Ctrl Pts',(32.7184160259125,18.1307342364494,39.5138369066759));
#37399=CARTESIAN_POINT('Ctrl Pts',(33.0069098816923,18.0083786966032,37.6808619105327));
#37400=CARTESIAN_POINT('Ctrl Pts',(33.2893521670055,17.830846834045,34.8862535762931));
#37401=CARTESIAN_POINT('Ctrl Pts',(33.2555646360601,17.5925027676131,30.7527878233976));
#37402=CARTESIAN_POINT('Ctrl Pts',(32.7051064889568,17.3443426911773,26.0328695343581));
#37403=CARTESIAN_POINT('Ctrl Pts',(31.5442365963815,17.1289494695207,21.4839276053616));
#37404=CARTESIAN_POINT('Ctrl Pts',(29.8158089418295,16.9369213116231,17.1703445361495));
#37405=CARTESIAN_POINT('Ctrl Pts',(27.6563687494004,16.7575317657622,13.0793476612587));
#37406=CARTESIAN_POINT('Ctrl Pts',(24.9870614584278,16.5859876106103,9.30941171936927));
#37407=CARTESIAN_POINT('Ctrl Pts',(21.8515956138191,16.4095763329362,5.92457317984241));
#37408=CARTESIAN_POINT('Ctrl Pts',(18.8645313333366,16.2491906636996,3.31651020420802));
#37409=CARTESIAN_POINT('Ctrl Pts',(16.6869382415737,16.1323920433636,1.79267841142363));
#37410=CARTESIAN_POINT('Ctrl Pts',(15.1957006142707,16.0510402241362,0.866074551347136));
#37411=CARTESIAN_POINT('Ctrl Pts',(14.8330943827188,16.0311583490605,0.649363554666546));
#37412=CARTESIAN_POINT('Ctrl Pts',(14.4673343468776,16.01103806515,0.43920571884));
#37413=CARTESIAN_POINT('Ctrl Pts',(29.7866051558503,19.7983627848149,43.7804409554261));
#37414=CARTESIAN_POINT('Ctrl Pts',(29.889459148105,19.7720645135703,43.3515471357187));
#37415=CARTESIAN_POINT('Ctrl Pts',(29.9855637697716,19.7460021313493,42.9194818145262));
#37416=CARTESIAN_POINT('Ctrl Pts',(30.3651772634003,19.6361820466171,41.0681036249458));
#37417=CARTESIAN_POINT('Ctrl Pts',(30.7864638771974,19.4774394485581,38.2372822629002));
#37418=CARTESIAN_POINT('Ctrl Pts',(30.9571529902603,19.2670183310104,34.025583050656));
#37419=CARTESIAN_POINT('Ctrl Pts',(30.6383680494902,19.0520629838802,29.1868126511722));
#37420=CARTESIAN_POINT('Ctrl Pts',(29.697484286248,18.8717166252608,24.4849595349987));
#37421=CARTESIAN_POINT('Ctrl Pts',(28.1727214392882,18.7178122962125,19.9850708127111));
#37422=CARTESIAN_POINT('Ctrl Pts',(26.2014191897252,18.5794411422907,15.6814277247905));
#37423=CARTESIAN_POINT('Ctrl Pts',(23.6977578050179,18.4529446490623,11.6663983296305));
#37424=CARTESIAN_POINT('Ctrl Pts',(20.7008504579983,18.3257380682571,8.00476104675949));
#37425=CARTESIAN_POINT('Ctrl Pts',(17.8118961304768,18.2102139945187,5.13804607190731));
#37426=CARTESIAN_POINT('Ctrl Pts',(15.6845649626298,18.1249152482566,3.42774500705276));
#37427=CARTESIAN_POINT('Ctrl Pts',(14.2209995873091,18.064727637235,2.37376826844734));
#37428=CARTESIAN_POINT('Ctrl Pts',(13.8646592739966,18.0499634327475,2.12613341463877));
#37429=CARTESIAN_POINT('Ctrl Pts',(13.5047578340977,18.0349776243875,1.88482906425678));
#37430=CARTESIAN_POINT('Ctrl Pts',(27.7526639506774,20.6836496418694,46.2795822977866));
#37431=CARTESIAN_POINT('Ctrl Pts',(27.8705165233211,20.6606519170286,45.8482413413726));
#37432=CARTESIAN_POINT('Ctrl Pts',(27.9816862133389,20.6379063239872,45.4135423099364));
#37433=CARTESIAN_POINT('Ctrl Pts',(28.4256799254442,20.5422448076096,43.5501481782092));
#37434=CARTESIAN_POINT('Ctrl Pts',(28.9450621552993,20.4047755971079,40.6951986457009));
#37435=CARTESIAN_POINT('Ctrl Pts',(29.2601668709738,20.225761668211,36.430272862676));
#37436=CARTESIAN_POINT('Ctrl Pts',(29.104902952896,20.0475517349526,31.5097756876155));
#37437=CARTESIAN_POINT('Ctrl Pts',(28.3191048348243,19.9048724048602,26.7019746382763));
#37438=CARTESIAN_POINT('Ctrl Pts',(26.9376410290806,19.790507905872,22.0724169164535));
#37439=CARTESIAN_POINT('Ctrl Pts',(25.0984225618106,19.6935273080542,17.6204087054907));
#37440=CARTESIAN_POINT('Ctrl Pts',(22.7105958915495,19.6110850660289,13.4340017986264));
#37441=CARTESIAN_POINT('Ctrl Pts',(19.8099493704634,19.530779076001,9.57852885042505));
#37442=CARTESIAN_POINT('Ctrl Pts',(16.9885762929046,19.4573327991495,6.53052694702122));
#37443=CARTESIAN_POINT('Ctrl Pts',(14.8953515136484,19.4012238336331,4.68944489777427));
#37444=CARTESIAN_POINT('Ctrl Pts',(13.4503222706086,19.3605693891818,3.54611204363267));
#37445=CARTESIAN_POINT('Ctrl Pts',(13.0981976310342,19.3505226070412,3.27681676297094));
#37446=CARTESIAN_POINT('Ctrl Pts',(12.7422574691309,19.3402634731691,3.01372770483773));
#37447=CARTESIAN_POINT('Ctrl Pts',(26.6080532394981,21.117312799858,47.6853113156483));
#37448=CARTESIAN_POINT('Ctrl Pts',(26.7342384178453,21.0964267127388,47.2526690936168));
#37449=CARTESIAN_POINT('Ctrl Pts',(26.8537736232549,21.0758020890032,46.8165686819745));
#37450=CARTESIAN_POINT('Ctrl Pts',(27.3335005166717,20.9891913310095,44.9467780571391));
#37451=CARTESIAN_POINT('Ctrl Pts',(27.9073295027061,20.8653273744228,42.0788365144294));
#37452=CARTESIAN_POINT('Ctrl Pts',(28.3025817120245,20.7063681300896,37.784920215597));
#37453=CARTESIAN_POINT('Ctrl Pts',(28.2380468618629,20.5515335415639,32.8196546797573));
#37454=CARTESIAN_POINT('Ctrl Pts',(27.5382555433897,20.4326519806542,27.9535830792282));
#37455=CARTESIAN_POINT('Ctrl Pts',(26.2361957108526,20.3430531321453,23.252537996115));
#37456=CARTESIAN_POINT('Ctrl Pts',(24.4700967317106,20.2718184169426,18.7186288699449));
#37457=CARTESIAN_POINT('Ctrl Pts',(22.1462824761541,20.2165549432469,14.4375077942308));
#37458=CARTESIAN_POINT('Ctrl Pts',(19.2986750354573,20.164982094833,10.4748228833348));
#37459=CARTESIAN_POINT('Ctrl Pts',(16.5143939304978,20.117197691553,7.32650190177016));
#37460=CARTESIAN_POINT('Ctrl Pts',(14.4397578973729,20.0788282397779,5.41302288571427));
#37461=CARTESIAN_POINT('Ctrl Pts',(13.0047690687654,20.0500302875854,4.22021769274083));
#37462=CARTESIAN_POINT('Ctrl Pts',(12.6549332160082,20.0428451797642,3.93894201614119));
#37463=CARTESIAN_POINT('Ctrl Pts',(12.3011493997076,20.0354515632684,3.66381517387371));
#37464=CARTESIAN_POINT('Ctrl Pts',(26.2824873057561,21.2334813897109,48.0850725526183));
#37465=CARTESIAN_POINT('Ctrl Pts',(26.4110343322392,21.2132228077857,47.6520643827852));
#37466=CARTESIAN_POINT('Ctrl Pts',(26.5329401420435,21.1932283095702,47.2155698874215));
#37467=CARTESIAN_POINT('Ctrl Pts',(27.022790635021,21.1093059289188,45.3439807507387));
#37468=CARTESIAN_POINT('Ctrl Pts',(27.6120426416372,20.9894835119608,42.4723801622684));
#37469=CARTESIAN_POINT('Ctrl Pts',(28.0299894261123,20.8364792943525,38.1702892347921));
#37470=CARTESIAN_POINT('Ctrl Pts',(27.991132522269,20.6885792302246,33.1923965419472));
#37471=CARTESIAN_POINT('Ctrl Pts',(27.3156638017101,20.5767478260626,28.3098930006326));
#37472=CARTESIAN_POINT('Ctrl Pts',(26.0360362828936,20.4944756050622,23.5886985169737));
#37473=CARTESIAN_POINT('Ctrl Pts',(24.2905703227061,20.4308554028779,19.0317189717236));
#37474=CARTESIAN_POINT('Ctrl Pts',(21.9847846102783,20.3836340081555,14.7239348286272));
#37475=CARTESIAN_POINT('Ctrl Pts',(19.1520689743563,20.340580727313,10.7310827937134));
#37476=CARTESIAN_POINT('Ctrl Pts',(16.3781561160741,20.3004356869138,7.55454097932343));
#37477=CARTESIAN_POINT('Ctrl Pts',(14.3086760657568,20.2673681898868,5.62069087823361));
#37478=CARTESIAN_POINT('Ctrl Pts',(12.8764521475924,20.2421246596599,4.41396068576133));
#37479=CARTESIAN_POINT('Ctrl Pts',(12.5272471452757,20.2357981340653,4.12931503535631));
#37480=CARTESIAN_POINT('Ctrl Pts',(12.1740582093971,20.2292648564311,3.85080413039918));
#37481=CARTESIAN_POINT('Ctrl Pts',(25.9559446728124,21.3428689572265,48.4859646953694));
#37482=CARTESIAN_POINT('Ctrl Pts',(26.0868514733104,21.323266505305,48.0525937135402));
#37483=CARTESIAN_POINT('Ctrl Pts',(26.2111255193517,21.303930781031,47.6157083582835));
#37484=CARTESIAN_POINT('Ctrl Pts',(26.7110882848482,21.2228186866547,45.7423349337262));
#37485=CARTESIAN_POINT('Ctrl Pts',(27.3157439744971,21.1072213437662,42.8670987183852));
#37486=CARTESIAN_POINT('Ctrl Pts',(27.7563489980754,20.9604400919523,38.5568768250566));
#37487=CARTESIAN_POINT('Ctrl Pts',(27.7431168114943,20.819779963638,33.5664217702629));
#37488=CARTESIAN_POINT('Ctrl Pts',(27.0919024222535,20.7152993064879,28.6675748991354));
#37489=CARTESIAN_POINT('Ctrl Pts',(25.8346222954885,20.6406553883908,23.9263498379602));
#37490=CARTESIAN_POINT('Ctrl Pts',(24.1096882069938,20.5849601975755,19.3464505651354));
#37491=CARTESIAN_POINT('Ctrl Pts',(21.8218093008398,20.5461109852346,15.0121949824723));
#37492=CARTESIAN_POINT('Ctrl Pts',(19.0038402671502,20.5119420676311,10.9894081969158));
#37493=CARTESIAN_POINT('Ctrl Pts',(16.2401496479356,20.4797911688045,7.78487143238121));
#37494=CARTESIAN_POINT('Ctrl Pts',(14.1757138007688,20.4522911786996,5.83080964155293));
#37495=CARTESIAN_POINT('Ctrl Pts',(12.7461750731845,20.4307901345004,4.6102596399058));
#37496=CARTESIAN_POINT('Ctrl Pts',(12.3975828398805,20.4253683033402,4.3222709374315));
#37497=CARTESIAN_POINT('Ctrl Pts',(12.0449717795587,20.4197421663948,4.04040440327869));
#37498=CARTESIAN_POINT('',(28.5350439006909,20.5529756002067,37.188944948637));
#37499=CARTESIAN_POINT('Ctrl Pts',(45.8340192197807,-3.27137127985418,9.82390328601451));
#37500=CARTESIAN_POINT('Ctrl Pts',(44.9697966722668,1.76302065361956,13.855987239011));
#37501=CARTESIAN_POINT('Ctrl Pts',(43.3148043132766,6.26298702225421,18.861450934027));
#37502=CARTESIAN_POINT('Ctrl Pts',(38.8444439114925,12.5188402724798,26.3935858075399));
#37503=CARTESIAN_POINT('Ctrl Pts',(37.0863575215197,14.4577038717082,28.8308190938515));
#37504=CARTESIAN_POINT('Ctrl Pts',(33.151540262371,17.848637426394,33.2637736993417));
#37505=CARTESIAN_POINT('Ctrl Pts',(30.9674108740526,19.3555632898772,35.3225922516136));
#37506=CARTESIAN_POINT('Ctrl Pts',(28.5350439006906,20.5529756002057,37.1889449486372));
#37507=CARTESIAN_POINT('Ctrl Pts',(18.4983482597372,19.9464420456703,9.15631398661356));
#37508=CARTESIAN_POINT('Ctrl Pts',(21.8233107194045,20.0189549105364,12.9978580624312));
#37509=CARTESIAN_POINT('Ctrl Pts',(24.3992471837434,20.0954766247834,17.4724801790673));
#37510=CARTESIAN_POINT('Ctrl Pts',(27.8197485288317,20.2752040736289,27.033257475201));
#37511=CARTESIAN_POINT('Ctrl Pts',(28.6662063188346,20.3824974081049,32.1189996344999));
#37512=CARTESIAN_POINT('Ctrl Pts',(28.5350439006908,20.5529756002056,37.188944948637));
#37513=CARTESIAN_POINT('Ctrl Pts',(27.1639503240327,20.9435908393615,46.4304062506873));
#37514=CARTESIAN_POINT('Ctrl Pts',(27.2038388093363,20.9358615047579,46.2802752340366));
#37515=CARTESIAN_POINT('Ctrl Pts',(27.2437272946399,20.9281321701544,46.1301442173858));
#37516=CARTESIAN_POINT('Ctrl Pts',(27.2836157799436,20.9204028355509,45.980013200735));
#37517=CARTESIAN_POINT('Ctrl Pts',(31.2724643103077,20.1474693751975,30.9669115356589));
#37518=CARTESIAN_POINT('Ctrl Pts',(25.5907014765415,20.0812550388979,14.0171226984615));
#37519=CARTESIAN_POINT('Ctrl Pts',(13.4755336335094,19.8399463130827,4.31382061658607));
#37520=CARTESIAN_POINT('Ctrl Pts',(27.1640149500145,20.9469886892296,46.4303364767158));
#37521=CARTESIAN_POINT('Ctrl Pts',(27.203911504098,20.9392720585054,46.2802053778394));
#37522=CARTESIAN_POINT('Ctrl Pts',(27.2438080581816,20.9315554277811,46.130074278963));
#37523=CARTESIAN_POINT('Ctrl Pts',(27.2837046122652,20.9238387970569,45.9799431800866));
#37524=CARTESIAN_POINT('Ctrl Pts',(31.2733600206231,20.1521757246323,30.9668332924482));
#37525=CARTESIAN_POINT('Ctrl Pts',(25.5911393772508,20.0873688943554,14.0170271739793));
#37526=CARTESIAN_POINT('Ctrl Pts',(13.4761812282898,19.8474084919615,4.31358578508753));
#37527=CARTESIAN_POINT('Ctrl Pts',(27.1640795759962,20.9503865390978,46.4302667027442));
#37528=CARTESIAN_POINT('Ctrl Pts',(27.2039841988597,20.9426826122528,46.2801355216422));
#37529=CARTESIAN_POINT('Ctrl Pts',(27.2438888217233,20.9349786854078,46.1300043405402));
#37530=CARTESIAN_POINT('Ctrl Pts',(27.2837934445868,20.9272747585629,45.9798731594382));
#37531=CARTESIAN_POINT('Ctrl Pts',(31.2742557309385,20.1568820740671,30.9667550492374));
#37532=CARTESIAN_POINT('Ctrl Pts',(25.5915772779602,20.093482749813,14.016931649497));
#37533=CARTESIAN_POINT('Ctrl Pts',(13.4768288230703,19.8548706708402,4.31335095358899));
#37534=CARTESIAN_POINT('Ctrl Pts',(27.164144201978,20.9537843889659,46.4301969287727));
#37535=CARTESIAN_POINT('Ctrl Pts',(27.2040568936215,20.9460931660003,46.2800656654451));
#37536=CARTESIAN_POINT('Ctrl Pts',(27.2439695852649,20.9384019430346,46.1299344021174));
#37537=CARTESIAN_POINT('Ctrl Pts',(27.2838822769084,20.9307107200689,45.9798031387898));
#37538=CARTESIAN_POINT('Ctrl Pts',(31.2751514412539,20.1615884235019,30.9666768060267));
#37539=CARTESIAN_POINT('Ctrl Pts',(25.5920151786696,20.0995966052706,14.0168361250147));
#37540=CARTESIAN_POINT('Ctrl Pts',(13.4774764178507,19.862332849719,4.31311612209045));
#37541=CARTESIAN_POINT('Ctrl Pts',(27.1643404540439,20.9641027630587,46.4299850436194));
#37542=CARTESIAN_POINT('Ctrl Pts',(27.2042776484444,20.9564501184246,46.2798535305942));
#37543=CARTESIAN_POINT('Ctrl Pts',(27.244214842845,20.9487974737906,46.129722017569));
#37544=CARTESIAN_POINT('Ctrl Pts',(27.2841520372455,20.9411448291565,45.9795905045439));
#37545=CARTESIAN_POINT('Ctrl Pts',(31.2778714772977,20.1758803657488,30.9664392020272));
#37546=CARTESIAN_POINT('Ctrl Pts',(25.5933449676568,20.1181627721728,14.0165460423503));
#37547=CARTESIAN_POINT('Ctrl Pts',(13.4794429924389,19.8849935193208,4.31240300075057));
#37548=CARTESIAN_POINT('Ctrl Pts',(27.1647329580989,20.9847395112521,46.4295612730399));
#37549=CARTESIAN_POINT('Ctrl Pts',(27.2047191580392,20.9771640232786,46.2794292607107));
#37550=CARTESIAN_POINT('Ctrl Pts',(27.2447053579794,20.9695885353052,46.1292972483814));
#37551=CARTESIAN_POINT('Ctrl Pts',(27.2846915579197,20.9620130473318,45.9791652360522));
#37552=CARTESIAN_POINT('Ctrl Pts',(31.2833115519458,20.2044642499886,30.9659640031278));
#37553=CARTESIAN_POINT('Ctrl Pts',(25.5960045460592,20.1552951062578,14.0159658718316));
#37554=CARTESIAN_POINT('Ctrl Pts',(13.4833761416152,19.9303148585245,4.31097675807076));
#37555=CARTESIAN_POINT('Ctrl Pts',(27.1653217095864,21.0156946339229,46.4289255987532));
#37556=CARTESIAN_POINT('Ctrl Pts',(27.2053814193679,21.0082348808134,46.278792843607));
#37557=CARTESIAN_POINT('Ctrl Pts',(27.2454411291495,21.000775127704,46.1286600884607));
#37558=CARTESIAN_POINT('Ctrl Pts',(27.285500838931,20.9933153745945,45.9785273333144));
#37559=CARTESIAN_POINT('Ctrl Pts',(31.2914718170848,20.2473400636495,30.9652518186868));
#37560=CARTESIAN_POINT('Ctrl Pts',(25.5999939466102,20.2109936225946,14.0150952948138));
#37561=CARTESIAN_POINT('Ctrl Pts',(13.4892758653797,19.9982968673298,4.30883739405111));
#37562=CARTESIAN_POINT('Ctrl Pts',(27.165910455003,21.0466497571015,46.4282899002481));
#37563=CARTESIAN_POINT('Ctrl Pts',(27.2060436766494,21.0393057386868,46.2781564103577));
#37564=CARTESIAN_POINT('Ctrl Pts',(27.2461768982959,21.0319617202721,46.1280229204672));
#37565=CARTESIAN_POINT('Ctrl Pts',(27.2863101199424,21.0246177018574,45.9778894305768));
#37566=CARTESIAN_POINT('Ctrl Pts',(31.2996322845879,20.2902158603888,30.9645404415346));
#37567=CARTESIAN_POINT('Ctrl Pts',(25.6039833885755,20.2666921589687,14.0142242928149));
#37568=CARTESIAN_POINT('Ctrl Pts',(13.4951755891442,20.0662788761352,4.30669803003142));
#37569=CARTESIAN_POINT('Ctrl Pts',(27.1663029488616,21.0672865061488,46.4278660890332));
#37570=CARTESIAN_POINT('Ctrl Pts',(27.2064851794466,21.0600196441101,46.2777321133838));
#37571=CARTESIAN_POINT('Ctrl Pts',(27.2466674100316,21.0527527820714,46.1275981377344));
#37572=CARTESIAN_POINT('Ctrl Pts',(27.2868496406165,21.0454859200326,45.977464162085));
#37573=CARTESIAN_POINT('Ctrl Pts',(31.3050726991135,20.3187997161584,30.9640665971437));
#37574=CARTESIAN_POINT('Ctrl Pts',(25.6066430363201,20.3038245267329,14.0136434086836));
#37575=CARTESIAN_POINT('Ctrl Pts',(13.4991087383205,20.1116002153389,4.30527178735164));
#37576=CARTESIAN_POINT('Ctrl Pts',(27.1664991957514,21.0776048806767,46.4276541832925));
#37577=CARTESIAN_POINT('Ctrl Pts',(27.2067059308188,21.0703765968246,46.277519964808));
#37578=CARTESIAN_POINT('Ctrl Pts',(27.2469126658862,21.0631483129724,46.1273857463236));
#37579=CARTESIAN_POINT('Ctrl Pts',(27.2871194009536,21.0559200291202,45.9772515278391));
#37580=CARTESIAN_POINT('Ctrl Pts',(31.3077929076951,20.3330916439037,30.9638296793928));
#37581=CARTESIAN_POINT('Ctrl Pts',(25.6079728602995,20.3223907107576,14.0133529639299));
#37582=CARTESIAN_POINT('Ctrl Pts',(13.5010753129087,20.1342608849406,4.30455866601175));
#37583=CARTESIAN_POINT('Ctrl Pts',(27.1665181061429,21.0785991614118,46.4276337640108));
#37584=CARTESIAN_POINT('Ctrl Pts',(27.2067272024674,21.0713745949617,46.2774995221267));
#37585=CARTESIAN_POINT('Ctrl Pts',(27.2469362987919,21.0641500285117,46.1273652802426));
#37586=CARTESIAN_POINT('Ctrl Pts',(27.2871453951164,21.0569254620617,45.9772310383585));
#37587=CARTESIAN_POINT('Ctrl Pts',(31.308055027565,20.3344688170607,30.9638068499487));
#37588=CARTESIAN_POINT('Ctrl Pts',(25.6081010024172,20.3241797521467,14.0133249766125));
#37589=CARTESIAN_POINT('Ctrl Pts',(13.5012648124487,20.1364444718193,4.30448994948977));
#37590=CARTESIAN_POINT('Ctrl Pts',(27.1665370165344,21.0795934421468,46.4276133447292));
#37591=CARTESIAN_POINT('Ctrl Pts',(27.2067484741159,21.0723725930989,46.2774790794455));
#37592=CARTESIAN_POINT('Ctrl Pts',(27.2469599316975,21.0651517440511,46.1273448141617));
#37593=CARTESIAN_POINT('Ctrl Pts',(27.287171389279,21.0579308950032,45.977210548878));
#37594=CARTESIAN_POINT('Ctrl Pts',(31.3083171474348,20.3358459902176,30.9637840205045));
#37595=CARTESIAN_POINT('Ctrl Pts',(25.608229144535,20.3259687935359,14.0132969892951));
#37596=CARTESIAN_POINT('Ctrl Pts',(13.5014543119888,20.1386280586979,4.3044212329678));
#37597=CARTESIAN_POINT('Ctrl Pts',(27.1665559269259,21.0805877228818,46.4275929254476));
#37598=CARTESIAN_POINT('Ctrl Pts',(27.2067697457645,21.0733705912361,46.2774586367642));
#37599=CARTESIAN_POINT('Ctrl Pts',(27.2469835646031,21.0661534595904,46.1273243480808));
#37600=CARTESIAN_POINT('Ctrl Pts',(27.2871973834418,21.0589363279447,45.9771900593974));
#37601=CARTESIAN_POINT('Ctrl Pts',(31.3085792673046,20.3372231633746,30.9637611910603));
#37602=CARTESIAN_POINT('Ctrl Pts',(25.6083572866527,20.327757834925,14.0132690019777));
#37603=CARTESIAN_POINT('Ctrl Pts',(13.5016438115288,20.1408116455766,4.30435251644582));
#37604=CARTESIAN_POINT('',(28.5350439006909,20.5529756002067,37.188944948637));
#37605=CARTESIAN_POINT('Origin',(7.5111559719605E-6,20.2903503023534,4.07573877568452E-6));
#37606=CARTESIAN_POINT('Origin',(7.5111559719605E-6,-3.14714969764662,4.07573877568452E-6));
#37607=CARTESIAN_POINT('Origin',(7.5111559719605E-6,21.2397676607012,4.07573877568452E-6));
#37608=CARTESIAN_POINT('Origin',(7.5111559719605E-6,21.2397676607012,4.07573877568452E-6));
#37609=CARTESIAN_POINT('Origin',(7.5111559719605E-6,21.2397676607012,4.07573877568452E-6));
#37610=CARTESIAN_POINT('Origin',(7.5111559719605E-6,21.2397676607012,4.07573877568452E-6));
#37611=CARTESIAN_POINT('Origin',(7.5111559719605E-6,21.2397676607012,4.07573877568452E-6));
#37612=CARTESIAN_POINT('Origin',(7.5111559719605E-6,21.2397676607012,4.07573877568452E-6));
#37613=CARTESIAN_POINT('Origin',(7.5111559719605E-6,15.6028503023534,4.07573877568452E-6));
#37614=CARTESIAN_POINT('Origin',(7.5111559719605E-6,13.1028503023534,4.07573877568452E-6));
#37615=CARTESIAN_POINT('Origin',(7.5111559719605E-6,15.6028503023534,4.07573877568452E-6));
#37620=UNCERTAINTY_MEASURE_WITH_UNIT(LENGTH_MEASURE(0.01),#37626,
'DISTANCE_ACCURACY_VALUE',
'Maximum model space distance between geometric entities at asserted c
onnectivities');
#37621=UNCERTAINTY_MEASURE_WITH_UNIT(LENGTH_MEASURE(0.01),#37626,
'DISTANCE_ACCURACY_VALUE',
'Maximum model space distance between geometric entities at asserted c
onnectivities');
#37624=(
GEOMETRIC_REPRESENTATION_CONTEXT(3)
GLOBAL_UNCERTAINTY_ASSIGNED_CONTEXT((#37620))
GLOBAL_UNIT_ASSIGNED_CONTEXT((#37626,#37628,#37629))
REPRESENTATION_CONTEXT('','3D')
);
#37625=(
GEOMETRIC_REPRESENTATION_CONTEXT(3)
GLOBAL_UNCERTAINTY_ASSIGNED_CONTEXT((#37621))
GLOBAL_UNIT_ASSIGNED_CONTEXT((#37626,#37628,#37629))
REPRESENTATION_CONTEXT('','3D')
);
#37626=(
LENGTH_UNIT()
NAMED_UNIT(*)
SI_UNIT(.MILLI.,.METRE.)
);
#37628=(
NAMED_UNIT(*)
PLANE_ANGLE_UNIT()
SI_UNIT($,.RADIAN.)
);
#37629=(
NAMED_UNIT(*)
SI_UNIT($,.STERADIAN.)
SOLID_ANGLE_UNIT()
);
#37632=SHAPE_DEFINITION_REPRESENTATION(#37635,#37640);
#37635=PRODUCT_DEFINITION_SHAPE('',$,#37644);
#37640=SHAPE_REPRESENTATION('',(#12950),#37624);
#37641=PRODUCT_DEFINITION_CONTEXT('part definition',#37652,'design');
#37644=PRODUCT_DEFINITION('Part 2 - Fan','Part 2 - Fan',#37647,#37641);
#37647=PRODUCT_DEFINITION_FORMATION('',$,#37656);
#37652=APPLICATION_CONTEXT(
'Core Data for Automotive Mechanical Design Process');
#37653=PRODUCT_CONTEXT('part definition',#37652,'mechanical');
#37656=PRODUCT('Part 2 - Fan','Part 2 - Fan',$,(#37653));
#37659=PRESENTATION_STYLE_ASSIGNMENT((#37662));
#37662=SURFACE_STYLE_USAGE(.BOTH.,#37665);
#37665=SURFACE_SIDE_STYLE('',(#37668));
#37668=SURFACE_STYLE_FILL_AREA(#37671);
#37671=FILL_AREA_STYLE('Opaque(61,176,222)',(#37674));
#37674=FILL_AREA_STYLE_COLOUR('Opaque(61,176,222)',#37677);
#37677=COLOUR_RGB('Opaque(61,176,222)',0.23921568627451,0.690196078431373,
0.870588235294118);
ENDSEC;
END-ISO-10303-21;
